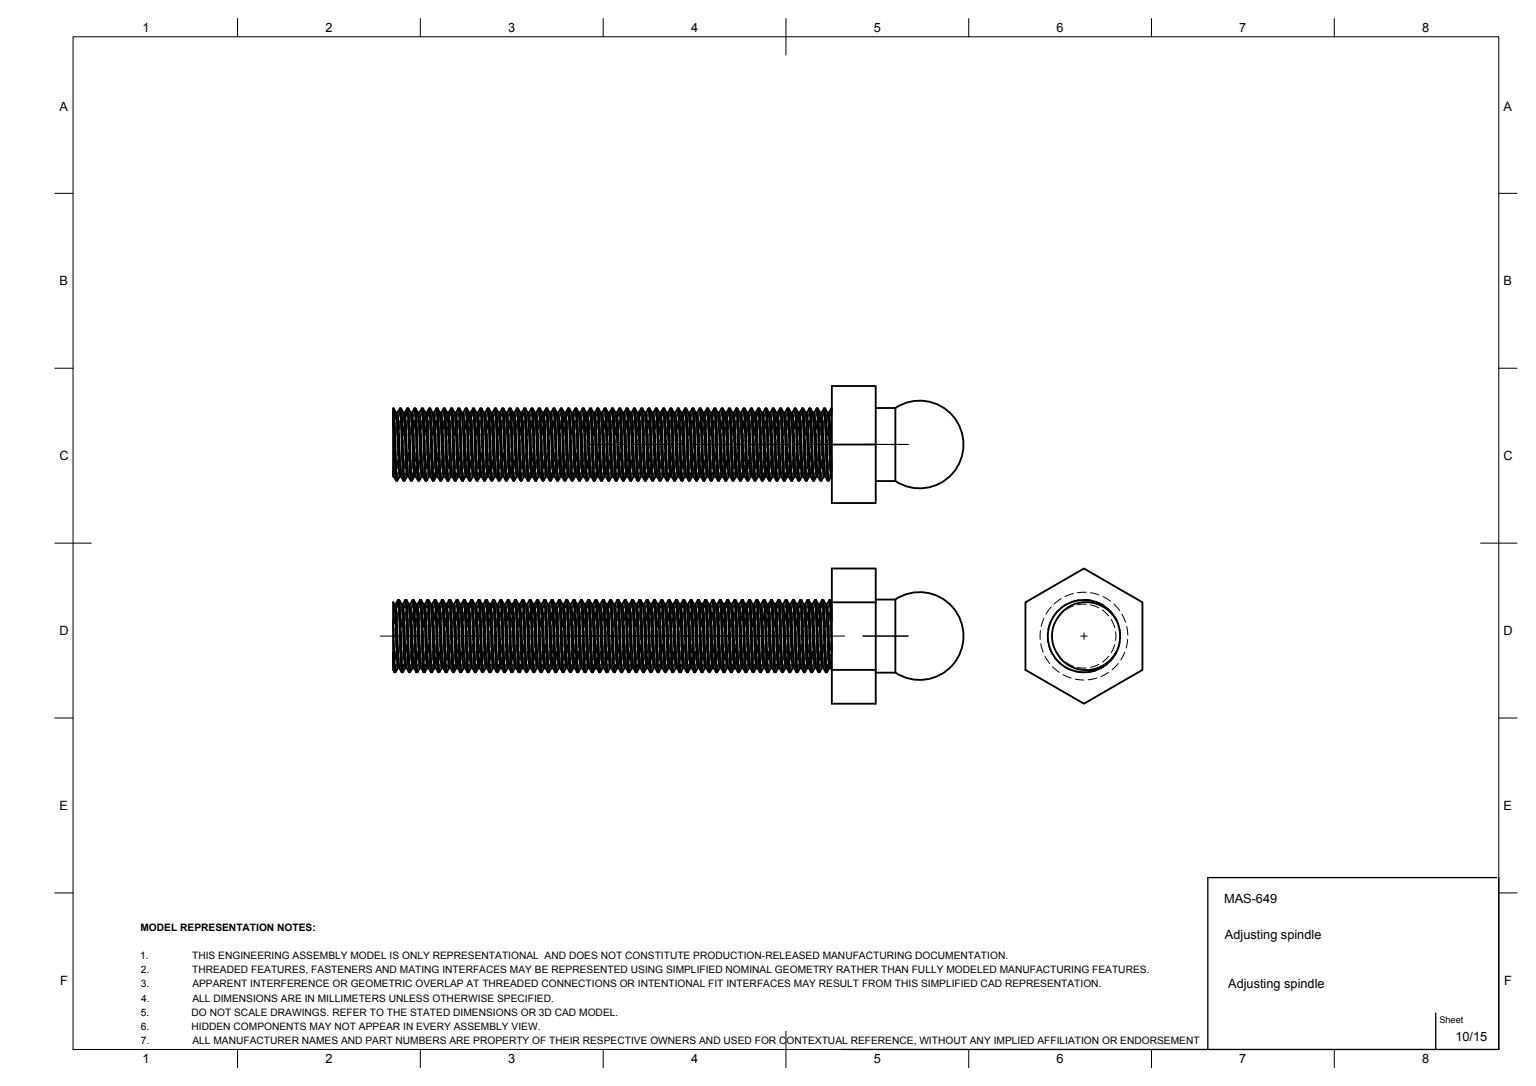
ISO-10303-21;
HEADER;
/* Generated by software containing ST-Developer
 * from STEP Tools, Inc. (www.steptools.com) 
 */

FILE_DESCRIPTION(
/* description */ ('Independent equipment support assembly with bolted 600 x 500 mm welde
d perimeter frame, four adjustable legs and swivel feet. Nominal overa
ll height 518 mm. No load rating assigned.'),
/* implementation_level */ '2;1');

FILE_NAME(
/* name */ 'Adjusting spindle.step',
/* time_stamp */ '2026-11-07T17:30:39-08:00',
/* author */ (''),
/* organization */ (''),
/* preprocessor_version */ 'ST-DEVELOPER v20.2',
/* originating_system */ 'Autodesk Translation Framework v15.17.0.0',
/* authorisation */ '');

FILE_SCHEMA (('AUTOMOTIVE_DESIGN { 1 0 10303 214 3 1 1 }'));
ENDSEC;

DATA;
#10=MECHANICAL_DESIGN_GEOMETRIC_PRESENTATION_REPRESENTATION('',(#2219),#63755);
#13=SPHERICAL_SURFACE('',#15392,6.);
#279=B_SPLINE_SURFACE_WITH_KNOTS('',3,3,((#55973,#55974,#55975,#55976,#55977,
#55978,#55979,#55980,#55981,#55982,#55983,#55984,#55985,#55986,#55987,#55988,
#55989,#55990,#55991,#55992,#55993,#55994,#55995,#55996,#55997,#55998,#55999,
#56000,#56001,#56002,#56003,#56004,#56005,#56006,#56007,#56008,#56009,#56010,
#56011,#56012,#56013,#56014,#56015,#56016,#56017,#56018,#56019,#56020,#56021,
#56022,#56023,#56024,#56025,#56026,#56027,#56028,#56029,#56030,#56031,#56032,
#56033,#56034,#56035,#56036,#56037,#56038,#56039,#56040,#56041,#56042,#56043,
#56044,#56045,#56046,#56047,#56048,#56049,#56050,#56051,#56052,#56053,#56054,
#56055,#56056,#56057,#56058,#56059,#56060,#56061,#56062,#56063,#56064,#56065,
#56066,#56067,#56068,#56069,#56070,#56071,#56072,#56073,#56074,#56075,#56076,
#56077,#56078,#56079,#56080,#56081,#56082,#56083,#56084,#56085,#56086,#56087,
#56088,#56089,#56090,#56091,#56092,#56093,#56094,#56095,#56096,#56097,#56098,
#56099,#56100,#56101,#56102,#56103,#56104,#56105,#56106,#56107,#56108,#56109,
#56110,#56111,#56112,#56113,#56114,#56115,#56116,#56117,#56118,#56119,#56120,
#56121,#56122,#56123,#56124,#56125,#56126,#56127,#56128,#56129,#56130,#56131,
#56132,#56133,#56134,#56135,#56136,#56137,#56138,#56139,#56140,#56141,#56142,
#56143,#56144,#56145,#56146,#56147,#56148,#56149,#56150,#56151,#56152,#56153,
#56154,#56155,#56156,#56157,#56158,#56159,#56160,#56161,#56162,#56163,#56164,
#56165,#56166,#56167,#56168,#56169,#56170,#56171,#56172,#56173,#56174,#56175,
#56176,#56177,#56178,#56179,#56180,#56181,#56182,#56183,#56184,#56185,#56186,
#56187,#56188,#56189,#56190,#56191,#56192,#56193,#56194,#56195,#56196,#56197,
#56198,#56199,#56200,#56201,#56202,#56203,#56204,#56205,#56206,#56207,#56208,
#56209,#56210,#56211,#56212,#56213,#56214,#56215,#56216,#56217,#56218,#56219,
#56220,#56221,#56222,#56223,#56224,#56225,#56226,#56227,#56228,#56229,#56230,
#56231,#56232,#56233,#56234,#56235,#56236,#56237,#56238,#56239,#56240,#56241,
#56242,#56243,#56244,#56245,#56246,#56247,#56248,#56249,#56250,#56251,#56252,
#56253,#56254,#56255,#56256,#56257,#56258,#56259,#56260,#56261,#56262,#56263,
#56264,#56265,#56266,#56267,#56268,#56269,#56270,#56271,#56272,#56273,#56274,
#56275,#56276,#56277,#56278,#56279,#56280,#56281,#56282,#56283,#56284,#56285,
#56286,#56287,#56288,#56289,#56290,#56291,#56292,#56293,#56294,#56295,#56296,
#56297,#56298,#56299,#56300,#56301,#56302,#56303,#56304,#56305,#56306,#56307,
#56308,#56309,#56310,#56311,#56312,#56313,#56314,#56315,#56316,#56317,#56318,
#56319,#56320,#56321,#56322,#56323,#56324,#56325,#56326,#56327,#56328,#56329,
#56330,#56331,#56332,#56333,#56334,#56335,#56336,#56337,#56338,#56339,#56340,
#56341,#56342,#56343,#56344,#56345,#56346,#56347,#56348,#56349,#56350,#56351,
#56352,#56353,#56354,#56355,#56356,#56357),(#56358,#56359,#56360,#56361,
#56362,#56363,#56364,#56365,#56366,#56367,#56368,#56369,#56370,#56371,#56372,
#56373,#56374,#56375,#56376,#56377,#56378,#56379,#56380,#56381,#56382,#56383,
#56384,#56385,#56386,#56387,#56388,#56389,#56390,#56391,#56392,#56393,#56394,
#56395,#56396,#56397,#56398,#56399,#56400,#56401,#56402,#56403,#56404,#56405,
#56406,#56407,#56408,#56409,#56410,#56411,#56412,#56413,#56414,#56415,#56416,
#56417,#56418,#56419,#56420,#56421,#56422,#56423,#56424,#56425,#56426,#56427,
#56428,#56429,#56430,#56431,#56432,#56433,#56434,#56435,#56436,#56437,#56438,
#56439,#56440,#56441,#56442,#56443,#56444,#56445,#56446,#56447,#56448,#56449,
#56450,#56451,#56452,#56453,#56454,#56455,#56456,#56457,#56458,#56459,#56460,
#56461,#56462,#56463,#56464,#56465,#56466,#56467,#56468,#56469,#56470,#56471,
#56472,#56473,#56474,#56475,#56476,#56477,#56478,#56479,#56480,#56481,#56482,
#56483,#56484,#56485,#56486,#56487,#56488,#56489,#56490,#56491,#56492,#56493,
#56494,#56495,#56496,#56497,#56498,#56499,#56500,#56501,#56502,#56503,#56504,
#56505,#56506,#56507,#56508,#56509,#56510,#56511,#56512,#56513,#56514,#56515,
#56516,#56517,#56518,#56519,#56520,#56521,#56522,#56523,#56524,#56525,#56526,
#56527,#56528,#56529,#56530,#56531,#56532,#56533,#56534,#56535,#56536,#56537,
#56538,#56539,#56540,#56541,#56542,#56543,#56544,#56545,#56546,#56547,#56548,
#56549,#56550,#56551,#56552,#56553,#56554,#56555,#56556,#56557,#56558,#56559,
#56560,#56561,#56562,#56563,#56564,#56565,#56566,#56567,#56568,#56569,#56570,
#56571,#56572,#56573,#56574,#56575,#56576,#56577,#56578,#56579,#56580,#56581,
#56582,#56583,#56584,#56585,#56586,#56587,#56588,#56589,#56590,#56591,#56592,
#56593,#56594,#56595,#56596,#56597,#56598,#56599,#56600,#56601,#56602,#56603,
#56604,#56605,#56606,#56607,#56608,#56609,#56610,#56611,#56612,#56613,#56614,
#56615,#56616,#56617,#56618,#56619,#56620,#56621,#56622,#56623,#56624,#56625,
#56626,#56627,#56628,#56629,#56630,#56631,#56632,#56633,#56634,#56635,#56636,
#56637,#56638,#56639,#56640,#56641,#56642,#56643,#56644,#56645,#56646,#56647,
#56648,#56649,#56650,#56651,#56652,#56653,#56654,#56655,#56656,#56657,#56658,
#56659,#56660,#56661,#56662,#56663,#56664,#56665,#56666,#56667,#56668,#56669,
#56670,#56671,#56672,#56673,#56674,#56675,#56676,#56677,#56678,#56679,#56680,
#56681,#56682,#56683,#56684,#56685,#56686,#56687,#56688,#56689,#56690,#56691,
#56692,#56693,#56694,#56695,#56696,#56697,#56698,#56699,#56700,#56701,#56702,
#56703,#56704,#56705,#56706,#56707,#56708,#56709,#56710,#56711,#56712,#56713,
#56714,#56715,#56716,#56717,#56718,#56719,#56720,#56721,#56722,#56723,#56724,
#56725,#56726,#56727,#56728,#56729,#56730,#56731,#56732,#56733,#56734,#56735,
#56736,#56737,#56738,#56739,#56740,#56741,#56742),(#56743,#56744,#56745,
#56746,#56747,#56748,#56749,#56750,#56751,#56752,#56753,#56754,#56755,#56756,
#56757,#56758,#56759,#56760,#56761,#56762,#56763,#56764,#56765,#56766,#56767,
#56768,#56769,#56770,#56771,#56772,#56773,#56774,#56775,#56776,#56777,#56778,
#56779,#56780,#56781,#56782,#56783,#56784,#56785,#56786,#56787,#56788,#56789,
#56790,#56791,#56792,#56793,#56794,#56795,#56796,#56797,#56798,#56799,#56800,
#56801,#56802,#56803,#56804,#56805,#56806,#56807,#56808,#56809,#56810,#56811,
#56812,#56813,#56814,#56815,#56816,#56817,#56818,#56819,#56820,#56821,#56822,
#56823,#56824,#56825,#56826,#56827,#56828,#56829,#56830,#56831,#56832,#56833,
#56834,#56835,#56836,#56837,#56838,#56839,#56840,#56841,#56842,#56843,#56844,
#56845,#56846,#56847,#56848,#56849,#56850,#56851,#56852,#56853,#56854,#56855,
#56856,#56857,#56858,#56859,#56860,#56861,#56862,#56863,#56864,#56865,#56866,
#56867,#56868,#56869,#56870,#56871,#56872,#56873,#56874,#56875,#56876,#56877,
#56878,#56879,#56880,#56881,#56882,#56883,#56884,#56885,#56886,#56887,#56888,
#56889,#56890,#56891,#56892,#56893,#56894,#56895,#56896,#56897,#56898,#56899,
#56900,#56901,#56902,#56903,#56904,#56905,#56906,#56907,#56908,#56909,#56910,
#56911,#56912,#56913,#56914,#56915,#56916,#56917,#56918,#56919,#56920,#56921,
#56922,#56923,#56924,#56925,#56926,#56927,#56928,#56929,#56930,#56931,#56932,
#56933,#56934,#56935,#56936,#56937,#56938,#56939,#56940,#56941,#56942,#56943,
#56944,#56945,#56946,#56947,#56948,#56949,#56950,#56951,#56952,#56953,#56954,
#56955,#56956,#56957,#56958,#56959,#56960,#56961,#56962,#56963,#56964,#56965,
#56966,#56967,#56968,#56969,#56970,#56971,#56972,#56973,#56974,#56975,#56976,
#56977,#56978,#56979,#56980,#56981,#56982,#56983,#56984,#56985,#56986,#56987,
#56988,#56989,#56990,#56991,#56992,#56993,#56994,#56995,#56996,#56997,#56998,
#56999,#57000,#57001,#57002,#57003,#57004,#57005,#57006,#57007,#57008,#57009,
#57010,#57011,#57012,#57013,#57014,#57015,#57016,#57017,#57018,#57019,#57020,
#57021,#57022,#57023,#57024,#57025,#57026,#57027,#57028,#57029,#57030,#57031,
#57032,#57033,#57034,#57035,#57036,#57037,#57038,#57039,#57040,#57041,#57042,
#57043,#57044,#57045,#57046,#57047,#57048,#57049,#57050,#57051,#57052,#57053,
#57054,#57055,#57056,#57057,#57058,#57059,#57060,#57061,#57062,#57063,#57064,
#57065,#57066,#57067,#57068,#57069,#57070,#57071,#57072,#57073,#57074,#57075,
#57076,#57077,#57078,#57079,#57080,#57081,#57082,#57083,#57084,#57085,#57086,
#57087,#57088,#57089,#57090,#57091,#57092,#57093,#57094,#57095,#57096,#57097,
#57098,#57099,#57100,#57101,#57102,#57103,#57104,#57105,#57106,#57107,#57108,
#57109,#57110,#57111,#57112,#57113,#57114,#57115,#57116,#57117,#57118,#57119,
#57120,#57121,#57122,#57123,#57124,#57125,#57126,#57127),(#57128,#57129,
#57130,#57131,#57132,#57133,#57134,#57135,#57136,#57137,#57138,#57139,#57140,
#57141,#57142,#57143,#57144,#57145,#57146,#57147,#57148,#57149,#57150,#57151,
#57152,#57153,#57154,#57155,#57156,#57157,#57158,#57159,#57160,#57161,#57162,
#57163,#57164,#57165,#57166,#57167,#57168,#57169,#57170,#57171,#57172,#57173,
#57174,#57175,#57176,#57177,#57178,#57179,#57180,#57181,#57182,#57183,#57184,
#57185,#57186,#57187,#57188,#57189,#57190,#57191,#57192,#57193,#57194,#57195,
#57196,#57197,#57198,#57199,#57200,#57201,#57202,#57203,#57204,#57205,#57206,
#57207,#57208,#57209,#57210,#57211,#57212,#57213,#57214,#57215,#57216,#57217,
#57218,#57219,#57220,#57221,#57222,#57223,#57224,#57225,#57226,#57227,#57228,
#57229,#57230,#57231,#57232,#57233,#57234,#57235,#57236,#57237,#57238,#57239,
#57240,#57241,#57242,#57243,#57244,#57245,#57246,#57247,#57248,#57249,#57250,
#57251,#57252,#57253,#57254,#57255,#57256,#57257,#57258,#57259,#57260,#57261,
#57262,#57263,#57264,#57265,#57266,#57267,#57268,#57269,#57270,#57271,#57272,
#57273,#57274,#57275,#57276,#57277,#57278,#57279,#57280,#57281,#57282,#57283,
#57284,#57285,#57286,#57287,#57288,#57289,#57290,#57291,#57292,#57293,#57294,
#57295,#57296,#57297,#57298,#57299,#57300,#57301,#57302,#57303,#57304,#57305,
#57306,#57307,#57308,#57309,#57310,#57311,#57312,#57313,#57314,#57315,#57316,
#57317,#57318,#57319,#57320,#57321,#57322,#57323,#57324,#57325,#57326,#57327,
#57328,#57329,#57330,#57331,#57332,#57333,#57334,#57335,#57336,#57337,#57338,
#57339,#57340,#57341,#57342,#57343,#57344,#57345,#57346,#57347,#57348,#57349,
#57350,#57351,#57352,#57353,#57354,#57355,#57356,#57357,#57358,#57359,#57360,
#57361,#57362,#57363,#57364,#57365,#57366,#57367,#57368,#57369,#57370,#57371,
#57372,#57373,#57374,#57375,#57376,#57377,#57378,#57379,#57380,#57381,#57382,
#57383,#57384,#57385,#57386,#57387,#57388,#57389,#57390,#57391,#57392,#57393,
#57394,#57395,#57396,#57397,#57398,#57399,#57400,#57401,#57402,#57403,#57404,
#57405,#57406,#57407,#57408,#57409,#57410,#57411,#57412,#57413,#57414,#57415,
#57416,#57417,#57418,#57419,#57420,#57421,#57422,#57423,#57424,#57425,#57426,
#57427,#57428,#57429,#57430,#57431,#57432,#57433,#57434,#57435,#57436,#57437,
#57438,#57439,#57440,#57441,#57442,#57443,#57444,#57445,#57446,#57447,#57448,
#57449,#57450,#57451,#57452,#57453,#57454,#57455,#57456,#57457,#57458,#57459,
#57460,#57461,#57462,#57463,#57464,#57465,#57466,#57467,#57468,#57469,#57470,
#57471,#57472,#57473,#57474,#57475,#57476,#57477,#57478,#57479,#57480,#57481,
#57482,#57483,#57484,#57485,#57486,#57487,#57488,#57489,#57490,#57491,#57492,
#57493,#57494,#57495,#57496,#57497,#57498,#57499,#57500,#57501,#57502,#57503,
#57504,#57505,#57506,#57507,#57508,#57509,#57510,#57511,#57512)),
 .UNSPECIFIED.,.F.,.F.,.F.,(4,4),(4,1,1,1,1,1,1,1,1,1,1,1,1,1,1,1,1,1,1,
1,1,1,1,1,1,1,1,1,1,1,1,1,1,1,1,1,1,1,1,1,1,1,1,1,1,1,1,1,1,1,1,1,1,1,1,
1,1,1,1,1,1,1,1,1,1,1,1,1,1,1,1,1,1,1,1,1,1,1,1,1,1,1,1,1,1,1,1,1,1,1,1,
1,1,1,1,1,1,1,1,1,1,1,1,1,1,1,1,1,1,1,1,1,1,1,1,1,1,1,1,1,1,1,1,1,1,1,1,
1,1,1,1,1,1,1,1,1,1,1,1,1,1,1,1,1,1,1,1,1,1,1,1,1,1,1,1,1,1,1,1,1,1,1,1,
1,1,1,1,1,1,1,1,1,1,1,1,1,1,1,1,1,1,1,1,1,1,1,1,1,1,1,1,1,1,1,1,1,1,1,1,
1,1,1,1,1,1,1,1,1,1,1,1,1,1,1,1,1,1,1,1,1,1,1,1,1,1,1,1,1,1,1,1,1,1,1,1,
1,1,1,1,1,1,1,1,1,1,1,1,1,1,1,1,1,1,1,1,1,1,1,1,1,1,1,1,1,1,1,1,1,1,1,1,
1,1,1,1,1,1,1,1,1,1,1,1,1,1,1,1,1,1,1,1,1,1,1,1,1,1,1,1,1,1,1,1,1,1,1,1,
1,1,1,1,1,1,1,1,1,1,1,1,1,1,1,1,1,1,1,1,1,1,1,1,1,1,1,1,1,1,1,1,1,1,1,1,
1,1,1,1,1,1,1,1,1,1,1,1,1,1,1,1,1,1,1,1,1,1,1,1,1,1,1,1,1,1,1,1,1,1,1,1,
1,1,1,4),(0.,0.0658179306876174),(8.30838445208392,8.80714609643392,9.30590774078392,
10.3034310294839,11.3009543181839,12.2984776068839,13.2960008955839,14.2935241842839,
15.291047472984,16.288570761684,17.286094050384,18.283617339084,19.281140627784,
20.278663916484,21.276187205184,22.273710493884,23.271233782584,24.268757071284,
25.266280359984,26.263803648684,27.261326937384,28.258850226084,29.256373514784,
30.253896803484,31.251420092184,32.2489433808841,33.2464666695841,34.2439899582841,
35.2415132469841,36.2390365356841,37.2365598243841,38.2340831130841,39.2316064017841,
40.2291296904841,41.2266529791841,42.2241762678841,43.2216995565841,44.2192228452841,
45.2167461339841,46.2142694226841,47.2117927113841,48.2093160000841,49.2068392887841,
50.2043625774841,51.2018858661842,52.1994091548842,53.1969324435842,54.1944557322842,
55.1919790209842,56.1895023096842,57.1870255983842,58.1845488870842,59.1820721757842,
60.1795954644842,61.1771187531842,62.1746420418842,63.1721653305842,64.1696886192842,
65.1672119079842,66.1647351966842,67.1622584853842,68.1597817740843,69.1573050627842,
70.1548283514843,71.1523516401843,72.1498749288843,73.1473982175843,74.1449215062843,
75.1424447949843,76.1399680836843,77.1374913723843,78.1350146610843,79.1325379497843,
80.1300612384843,81.1275845271843,82.1251078158843,83.1226311045843,84.1201543932843,
85.1176776819843,86.1152009706843,87.1127242593844,88.1102475480844,89.1077708367844,
90.1052941254844,91.1028174141844,92.1003407028844,93.0978639915844,94.0953872802844,
95.0929105689844,96.0904338576844,97.0879571463844,98.0854804350844,99.0830037237844,
100.080527012484,101.078050301184,102.075573589884,103.073096878584,104.070620167284,
105.068143455984,106.065666744684,107.063190033384,108.060713322084,109.058236610784,
110.055759899484,111.053283188184,112.050806476884,113.048329765584,114.045853054284,
115.043376342985,116.040899631685,117.038422920385,118.035946209085,119.033469497785,
120.030992786485,121.028516075185,122.026039363885,123.023562652585,124.021085941285,
125.018609229985,126.016132518685,127.013655807385,128.011179096085,129.008702384785,
130.006225673485,131.003748962185,132.001272250885,132.998795539585,133.996318828285,
134.993842116985,135.991365405685,136.988888694385,137.986411983085,138.983935271785,
139.981458560485,140.978981849185,141.976505137885,142.974028426585,143.971551715285,
144.969075003985,145.966598292685,146.964121581385,147.961644870085,148.959168158785,
149.956691447485,150.954214736185,151.951738024885,152.949261313585,153.946784602285,
154.944307890985,155.941831179685,156.939354468385,157.936877757085,158.934401045785,
159.931924334485,160.929447623185,161.926970911885,162.924494200585,163.922017489285,
164.919540777985,165.917064066685,166.914587355385,167.912110644085,168.909633932785,
169.907157221485,170.904680510185,171.902203798885,172.899727087585,173.897250376285,
174.894773664985,175.892296953685,176.889820242385,177.887343531085,178.884866819785,
179.882390108485,180.879913397185,181.877436685885,182.874959974585,183.872483263285,
184.870006551985,185.867529840685,186.865053129385,187.862576418085,188.860099706785,
189.857622995485,190.855146284185,191.852669572885,192.850192861585,193.847716150285,
194.845239438985,195.842762727685,196.840286016385,197.837809305085,198.835332593785,
199.832855882485,200.830379171185,201.827902459885,202.825425748585,203.822949037285,
204.820472325985,205.817995614685,206.815518903385,207.813042192085,208.810565480785,
209.808088769485,210.805612058185,211.803135346885,212.800658635585,213.798181924285,
214.795705212985,215.793228501685,216.790751790385,217.788275079085,218.785798367785,
219.783321656485,220.780844945185,221.778368233885,222.775891522585,223.773414811285,
224.770938099985,225.768461388685,226.765984677385,227.763507966085,228.761031254785,
229.758554543485,230.756077832185,231.753601120885,232.751124409585,233.748647698285,
234.746170986985,235.743694275685,236.741217564385,237.738740853085,238.736264141785,
239.733787430485,240.731310719185,241.728834007885,242.726357296585,243.723880585285,
244.721403873985,245.718927162685,246.716450451385,247.713973740085,248.711497028785,
249.709020317485,250.706543606185,251.704066894885,252.701590183585,253.699113472285,
254.696636760985,255.694160049685,256.691683338385,257.689206627085,258.686729915785,
259.684253204485,260.681776493185,261.679299781885,262.676823070585,263.674346359285,
264.671869647985,265.669392936685,266.666916225385,267.664439514085,268.661962802785,
269.659486091485,270.657009380185,271.654532668885,272.652055957585,273.649579246285,
274.647102534985,275.644625823685,276.642149112385,277.639672401085,278.637195689785,
279.634718978485,280.632242267185,281.629765555885,282.627288844585,283.624812133285,
284.622335421985,285.619858710685,286.617381999385,287.614905288085,288.612428576785,
289.609951865485,290.607475154186,291.604998442886,292.602521731586,293.600045020286,
294.597568308986,295.595091597686,296.592614886386,297.590138175086,298.587661463786,
299.585184752486,300.582708041186,301.580231329886,302.577754618586,303.575277907286,
304.572801195986,305.570324484686,306.567847773386,307.565371062086,308.562894350786,
309.560417639486,310.557940928186,311.555464216886,312.552987505586,313.550510794286,
314.548034082986,315.545557371686,316.543080660386,317.540603949086,318.538127237786,
319.535650526486,320.533173815186,321.530697103886,322.528220392586,323.525743681286,
324.523266969986,325.520790258686,326.518313547386,327.515836836086,328.513360124786,
329.510883413486,330.508406702186,331.505929990886,332.503453279586,333.500976568286,
334.498499856986,335.496023145686,336.493546434386,337.491069723086,338.488593011786,
339.486116300486,340.483639589186,341.481162877886,342.478686166586,343.476209455286,
344.473732743986,345.471256032686,346.468779321386,347.466302610086,348.463825898786,
349.461349187486,350.458872476186,351.456395764886,352.453919053586,353.451442342286,
354.448965630986,355.446488919686,356.444012208386,357.441535497086,358.439058785786,
359.436582074486,360.434105363186,361.431628651886,362.429151940586,363.426675229286,
364.424198517986,365.421721806686,366.419245095386,367.416768384086,368.414291672786,
369.411814961486,370.409338250186,371.406861538886,372.404384827586,373.401908116286,
374.399431404986,375.396954693686,376.394477982386,377.392001271086,378.389524559786,
379.387047848486,380.384571137186,381.382094425886,382.379617714586,383.377141003286,
384.374664291986,385.372187580686,386.369710869386,386.868472513736,387.367234158086),
 .UNSPECIFIED.);
#280=B_SPLINE_SURFACE_WITH_KNOTS('',3,3,((#57770,#57771,#57772,#57773,#57774,
#57775,#57776,#57777,#57778,#57779,#57780,#57781,#57782,#57783,#57784,#57785,
#57786,#57787,#57788,#57789,#57790,#57791,#57792,#57793,#57794,#57795,#57796,
#57797,#57798,#57799,#57800,#57801,#57802,#57803,#57804,#57805,#57806,#57807,
#57808,#57809,#57810,#57811,#57812,#57813,#57814,#57815,#57816,#57817,#57818,
#57819,#57820,#57821,#57822,#57823,#57824,#57825,#57826,#57827,#57828,#57829,
#57830,#57831,#57832,#57833,#57834,#57835,#57836,#57837,#57838,#57839,#57840,
#57841,#57842,#57843,#57844,#57845,#57846,#57847,#57848,#57849,#57850,#57851,
#57852,#57853,#57854,#57855,#57856,#57857,#57858,#57859,#57860,#57861,#57862,
#57863,#57864,#57865,#57866,#57867,#57868,#57869,#57870,#57871,#57872,#57873,
#57874,#57875,#57876,#57877,#57878,#57879,#57880,#57881,#57882,#57883,#57884,
#57885,#57886,#57887,#57888,#57889,#57890,#57891,#57892,#57893,#57894,#57895,
#57896,#57897,#57898,#57899,#57900,#57901,#57902,#57903,#57904,#57905,#57906,
#57907,#57908,#57909,#57910,#57911,#57912,#57913,#57914,#57915,#57916,#57917,
#57918,#57919,#57920,#57921,#57922,#57923,#57924,#57925,#57926,#57927,#57928,
#57929,#57930,#57931,#57932,#57933,#57934,#57935,#57936,#57937,#57938,#57939,
#57940,#57941,#57942,#57943,#57944,#57945,#57946,#57947,#57948,#57949,#57950,
#57951,#57952,#57953,#57954,#57955,#57956,#57957,#57958,#57959,#57960,#57961,
#57962,#57963,#57964,#57965,#57966,#57967,#57968,#57969,#57970,#57971,#57972,
#57973,#57974,#57975,#57976,#57977,#57978,#57979,#57980,#57981,#57982,#57983,
#57984,#57985,#57986,#57987,#57988,#57989,#57990,#57991,#57992,#57993,#57994,
#57995,#57996,#57997,#57998,#57999,#58000,#58001,#58002,#58003,#58004,#58005,
#58006,#58007,#58008,#58009,#58010,#58011,#58012,#58013,#58014,#58015,#58016,
#58017,#58018,#58019,#58020,#58021,#58022,#58023,#58024,#58025,#58026,#58027,
#58028,#58029,#58030,#58031,#58032,#58033,#58034,#58035,#58036,#58037,#58038,
#58039,#58040,#58041,#58042,#58043,#58044,#58045,#58046,#58047,#58048,#58049,
#58050,#58051,#58052,#58053,#58054,#58055,#58056,#58057,#58058,#58059,#58060,
#58061,#58062,#58063,#58064,#58065,#58066,#58067,#58068,#58069,#58070,#58071,
#58072,#58073,#58074,#58075,#58076,#58077,#58078,#58079,#58080,#58081,#58082,
#58083,#58084,#58085,#58086,#58087,#58088,#58089,#58090,#58091,#58092,#58093,
#58094,#58095,#58096,#58097,#58098,#58099,#58100,#58101,#58102,#58103,#58104,
#58105,#58106,#58107,#58108,#58109,#58110,#58111,#58112,#58113,#58114,#58115,
#58116,#58117,#58118,#58119,#58120,#58121,#58122,#58123,#58124,#58125,#58126,
#58127,#58128,#58129,#58130,#58131,#58132,#58133,#58134,#58135,#58136,#58137,
#58138,#58139,#58140,#58141,#58142,#58143,#58144,#58145,#58146,#58147,#58148,
#58149,#58150,#58151,#58152,#58153,#58154),(#58155,#58156,#58157,#58158,
#58159,#58160,#58161,#58162,#58163,#58164,#58165,#58166,#58167,#58168,#58169,
#58170,#58171,#58172,#58173,#58174,#58175,#58176,#58177,#58178,#58179,#58180,
#58181,#58182,#58183,#58184,#58185,#58186,#58187,#58188,#58189,#58190,#58191,
#58192,#58193,#58194,#58195,#58196,#58197,#58198,#58199,#58200,#58201,#58202,
#58203,#58204,#58205,#58206,#58207,#58208,#58209,#58210,#58211,#58212,#58213,
#58214,#58215,#58216,#58217,#58218,#58219,#58220,#58221,#58222,#58223,#58224,
#58225,#58226,#58227,#58228,#58229,#58230,#58231,#58232,#58233,#58234,#58235,
#58236,#58237,#58238,#58239,#58240,#58241,#58242,#58243,#58244,#58245,#58246,
#58247,#58248,#58249,#58250,#58251,#58252,#58253,#58254,#58255,#58256,#58257,
#58258,#58259,#58260,#58261,#58262,#58263,#58264,#58265,#58266,#58267,#58268,
#58269,#58270,#58271,#58272,#58273,#58274,#58275,#58276,#58277,#58278,#58279,
#58280,#58281,#58282,#58283,#58284,#58285,#58286,#58287,#58288,#58289,#58290,
#58291,#58292,#58293,#58294,#58295,#58296,#58297,#58298,#58299,#58300,#58301,
#58302,#58303,#58304,#58305,#58306,#58307,#58308,#58309,#58310,#58311,#58312,
#58313,#58314,#58315,#58316,#58317,#58318,#58319,#58320,#58321,#58322,#58323,
#58324,#58325,#58326,#58327,#58328,#58329,#58330,#58331,#58332,#58333,#58334,
#58335,#58336,#58337,#58338,#58339,#58340,#58341,#58342,#58343,#58344,#58345,
#58346,#58347,#58348,#58349,#58350,#58351,#58352,#58353,#58354,#58355,#58356,
#58357,#58358,#58359,#58360,#58361,#58362,#58363,#58364,#58365,#58366,#58367,
#58368,#58369,#58370,#58371,#58372,#58373,#58374,#58375,#58376,#58377,#58378,
#58379,#58380,#58381,#58382,#58383,#58384,#58385,#58386,#58387,#58388,#58389,
#58390,#58391,#58392,#58393,#58394,#58395,#58396,#58397,#58398,#58399,#58400,
#58401,#58402,#58403,#58404,#58405,#58406,#58407,#58408,#58409,#58410,#58411,
#58412,#58413,#58414,#58415,#58416,#58417,#58418,#58419,#58420,#58421,#58422,
#58423,#58424,#58425,#58426,#58427,#58428,#58429,#58430,#58431,#58432,#58433,
#58434,#58435,#58436,#58437,#58438,#58439,#58440,#58441,#58442,#58443,#58444,
#58445,#58446,#58447,#58448,#58449,#58450,#58451,#58452,#58453,#58454,#58455,
#58456,#58457,#58458,#58459,#58460,#58461,#58462,#58463,#58464,#58465,#58466,
#58467,#58468,#58469,#58470,#58471,#58472,#58473,#58474,#58475,#58476,#58477,
#58478,#58479,#58480,#58481,#58482,#58483,#58484,#58485,#58486,#58487,#58488,
#58489,#58490,#58491,#58492,#58493,#58494,#58495,#58496,#58497,#58498,#58499,
#58500,#58501,#58502,#58503,#58504,#58505,#58506,#58507,#58508,#58509,#58510,
#58511,#58512,#58513,#58514,#58515,#58516,#58517,#58518,#58519,#58520,#58521,
#58522,#58523,#58524,#58525,#58526,#58527,#58528,#58529,#58530,#58531,#58532,
#58533,#58534,#58535,#58536,#58537,#58538,#58539),(#58540,#58541,#58542,
#58543,#58544,#58545,#58546,#58547,#58548,#58549,#58550,#58551,#58552,#58553,
#58554,#58555,#58556,#58557,#58558,#58559,#58560,#58561,#58562,#58563,#58564,
#58565,#58566,#58567,#58568,#58569,#58570,#58571,#58572,#58573,#58574,#58575,
#58576,#58577,#58578,#58579,#58580,#58581,#58582,#58583,#58584,#58585,#58586,
#58587,#58588,#58589,#58590,#58591,#58592,#58593,#58594,#58595,#58596,#58597,
#58598,#58599,#58600,#58601,#58602,#58603,#58604,#58605,#58606,#58607,#58608,
#58609,#58610,#58611,#58612,#58613,#58614,#58615,#58616,#58617,#58618,#58619,
#58620,#58621,#58622,#58623,#58624,#58625,#58626,#58627,#58628,#58629,#58630,
#58631,#58632,#58633,#58634,#58635,#58636,#58637,#58638,#58639,#58640,#58641,
#58642,#58643,#58644,#58645,#58646,#58647,#58648,#58649,#58650,#58651,#58652,
#58653,#58654,#58655,#58656,#58657,#58658,#58659,#58660,#58661,#58662,#58663,
#58664,#58665,#58666,#58667,#58668,#58669,#58670,#58671,#58672,#58673,#58674,
#58675,#58676,#58677,#58678,#58679,#58680,#58681,#58682,#58683,#58684,#58685,
#58686,#58687,#58688,#58689,#58690,#58691,#58692,#58693,#58694,#58695,#58696,
#58697,#58698,#58699,#58700,#58701,#58702,#58703,#58704,#58705,#58706,#58707,
#58708,#58709,#58710,#58711,#58712,#58713,#58714,#58715,#58716,#58717,#58718,
#58719,#58720,#58721,#58722,#58723,#58724,#58725,#58726,#58727,#58728,#58729,
#58730,#58731,#58732,#58733,#58734,#58735,#58736,#58737,#58738,#58739,#58740,
#58741,#58742,#58743,#58744,#58745,#58746,#58747,#58748,#58749,#58750,#58751,
#58752,#58753,#58754,#58755,#58756,#58757,#58758,#58759,#58760,#58761,#58762,
#58763,#58764,#58765,#58766,#58767,#58768,#58769,#58770,#58771,#58772,#58773,
#58774,#58775,#58776,#58777,#58778,#58779,#58780,#58781,#58782,#58783,#58784,
#58785,#58786,#58787,#58788,#58789,#58790,#58791,#58792,#58793,#58794,#58795,
#58796,#58797,#58798,#58799,#58800,#58801,#58802,#58803,#58804,#58805,#58806,
#58807,#58808,#58809,#58810,#58811,#58812,#58813,#58814,#58815,#58816,#58817,
#58818,#58819,#58820,#58821,#58822,#58823,#58824,#58825,#58826,#58827,#58828,
#58829,#58830,#58831,#58832,#58833,#58834,#58835,#58836,#58837,#58838,#58839,
#58840,#58841,#58842,#58843,#58844,#58845,#58846,#58847,#58848,#58849,#58850,
#58851,#58852,#58853,#58854,#58855,#58856,#58857,#58858,#58859,#58860,#58861,
#58862,#58863,#58864,#58865,#58866,#58867,#58868,#58869,#58870,#58871,#58872,
#58873,#58874,#58875,#58876,#58877,#58878,#58879,#58880,#58881,#58882,#58883,
#58884,#58885,#58886,#58887,#58888,#58889,#58890,#58891,#58892,#58893,#58894,
#58895,#58896,#58897,#58898,#58899,#58900,#58901,#58902,#58903,#58904,#58905,
#58906,#58907,#58908,#58909,#58910,#58911,#58912,#58913,#58914,#58915,#58916,
#58917,#58918,#58919,#58920,#58921,#58922,#58923,#58924),(#58925,#58926,
#58927,#58928,#58929,#58930,#58931,#58932,#58933,#58934,#58935,#58936,#58937,
#58938,#58939,#58940,#58941,#58942,#58943,#58944,#58945,#58946,#58947,#58948,
#58949,#58950,#58951,#58952,#58953,#58954,#58955,#58956,#58957,#58958,#58959,
#58960,#58961,#58962,#58963,#58964,#58965,#58966,#58967,#58968,#58969,#58970,
#58971,#58972,#58973,#58974,#58975,#58976,#58977,#58978,#58979,#58980,#58981,
#58982,#58983,#58984,#58985,#58986,#58987,#58988,#58989,#58990,#58991,#58992,
#58993,#58994,#58995,#58996,#58997,#58998,#58999,#59000,#59001,#59002,#59003,
#59004,#59005,#59006,#59007,#59008,#59009,#59010,#59011,#59012,#59013,#59014,
#59015,#59016,#59017,#59018,#59019,#59020,#59021,#59022,#59023,#59024,#59025,
#59026,#59027,#59028,#59029,#59030,#59031,#59032,#59033,#59034,#59035,#59036,
#59037,#59038,#59039,#59040,#59041,#59042,#59043,#59044,#59045,#59046,#59047,
#59048,#59049,#59050,#59051,#59052,#59053,#59054,#59055,#59056,#59057,#59058,
#59059,#59060,#59061,#59062,#59063,#59064,#59065,#59066,#59067,#59068,#59069,
#59070,#59071,#59072,#59073,#59074,#59075,#59076,#59077,#59078,#59079,#59080,
#59081,#59082,#59083,#59084,#59085,#59086,#59087,#59088,#59089,#59090,#59091,
#59092,#59093,#59094,#59095,#59096,#59097,#59098,#59099,#59100,#59101,#59102,
#59103,#59104,#59105,#59106,#59107,#59108,#59109,#59110,#59111,#59112,#59113,
#59114,#59115,#59116,#59117,#59118,#59119,#59120,#59121,#59122,#59123,#59124,
#59125,#59126,#59127,#59128,#59129,#59130,#59131,#59132,#59133,#59134,#59135,
#59136,#59137,#59138,#59139,#59140,#59141,#59142,#59143,#59144,#59145,#59146,
#59147,#59148,#59149,#59150,#59151,#59152,#59153,#59154,#59155,#59156,#59157,
#59158,#59159,#59160,#59161,#59162,#59163,#59164,#59165,#59166,#59167,#59168,
#59169,#59170,#59171,#59172,#59173,#59174,#59175,#59176,#59177,#59178,#59179,
#59180,#59181,#59182,#59183,#59184,#59185,#59186,#59187,#59188,#59189,#59190,
#59191,#59192,#59193,#59194,#59195,#59196,#59197,#59198,#59199,#59200,#59201,
#59202,#59203,#59204,#59205,#59206,#59207,#59208,#59209,#59210,#59211,#59212,
#59213,#59214,#59215,#59216,#59217,#59218,#59219,#59220,#59221,#59222,#59223,
#59224,#59225,#59226,#59227,#59228,#59229,#59230,#59231,#59232,#59233,#59234,
#59235,#59236,#59237,#59238,#59239,#59240,#59241,#59242,#59243,#59244,#59245,
#59246,#59247,#59248,#59249,#59250,#59251,#59252,#59253,#59254,#59255,#59256,
#59257,#59258,#59259,#59260,#59261,#59262,#59263,#59264,#59265,#59266,#59267,
#59268,#59269,#59270,#59271,#59272,#59273,#59274,#59275,#59276,#59277,#59278,
#59279,#59280,#59281,#59282,#59283,#59284,#59285,#59286,#59287,#59288,#59289,
#59290,#59291,#59292,#59293,#59294,#59295,#59296,#59297,#59298,#59299,#59300,
#59301,#59302,#59303,#59304,#59305,#59306,#59307,#59308,#59309)),
 .UNSPECIFIED.,.F.,.F.,.F.,(4,4),(4,1,1,1,1,1,1,1,1,1,1,1,1,1,1,1,1,1,1,
1,1,1,1,1,1,1,1,1,1,1,1,1,1,1,1,1,1,1,1,1,1,1,1,1,1,1,1,1,1,1,1,1,1,1,1,
1,1,1,1,1,1,1,1,1,1,1,1,1,1,1,1,1,1,1,1,1,1,1,1,1,1,1,1,1,1,1,1,1,1,1,1,
1,1,1,1,1,1,1,1,1,1,1,1,1,1,1,1,1,1,1,1,1,1,1,1,1,1,1,1,1,1,1,1,1,1,1,1,
1,1,1,1,1,1,1,1,1,1,1,1,1,1,1,1,1,1,1,1,1,1,1,1,1,1,1,1,1,1,1,1,1,1,1,1,
1,1,1,1,1,1,1,1,1,1,1,1,1,1,1,1,1,1,1,1,1,1,1,1,1,1,1,1,1,1,1,1,1,1,1,1,
1,1,1,1,1,1,1,1,1,1,1,1,1,1,1,1,1,1,1,1,1,1,1,1,1,1,1,1,1,1,1,1,1,1,1,1,
1,1,1,1,1,1,1,1,1,1,1,1,1,1,1,1,1,1,1,1,1,1,1,1,1,1,1,1,1,1,1,1,1,1,1,1,
1,1,1,1,1,1,1,1,1,1,1,1,1,1,1,1,1,1,1,1,1,1,1,1,1,1,1,1,1,1,1,1,1,1,1,1,
1,1,1,1,1,1,1,1,1,1,1,1,1,1,1,1,1,1,1,1,1,1,1,1,1,1,1,1,1,1,1,1,1,1,1,1,
1,1,1,1,1,1,1,1,1,1,1,1,1,1,1,1,1,1,1,1,1,1,1,1,1,1,1,1,1,1,1,1,1,1,1,1,
1,1,1,4),(0.,0.0658179306876174),(11.6150328478191,12.1137944921691,12.6125561365191,
13.6100794252191,14.6076027139191,15.6051260026191,16.6026492913191,17.6001725800191,
18.5976958687191,19.5952191574192,20.5927424461192,21.5902657348192,22.5877890235192,
23.5853123122192,24.5828356009192,25.5803588896192,26.5778821783192,27.5754054670192,
28.5729287557192,29.5704520444192,30.5679753331192,31.5654986218192,32.5630219105192,
33.5605451992192,34.5580684879192,35.5555917766192,36.5531150653192,37.5506383540192,
38.5481616427193,39.5456849314193,40.5432082201193,41.5407315088193,42.5382547975193,
43.5357780862193,44.5333013749193,45.5308246636193,46.5283479523193,47.5258712410193,
48.5233945297193,49.5209178184193,50.5184411071193,51.5159643958193,52.5134876845193,
53.5110109732193,54.5085342619193,55.5060575506193,56.5035808393194,57.5011041280194,
58.4986274167194,59.4961507054194,60.4936739941194,61.4911972828194,62.4887205715194,
63.4862438602194,64.4837671489194,65.4812904376194,66.4788137263194,67.4763370150194,
68.4738603037194,69.4713835924194,70.4689068811194,71.4664301698194,72.4639534585194,
73.4614767472195,74.4590000359194,75.4565233246195,76.4540466133195,77.4515699020195,
78.4490931907195,79.4466164794195,80.4441397681195,81.4416630568195,82.4391863455195,
83.4367096342195,84.4342329229195,85.4317562116195,86.4292795003195,87.4268027890195,
88.4243260777195,89.4218493664195,90.4193726551195,91.4168959438195,92.4144192325195,
93.4119425212196,94.4094658099196,95.4069890986196,96.4045123873196,97.4020356760196,
98.3995589647196,99.3970822534196,100.39460554212,101.39212883082,102.38965211952,
103.38717540822,104.38469869692,105.38222198562,106.37974527432,107.37726856302,
108.37479185172,109.37231514042,110.36983842912,111.36736171782,112.36488500652,
113.36240829522,114.35993158392,115.35745487262,116.35497816132,117.35250145002,
118.35002473872,119.34754802742,120.34507131612,121.34259460482,122.34011789352,
123.33764118222,124.33516447092,125.33268775962,126.33021104832,127.32773433702,
128.32525762572,129.32278091442,130.32030420312,131.31782749182,132.31535078052,
133.31287406922,134.31039735792,135.30792064662,136.30544393532,137.30296722402,
138.30049051272,139.29801380142,140.29553709012,141.29306037882,142.29058366752,
143.28810695622,144.28563024492,145.28315353362,146.28067682232,147.27820011102,
148.27572339972,149.27324668842,150.27076997712,151.26829326582,152.26581655452,
153.26333984322,154.26086313192,155.25838642062,156.25590970932,157.25343299802,
158.25095628672,159.24847957542,160.24600286412,161.24352615282,162.24104944152,
163.23857273022,164.23609601892,165.23361930762,166.23114259632,167.22866588502,
168.22618917372,169.22371246242,170.22123575112,171.21875903982,172.21628232852,
173.21380561722,174.21132890592,175.20885219462,176.20637548332,177.20389877202,
178.20142206072,179.19894534942,180.19646863812,181.19399192682,182.19151521552,
183.18903850422,184.18656179292,185.18408508162,186.18160837032,187.17913165902,
188.17665494772,189.17417823642,190.17170152512,191.16922481382,192.16674810252,
193.16427139122,194.16179467992,195.15931796862,196.15684125732,197.15436454602,
198.15188783472,199.14941112342,200.14693441212,201.14445770082,202.14198098952,
203.13950427822,204.13702756692,205.13455085562,206.13207414432,207.12959743302,
208.12712072172,209.12464401042,210.12216729912,211.11969058782,212.11721387652,
213.11473716522,214.11226045392,215.10978374262,216.10730703132,217.10483032002,
218.10235360872,219.09987689742,220.09740018612,221.09492347482,222.09244676352,
223.08997005222,224.08749334092,225.08501662962,226.08253991832,227.08006320702,
228.07758649572,229.07510978442,230.07263307312,231.07015636182,232.06767965052,
233.06520293922,234.06272622792,235.06024951662,236.05777280532,237.05529609402,
238.05281938272,239.05034267142,240.04786596012,241.04538924882,242.04291253752,
243.04043582622,244.03795911492,245.03548240362,246.03300569232,247.03052898102,
248.02805226972,249.02557555842,250.02309884712,251.02062213582,252.01814542452,
253.01566871322,254.01319200192,255.01071529062,256.00823857932,257.00576186802,
258.00328515672,259.00080844542,259.99833173412,260.99585502282,261.99337831152,
262.99090160022,263.98842488892,264.98594817762,265.983471466321,266.980994755021,
267.97851804372,268.97604133242,269.973564621121,270.971087909821,271.968611198521,
272.966134487221,273.963657775921,274.961181064621,275.958704353321,276.956227642021,
277.953750930721,278.951274219421,279.948797508121,280.946320796821,281.943844085521,
282.941367374221,283.938890662921,284.936413951621,285.933937240321,286.931460529021,
287.928983817721,288.926507106421,289.924030395121,290.921553683821,291.919076972521,
292.916600261221,293.914123549921,294.911646838621,295.909170127321,296.906693416021,
297.904216704721,298.901739993421,299.899263282121,300.896786570821,301.894309859521,
302.891833148221,303.889356436921,304.886879725621,305.884403014321,306.881926303021,
307.879449591721,308.876972880421,309.874496169121,310.872019457821,311.869542746521,
312.867066035221,313.864589323921,314.862112612621,315.859635901321,316.857159190021,
317.854682478721,318.852205767421,319.849729056121,320.847252344821,321.844775633521,
322.842298922221,323.839822210921,324.837345499621,325.834868788321,326.832392077021,
327.829915365721,328.827438654421,329.824961943121,330.822485231821,331.820008520521,
332.817531809221,333.815055097921,334.812578386621,335.810101675321,336.807624964021,
337.805148252721,338.802671541421,339.800194830121,340.797718118821,341.795241407521,
342.792764696221,343.790287984921,344.787811273621,345.785334562321,346.782857851021,
347.780381139721,348.777904428421,349.775427717121,350.772951005821,351.770474294521,
352.767997583221,353.765520871921,354.763044160621,355.760567449321,356.758090738021,
357.755614026721,358.753137315421,359.750660604121,360.748183892821,361.745707181521,
362.743230470221,363.740753758921,364.738277047621,365.735800336321,366.733323625021,
367.730846913721,368.728370202421,369.725893491121,370.723416779821,371.720940068521,
372.718463357221,373.715986645921,374.713509934621,375.711033223321,376.708556512021,
377.706079800721,378.703603089421,379.701126378121,380.698649666821,381.696172955521,
382.693696244221,383.691219532921,384.688742821621,385.686266110321,386.683789399021,
387.681312687721,388.678835976421,389.676359265121,390.175120909471,390.673882553821),
 .UNSPECIFIED.);
#461=CIRCLE('',#15255,4.942);
#462=CIRCLE('',#15316,4.372);
#463=CIRCLE('',#15377,4.372);
#464=CIRCLE('',#15379,4.942);
#465=CIRCLE('',#15382,5.);
#466=CIRCLE('',#15390,5.);
#467=CIRCLE('',#15393,6.);
#1233=B_SPLINE_CURVE_WITH_KNOTS('',3,(#51551,#51552,#51553,#51554,#51555,
#51556,#51557,#51558,#51559,#51560),.UNSPECIFIED.,.F.,.F.,(4,3,3,4),(-4.09293042013064,
-3.99009315480002,-2.99256986610002,-2.06773127522702),.UNSPECIFIED.);
#1234=B_SPLINE_CURVE_WITH_KNOTS('',3,(#51563,#51564,#51565,#51566,#51567,
#51568,#51569,#51570,#51571,#51572),.UNSPECIFIED.,.F.,.F.,(4,3,3,4),(0.,
0.49876164434999,0.997523288699981,1.11639350868703),.UNSPECIFIED.);
#1235=B_SPLINE_CURVE_WITH_KNOTS('',3,(#51577,#51578,#51579,#51580,#51581,
#51582,#51583,#51584,#51585,#51586,#51587,#51588,#51589,#51590,#51591,#51592,
#51593,#51594,#51595,#51596,#51597,#51598),.UNSPECIFIED.,.F.,.F.,(4,3,3,
3,3,3,3,4),(-10.3761157273102,-9.97523288700005,-8.97770959830005,-7.98018630960004,
-6.98266302090004,-5.98513973220003,-4.98761644350003,-4.09293042013064),
 .UNSPECIFIED.);
#1236=B_SPLINE_CURVE_WITH_KNOTS('',3,(#51599,#51600,#51601,#51602,#51603,
#51604,#51605,#51606,#51607,#51608,#51609,#51610,#51611,#51612,#51613,#51614,
#51615,#51616,#51617,#51618,#51619,#51620),.UNSPECIFIED.,.F.,.F.,(4,3,3,
3,3,3,3,4),(1.11639350868703,1.99504657739999,2.9925698661,3.9900931548,
4.98761644350001,5.98513973220002,6.98266302090003,7.39957881586659),
 .UNSPECIFIED.);
#1237=B_SPLINE_CURVE_WITH_KNOTS('',3,(#51625,#51626,#51627,#51628,#51629,
#51630,#51631,#51632,#51633,#51634,#51635,#51636,#51637,#51638,#51639,#51640,
#51641,#51642,#51643,#51644,#51645,#51646),.UNSPECIFIED.,.F.,.F.,(4,3,3,
3,3,3,3,4),(-16.6593010344898,-15.9603726192001,-14.9628493305001,-13.9653260418001,
-12.9678027531001,-11.9702794644001,-10.9727561757001,-10.3761157273102),
 .UNSPECIFIED.);
#1238=B_SPLINE_CURVE_WITH_KNOTS('',3,(#51647,#51648,#51649,#51650,#51651,
#51652,#51653,#51654,#51655,#51656,#51657,#51658,#51659,#51660,#51661,#51662,
#51663,#51664,#51665,#51666,#51667,#51668),.UNSPECIFIED.,.F.,.F.,(4,3,3,
3,3,3,3,4),(7.39957881586659,7.98018630960004,8.97770959830006,9.97523288700007,
10.9727561757001,11.9702794644001,12.9678027531001,13.6827641230462),
 .UNSPECIFIED.);
#1239=B_SPLINE_CURVE_WITH_KNOTS('',3,(#51673,#51674,#51675,#51676,#51677,
#51678,#51679,#51680,#51681,#51682,#51683,#51684,#51685,#51686,#51687,#51688,
#51689,#51690,#51691,#51692,#51693,#51694),.UNSPECIFIED.,.F.,.F.,(4,3,3,
3,3,3,3,4),(-22.9424863416694,-21.9455123514001,-20.9479890627001,-19.9504657740001,
-18.9529424853001,-17.9554191966001,-16.9578959079001,-16.6593010344898),
 .UNSPECIFIED.);
#1240=B_SPLINE_CURVE_WITH_KNOTS('',3,(#51695,#51696,#51697,#51698,#51699,
#51700,#51701,#51702,#51703,#51704,#51705,#51706,#51707,#51708,#51709,#51710,
#51711,#51712,#51713,#51714,#51715,#51716,#51717,#51718,#51719),
 .UNSPECIFIED.,.F.,.F.,(4,3,3,3,3,3,3,3,4),(13.6827641230462,13.9653260418001,
14.9628493305001,15.9603726192001,16.9578959079001,17.9554191966001,18.9529424853001,
19.9504657740001,19.9659494302258),.UNSPECIFIED.);
#1241=B_SPLINE_CURVE_WITH_KNOTS('',3,(#51724,#51725,#51726,#51727,#51728,
#51729,#51730,#51731,#51732,#51733,#51734,#51735,#51736,#51737,#51738,#51739,
#51740,#51741,#51742,#51743,#51744,#51745),.UNSPECIFIED.,.F.,.F.,(4,3,3,
3,3,3,3,4),(-29.225671648849,-28.9281753723002,-27.9306520836002,-26.9331287949001,
-25.9356055062001,-24.9380822175001,-23.9405589288001,-22.9424863416694),
 .UNSPECIFIED.);
#1242=B_SPLINE_CURVE_WITH_KNOTS('',3,(#51746,#51747,#51748,#51749,#51750,
#51751,#51752,#51753,#51754,#51755,#51756,#51757,#51758,#51759,#51760,#51761,
#51762,#51763,#51764,#51765,#51766,#51767),.UNSPECIFIED.,.F.,.F.,(4,3,3,
3,3,3,3,4),(19.9659494302258,20.9479890627001,21.9455123514001,22.9430356401001,
23.9405589288002,24.9380822175002,25.9356055062002,26.2491347374054),
 .UNSPECIFIED.);
#1243=B_SPLINE_CURVE_WITH_KNOTS('',3,(#51772,#51773,#51774,#51775,#51776,
#51777,#51778,#51779,#51780,#51781,#51782,#51783,#51784,#51785,#51786,#51787,
#51788,#51789,#51790,#51791,#51792,#51793),.UNSPECIFIED.,.F.,.F.,(4,3,3,
3,3,3,3,4),(-35.5088569560286,-34.9133151045002,-33.9157918158002,-32.9182685271002,
-31.9207452384002,-30.9232219497002,-29.9256986610002,-29.225671648849),
 .UNSPECIFIED.);
#1244=B_SPLINE_CURVE_WITH_KNOTS('',3,(#51794,#51795,#51796,#51797,#51798,
#51799,#51800,#51801,#51802,#51803,#51804,#51805,#51806,#51807,#51808,#51809,
#51810,#51811,#51812,#51813,#51814,#51815),.UNSPECIFIED.,.F.,.F.,(4,3,3,
3,3,3,3,4),(26.2491347374054,26.9331287949002,27.9306520836002,28.9281753723002,
29.9256986610002,30.9232219497002,31.9207452384002,32.532320044585),
 .UNSPECIFIED.);
#1245=B_SPLINE_CURVE_WITH_KNOTS('',3,(#51820,#51821,#51822,#51823,#51824,
#51825,#51826,#51827,#51828,#51829,#51830,#51831,#51832,#51833,#51834,#51835,
#51836,#51837,#51838,#51839,#51840,#51841),.UNSPECIFIED.,.F.,.F.,(4,3,3,
3,3,3,3,4),(-41.7920422632082,-40.8984548367002,-39.9009315480002,-38.9034082593002,
-37.9058849706002,-36.9083616819002,-35.9108383932002,-35.5088569560286),
 .UNSPECIFIED.);
#1246=B_SPLINE_CURVE_WITH_KNOTS('',3,(#51842,#51843,#51844,#51845,#51846,
#51847,#51848,#51849,#51850,#51851,#51852,#51853,#51854,#51855,#51856,#51857,
#51858,#51859,#51860,#51861,#51862,#51863),.UNSPECIFIED.,.F.,.F.,(4,3,3,
3,3,3,3,4),(32.532320044585,32.9182685271002,33.9157918158002,34.9133151045002,
35.9108383932002,36.9083616819002,37.9058849706002,38.8155053517645),
 .UNSPECIFIED.);
#1247=B_SPLINE_CURVE_WITH_KNOTS('',3,(#51868,#51869,#51870,#51871,#51872,
#51873,#51874,#51875,#51876,#51877,#51878,#51879,#51880,#51881,#51882,#51883,
#51884,#51885,#51886,#51887,#51888,#51889,#51890,#51891,#51892),
 .UNSPECIFIED.,.F.,.F.,(4,3,3,3,3,3,3,3,4),(-48.0752275703878,-47.8811178576003,
-46.8835945689003,-45.8860712802002,-44.8885479915002,-43.8910247028002,
-42.8935014141002,-41.8959781254002,-41.7920422632082),.UNSPECIFIED.);
#1248=B_SPLINE_CURVE_WITH_KNOTS('',3,(#51893,#51894,#51895,#51896,#51897,
#51898,#51899,#51900,#51901,#51902,#51903,#51904,#51905,#51906,#51907,#51908,
#51909,#51910,#51911,#51912,#51913,#51914,#51915,#51916,#51917),
 .UNSPECIFIED.,.F.,.F.,(4,3,3,3,3,3,3,3,4),(38.8155053517645,38.9034082593002,
39.9009315480002,40.8984548367002,41.8959781254002,42.8935014141002,43.8910247028003,
44.8885479915003,45.0986906589441),.UNSPECIFIED.);
#1249=B_SPLINE_CURVE_WITH_KNOTS('',3,(#51922,#51923,#51924,#51925,#51926,
#51927,#51928,#51929,#51930,#51931,#51932,#51933,#51934,#51935,#51936,#51937,
#51938,#51939,#51940,#51941,#51942,#51943),.UNSPECIFIED.,.F.,.F.,(4,3,3,
3,3,3,3,4),(-54.3584128775673,-53.8662575898003,-52.8687343011003,-51.8712110124003,
-50.8736877237003,-49.8761644350003,-48.8786411463003,-48.0752275703878),
 .UNSPECIFIED.);
#1250=B_SPLINE_CURVE_WITH_KNOTS('',3,(#51944,#51945,#51946,#51947,#51948,
#51949,#51950,#51951,#51952,#51953,#51954,#51955,#51956,#51957,#51958,#51959,
#51960,#51961,#51962,#51963,#51964,#51965),.UNSPECIFIED.,.F.,.F.,(4,3,3,
3,3,3,3,4),(45.0986906589441,45.8860712802003,46.8835945689003,47.8811178576003,
48.8786411463002,49.8761644350002,50.8736877237002,51.3818759661237),
 .UNSPECIFIED.);
#1251=B_SPLINE_CURVE_WITH_KNOTS('',3,(#51970,#51971,#51972,#51973,#51974,
#51975,#51976,#51977,#51978,#51979,#51980,#51981,#51982,#51983,#51984,#51985,
#51986,#51987,#51988,#51989,#51990,#51991),.UNSPECIFIED.,.F.,.F.,(4,3,3,
3,3,3,3,4),(-60.6415981847469,-59.8513973220003,-58.8538740333003,-57.8563507446003,
-56.8588274559003,-55.8613041672003,-54.8637808785003,-54.3584128775673),
 .UNSPECIFIED.);
#1252=B_SPLINE_CURVE_WITH_KNOTS('',3,(#51992,#51993,#51994,#51995,#51996,
#51997,#51998,#51999,#52000,#52001,#52002,#52003,#52004,#52005,#52006,#52007,
#52008,#52009,#52010,#52011,#52012,#52013),.UNSPECIFIED.,.F.,.F.,(4,3,3,
3,3,3,3,4),(51.3818759661237,51.8712110124002,52.8687343011003,53.8662575898003,
54.8637808785003,55.8613041672003,56.8588274559003,57.6650612733033),
 .UNSPECIFIED.);
#1253=B_SPLINE_CURVE_WITH_KNOTS('',3,(#52018,#52019,#52020,#52021,#52022,
#52023,#52024,#52025,#52026,#52027,#52028,#52029,#52030,#52031,#52032,#52033,
#52034,#52035,#52036,#52037,#52038,#52039,#52040,#52041,#52042),
 .UNSPECIFIED.,.F.,.F.,(4,3,3,3,3,3,3,3,4),(-66.9247834919265,-66.8340603429004,
-65.8365370542004,-64.8390137655004,-63.8414904768003,-62.8439671881003,
-61.8464438994003,-60.8489206107003,-60.6415981847469),.UNSPECIFIED.);
#1254=B_SPLINE_CURVE_WITH_KNOTS('',3,(#52043,#52044,#52045,#52046,#52047,
#52048,#52049,#52050,#52051,#52052,#52053,#52054,#52055,#52056,#52057,#52058,
#52059,#52060,#52061,#52062,#52063,#52064,#52065,#52066,#52067),
 .UNSPECIFIED.,.F.,.F.,(4,3,3,3,3,3,3,3,4),(57.6650612733033,57.8563507446003,
58.8538740333003,59.8513973220003,60.8489206107003,61.8464438994003,62.8439671881003,
63.8414904768003,63.9482465804829),.UNSPECIFIED.);
#1255=B_SPLINE_CURVE_WITH_KNOTS('',3,(#52072,#52073,#52074,#52075,#52076,
#52077,#52078,#52079,#52080,#52081,#52082,#52083,#52084,#52085,#52086,#52087,
#52088,#52089,#52090,#52091,#52092,#52093),.UNSPECIFIED.,.F.,.F.,(4,3,3,
3,3,3,3,4),(-73.2079687991061,-72.8192000751004,-71.8216767864004,-70.8241534977004,
-69.8266302090004,-68.8291069203004,-67.8315836316004,-66.9247834919265),
 .UNSPECIFIED.);
#1256=B_SPLINE_CURVE_WITH_KNOTS('',3,(#52094,#52095,#52096,#52097,#52098,
#52099,#52100,#52101,#52102,#52103,#52104,#52105,#52106,#52107,#52108,#52109,
#52110,#52111,#52112,#52113,#52114,#52115),.UNSPECIFIED.,.F.,.F.,(4,3,3,
3,3,3,3,4),(63.9482465804829,64.8390137655003,65.8365370542003,66.8340603429004,
67.8315836316004,68.8291069203004,69.8266302090004,70.2314318876625),
 .UNSPECIFIED.);
#1257=B_SPLINE_CURVE_WITH_KNOTS('',3,(#52120,#52121,#52122,#52123,#52124,
#52125,#52126,#52127,#52128,#52129,#52130,#52131,#52132,#52133,#52134,#52135,
#52136,#52137,#52138,#52139,#52140,#52141),.UNSPECIFIED.,.F.,.F.,(4,3,3,
3,3,3,3,4),(-79.4911541062857,-78.8043398073004,-77.8068165186004,-76.8092932299004,
-75.8117699412004,-74.8142466525004,-73.8167233638004,-73.2079687991061),
 .UNSPECIFIED.);
#1258=B_SPLINE_CURVE_WITH_KNOTS('',3,(#52142,#52143,#52144,#52145,#52146,
#52147,#52148,#52149,#52150,#52151,#52152,#52153,#52154,#52155,#52156,#52157,
#52158,#52159,#52160,#52161,#52162,#52163),.UNSPECIFIED.,.F.,.F.,(4,3,3,
3,3,3,3,4),(70.2314318876625,70.8241534977004,71.8216767864004,72.8192000751004,
73.8167233638004,74.8142466525004,75.8117699412004,76.5146171948421),
 .UNSPECIFIED.);
#1259=B_SPLINE_CURVE_WITH_KNOTS('',3,(#52168,#52169,#52170,#52171,#52172,
#52173,#52174,#52175,#52176,#52177,#52178,#52179,#52180,#52181,#52182,#52183,
#52184,#52185,#52186,#52187,#52188,#52189),.UNSPECIFIED.,.F.,.F.,(4,3,3,
3,3,3,3,4),(-85.7743394134653,-84.7894795395005,-83.7919562508005,-82.7944329621005,
-81.7969096734005,-80.7993863847005,-79.8018630960004,-79.4911541062857),
 .UNSPECIFIED.);
#1260=B_SPLINE_CURVE_WITH_KNOTS('',3,(#52190,#52191,#52192,#52193,#52194,
#52195,#52196,#52197,#52198,#52199,#52200,#52201,#52202,#52203,#52204,#52205,
#52206,#52207,#52208,#52209,#52210,#52211,#52212,#52213,#52214),
 .UNSPECIFIED.,.F.,.F.,(4,3,3,3,3,3,3,3,4),(76.5146171948421,76.8092932299004,
77.8068165186004,78.8043398073004,79.8018630960004,80.7993863847004,81.7969096734004,
82.7944329621005,82.7978025020217),.UNSPECIFIED.);
#1261=B_SPLINE_CURVE_WITH_KNOTS('',3,(#52219,#52220,#52221,#52222,#52223,
#52224,#52225,#52226,#52227,#52228,#52229,#52230,#52231,#52232,#52233,#52234,
#52235,#52236,#52237,#52238,#52239,#52240,#52241,#52242,#52243),
 .UNSPECIFIED.,.F.,.F.,(4,3,3,3,3,3,3,3,4),(-92.0575247206449,-91.7721425604005,
-90.7746192717005,-89.7770959830005,-88.7795726943005,-87.7820494056005,
-86.7845261169005,-85.7870028282005,-85.7743394134653),.UNSPECIFIED.);
#1262=B_SPLINE_CURVE_WITH_KNOTS('',3,(#52244,#52245,#52246,#52247,#52248,
#52249,#52250,#52251,#52252,#52253,#52254,#52255,#52256,#52257,#52258,#52259,
#52260,#52261,#52262,#52263,#52264,#52265),.UNSPECIFIED.,.F.,.F.,(4,3,3,
3,3,3,3,4),(82.7978025020217,83.7919562508005,84.7894795395004,85.7870028282005,
86.7845261169005,87.7820494056005,88.7795726943005,89.0809878092013),
 .UNSPECIFIED.);
#1263=B_SPLINE_CURVE_WITH_KNOTS('',3,(#52270,#52271,#52272,#52273,#52274,
#52275,#52276,#52277,#52278,#52279,#52280,#52281,#52282,#52283,#52284,#52285,
#52286,#52287,#52288,#52289,#52290,#52291),.UNSPECIFIED.,.F.,.F.,(4,3,3,
3,3,3,3,4),(-98.3407100278245,-97.7572822926005,-96.7597590039005,-95.7622357152005,
-94.7647124265005,-93.7671891378005,-92.7696658491005,-92.0575247206449),
 .UNSPECIFIED.);
#1264=B_SPLINE_CURVE_WITH_KNOTS('',3,(#52292,#52293,#52294,#52295,#52296,
#52297,#52298,#52299,#52300,#52301,#52302,#52303,#52304,#52305,#52306,#52307,
#52308,#52309,#52310,#52311,#52312,#52313),.UNSPECIFIED.,.F.,.F.,(4,3,3,
3,3,3,3,4),(89.0809878092013,89.7770959830005,90.7746192717005,91.7721425604005,
92.7696658491005,93.7671891378005,94.7647124265005,95.3641731163809),
 .UNSPECIFIED.);
#1265=B_SPLINE_CURVE_WITH_KNOTS('',3,(#52318,#52319,#52320,#52321,#52322,
#52323,#52324,#52325,#52326,#52327,#52328,#52329,#52330,#52331,#52332,#52333,
#52334,#52335,#52336,#52337,#52338,#52339),.UNSPECIFIED.,.F.,.F.,(4,3,3,
3,3,3,3,4),(-104.623895335004,-103.742422024801,-102.744898736101,-101.747375447401,
-100.749852158701,-99.7523288700005,-98.7548055813005,-98.3407100278245),
 .UNSPECIFIED.);
#1266=B_SPLINE_CURVE_WITH_KNOTS('',3,(#52340,#52341,#52342,#52343,#52344,
#52345,#52346,#52347,#52348,#52349,#52350,#52351,#52352,#52353,#52354,#52355,
#52356,#52357,#52358,#52359,#52360,#52361),.UNSPECIFIED.,.F.,.F.,(4,3,3,
3,3,3,3,4),(95.3641731163809,95.7622357152005,96.7597590039006,97.7572822926005,
98.7548055813005,99.7523288700006,100.749852158701,101.647358423561),
 .UNSPECIFIED.);
#1267=B_SPLINE_CURVE_WITH_KNOTS('',3,(#52366,#52367,#52368,#52369,#52370,
#52371,#52372,#52373,#52374,#52375,#52376,#52377,#52378,#52379,#52380,#52381,
#52382,#52383,#52384,#52385,#52386,#52387,#52388,#52389,#52390),
 .UNSPECIFIED.,.F.,.F.,(4,3,3,3,3,3,3,3,4),(-110.907080642184,-110.725085045701,
-109.727561757001,-108.730038468301,-107.732515179601,-106.734991890901,
-105.737468602201,-104.739945313501,-104.623895335004),.UNSPECIFIED.);
#1268=B_SPLINE_CURVE_WITH_KNOTS('',3,(#52391,#52392,#52393,#52394,#52395,
#52396,#52397,#52398,#52399,#52400,#52401,#52402,#52403,#52404,#52405,#52406,
#52407,#52408,#52409,#52410,#52411,#52412,#52413,#52414,#52415),
 .UNSPECIFIED.,.F.,.F.,(4,3,3,3,3,3,3,3,4),(101.647358423561,101.747375447401,
102.744898736101,103.742422024801,104.739945313501,105.737468602201,106.734991890901,
107.732515179601,107.93054373074),.UNSPECIFIED.);
#1269=B_SPLINE_CURVE_WITH_KNOTS('',3,(#52420,#52421,#52422,#52423,#52424,
#52425,#52426,#52427,#52428,#52429,#52430,#52431,#52432,#52433,#52434,#52435,
#52436,#52437,#52438,#52439,#52440,#52441),.UNSPECIFIED.,.F.,.F.,(4,3,3,
3,3,3,3,4),(-117.190265949363,-116.710224777901,-115.712701489201,-114.715178200501,
-113.717654911801,-112.720131623101,-111.722608334401,-110.907080642184),
 .UNSPECIFIED.);
#1270=B_SPLINE_CURVE_WITH_KNOTS('',3,(#52442,#52443,#52444,#52445,#52446,
#52447,#52448,#52449,#52450,#52451,#52452,#52453,#52454,#52455,#52456,#52457,
#52458,#52459,#52460,#52461,#52462,#52463),.UNSPECIFIED.,.F.,.F.,(4,3,3,
3,3,3,3,4),(107.93054373074,108.730038468301,109.727561757001,110.725085045701,
111.722608334401,112.720131623101,113.717654911801,114.21372903792),
 .UNSPECIFIED.);
#1271=B_SPLINE_CURVE_WITH_KNOTS('',3,(#52468,#52469,#52470,#52471,#52472,
#52473,#52474,#52475,#52476,#52477,#52478,#52479,#52480,#52481,#52482,#52483,
#52484,#52485,#52486,#52487,#52488,#52489),.UNSPECIFIED.,.F.,.F.,(4,3,3,
3,3,3,3,4),(-123.473451256543,-122.695364510101,-121.697841221401,-120.700317932701,
-119.702794644001,-118.705271355301,-117.707748066601,-117.190265949363),
 .UNSPECIFIED.);
#1272=B_SPLINE_CURVE_WITH_KNOTS('',3,(#52490,#52491,#52492,#52493,#52494,
#52495,#52496,#52497,#52498,#52499,#52500,#52501,#52502,#52503,#52504,#52505,
#52506,#52507,#52508,#52509,#52510,#52511),.UNSPECIFIED.,.F.,.F.,(4,3,3,
3,3,3,3,4),(114.21372903792,114.715178200501,115.712701489201,116.710224777901,
117.707748066601,118.705271355301,119.702794644001,120.496914345099),
 .UNSPECIFIED.);
#1273=B_SPLINE_CURVE_WITH_KNOTS('',3,(#52516,#52517,#52518,#52519,#52520,
#52521,#52522,#52523,#52524,#52525,#52526,#52527,#52528,#52529,#52530,#52531,
#52532,#52533,#52534,#52535,#52536,#52537,#52538,#52539,#52540),
 .UNSPECIFIED.,.F.,.F.,(4,3,3,3,3,3,3,3,4),(-129.756636563722,-129.678027531001,
-128.680504242301,-127.682980953601,-126.685457664901,-125.687934376201,
-124.690411087501,-123.692887798801,-123.473451256543),.UNSPECIFIED.);
#1274=B_SPLINE_CURVE_WITH_KNOTS('',3,(#52541,#52542,#52543,#52544,#52545,
#52546,#52547,#52548,#52549,#52550,#52551,#52552,#52553,#52554,#52555,#52556,
#52557,#52558,#52559,#52560,#52561,#52562,#52563,#52564,#52565),
 .UNSPECIFIED.,.F.,.F.,(4,3,3,3,3,3,3,3,4),(120.496914345099,120.700317932701,
121.697841221401,122.695364510101,123.692887798801,124.690411087501,125.687934376201,
126.685457664901,126.780099652279),.UNSPECIFIED.);
#1275=B_SPLINE_CURVE_WITH_KNOTS('',3,(#52570,#52571,#52572,#52573,#52574,
#52575,#52576,#52577,#52578,#52579,#52580,#52581,#52582,#52583,#52584,#52585,
#52586,#52587,#52588,#52589,#52590,#52591),.UNSPECIFIED.,.F.,.F.,(4,3,3,
3,3,3,3,4),(-136.039821870902,-135.663167263201,-134.665643974501,-133.668120685801,
-132.670597397101,-131.673074108401,-130.675550819701,-129.756636563722),
 .UNSPECIFIED.);
#1276=B_SPLINE_CURVE_WITH_KNOTS('',3,(#52592,#52593,#52594,#52595,#52596,
#52597,#52598,#52599,#52600,#52601,#52602,#52603,#52604,#52605,#52606,#52607,
#52608,#52609,#52610,#52611,#52612,#52613),.UNSPECIFIED.,.F.,.F.,(4,3,3,
3,3,3,3,4),(126.780099652279,127.682980953601,128.680504242301,129.678027531001,
130.675550819701,131.673074108401,132.670597397101,133.063284959458),
 .UNSPECIFIED.);
#1277=B_SPLINE_CURVE_WITH_KNOTS('',3,(#52618,#52619,#52620,#52621,#52622,
#52623,#52624,#52625,#52626,#52627,#52628,#52629,#52630,#52631,#52632,#52633,
#52634,#52635,#52636,#52637,#52638,#52639),.UNSPECIFIED.,.F.,.F.,(4,3,3,
3,3,3,3,4),(-142.323007178082,-141.648306995401,-140.650783706701,-139.653260418001,
-138.655737129301,-137.658213840601,-136.660690551901,-136.039821870902),
 .UNSPECIFIED.);
#1278=B_SPLINE_CURVE_WITH_KNOTS('',3,(#52640,#52641,#52642,#52643,#52644,
#52645,#52646,#52647,#52648,#52649,#52650,#52651,#52652,#52653,#52654,#52655,
#52656,#52657,#52658,#52659,#52660,#52661),.UNSPECIFIED.,.F.,.F.,(4,3,3,
3,3,3,3,4),(133.063284959458,133.668120685801,134.665643974501,135.663167263201,
136.660690551901,137.658213840601,138.655737129301,139.346470266638),
 .UNSPECIFIED.);
#1279=B_SPLINE_CURVE_WITH_KNOTS('',3,(#52666,#52667,#52668,#52669,#52670,
#52671,#52672,#52673,#52674,#52675,#52676,#52677,#52678,#52679,#52680,#52681,
#52682,#52683,#52684,#52685,#52686,#52687),.UNSPECIFIED.,.F.,.F.,(4,3,3,
3,3,3,3,4),(-148.606192485261,-147.633446727601,-146.635923438901,-145.638400150201,
-144.640876861501,-143.643353572801,-142.645830284101,-142.323007178082),
 .UNSPECIFIED.);
#1280=B_SPLINE_CURVE_WITH_KNOTS('',3,(#52688,#52689,#52690,#52691,#52692,
#52693,#52694,#52695,#52696,#52697,#52698,#52699,#52700,#52701,#52702,#52703,
#52704,#52705,#52706,#52707,#52708,#52709),.UNSPECIFIED.,.F.,.F.,(4,3,3,
3,3,3,3,4),(139.346470266638,139.653260418001,140.650783706701,141.648306995401,
142.645830284101,143.643353572801,144.640876861501,145.629655573818),
 .UNSPECIFIED.);
#1281=B_SPLINE_CURVE_WITH_KNOTS('',3,(#52714,#52715,#52716,#52717,#52718,
#52719,#52720,#52721,#52722,#52723,#52724,#52725,#52726,#52727,#52728,#52729,
#52730,#52731,#52732,#52733,#52734,#52735,#52736,#52737,#52738),
 .UNSPECIFIED.,.F.,.F.,(4,3,3,3,3,3,3,3,4),(-154.889377792441,-154.616109748501,
-153.618586459801,-152.621063171101,-151.623539882401,-150.626016593701,
-149.628493305001,-148.630970016301,-148.606192485261),.UNSPECIFIED.);
#1282=B_SPLINE_CURVE_WITH_KNOTS('',3,(#52739,#52740,#52741,#52742,#52743,
#52744,#52745,#52746,#52747,#52748,#52749,#52750,#52751,#52752,#52753,#52754,
#52755,#52756,#52757,#52758,#52759,#52760,#52761,#52762,#52763),
 .UNSPECIFIED.,.F.,.F.,(4,3,3,3,3,3,3,3,4),(145.629655573818,145.638400150201,
146.635923438901,147.633446727601,148.630970016301,149.628493305001,150.626016593701,
151.623539882401,151.912840880997),.UNSPECIFIED.);
#1283=B_SPLINE_CURVE_WITH_KNOTS('',3,(#52768,#52769,#52770,#52771,#52772,
#52773,#52774,#52775,#52776,#52777,#52778,#52779,#52780,#52781,#52782,#52783,
#52784,#52785,#52786,#52787,#52788,#52789),.UNSPECIFIED.,.F.,.F.,(4,3,3,
3,3,3,3,4),(-161.17256309962,-160.601249480701,-159.603726192001,-158.606202903301,
-157.608679614601,-156.611156325901,-155.613633037201,-154.889377792441),
 .UNSPECIFIED.);
#1284=B_SPLINE_CURVE_WITH_KNOTS('',3,(#52790,#52791,#52792,#52793,#52794,
#52795,#52796,#52797,#52798,#52799,#52800,#52801,#52802,#52803,#52804,#52805,
#52806,#52807,#52808,#52809,#52810,#52811),.UNSPECIFIED.,.F.,.F.,(4,3,3,
3,3,3,3,4),(151.912840880997,152.621063171101,153.618586459801,154.616109748501,
155.613633037201,156.611156325901,157.608679614601,158.196026188177),
 .UNSPECIFIED.);
#1285=B_SPLINE_CURVE_WITH_KNOTS('',3,(#52816,#52817,#52818,#52819,#52820,
#52821,#52822,#52823,#52824,#52825,#52826,#52827,#52828,#52829,#52830,#52831,
#52832,#52833,#52834,#52835,#52836,#52837),.UNSPECIFIED.,.F.,.F.,(4,3,3,
3,3,3,3,4),(-167.4557484068,-166.586389212901,-165.588865924201,-164.591342635501,
-163.593819346801,-162.596296058101,-161.598772769401,-161.17256309962),
 .UNSPECIFIED.);
#1286=B_SPLINE_CURVE_WITH_KNOTS('',3,(#52838,#52839,#52840,#52841,#52842,
#52843,#52844,#52845,#52846,#52847,#52848,#52849,#52850,#52851,#52852,#52853,
#52854,#52855,#52856,#52857,#52858,#52859),.UNSPECIFIED.,.F.,.F.,(4,3,3,
3,3,3,3,4),(158.196026188177,158.606202903301,159.603726192001,160.601249480701,
161.598772769401,162.596296058101,163.593819346801,164.479211495356),
 .UNSPECIFIED.);
#1287=B_SPLINE_CURVE_WITH_KNOTS('',3,(#52864,#52865,#52866,#52867,#52868,
#52869,#52870,#52871,#52872,#52873,#52874,#52875,#52876,#52877,#52878,#52879,
#52880,#52881,#52882,#52883,#52884,#52885,#52886,#52887,#52888),
 .UNSPECIFIED.,.F.,.F.,(4,3,3,3,3,3,3,3,4),(-173.738933713979,-173.569052233801,
-172.571528945101,-171.574005656401,-170.576482367701,-169.578959079001,
-168.581435790301,-167.583912501601,-167.4557484068),.UNSPECIFIED.);
#1288=B_SPLINE_CURVE_WITH_KNOTS('',3,(#52889,#52890,#52891,#52892,#52893,
#52894,#52895,#52896,#52897,#52898,#52899,#52900,#52901,#52902,#52903,#52904,
#52905,#52906,#52907,#52908,#52909,#52910,#52911,#52912,#52913),
 .UNSPECIFIED.,.F.,.F.,(4,3,3,3,3,3,3,3,4),(164.479211495356,164.591342635501,
165.588865924201,166.586389212901,167.583912501601,168.581435790301,169.578959079001,
170.576482367701,170.762396802536),.UNSPECIFIED.);
#1289=B_SPLINE_CURVE_WITH_KNOTS('',3,(#52918,#52919,#52920,#52921,#52922,
#52923,#52924,#52925,#52926,#52927,#52928,#52929,#52930,#52931,#52932,#52933,
#52934,#52935,#52936,#52937,#52938,#52939),.UNSPECIFIED.,.F.,.F.,(4,3,3,
3,3,3,3,4),(-180.022119021159,-179.554191966001,-178.556668677301,-177.559145388601,
-176.561622099901,-175.564098811201,-174.566575522501,-173.738933713979),
 .UNSPECIFIED.);
#1290=B_SPLINE_CURVE_WITH_KNOTS('',3,(#52940,#52941,#52942,#52943,#52944,
#52945,#52946,#52947,#52948,#52949,#52950,#52951,#52952,#52953,#52954,#52955,
#52956,#52957,#52958,#52959,#52960,#52961),.UNSPECIFIED.,.F.,.F.,(4,3,3,
3,3,3,3,4),(170.762396802536,171.574005656401,172.571528945101,173.569052233801,
174.566575522501,175.564098811201,176.561622099901,177.045582109715),
 .UNSPECIFIED.);
#1291=B_SPLINE_CURVE_WITH_KNOTS('',3,(#52966,#52967,#52968,#52969,#52970,
#52971,#52972,#52973,#52974,#52975,#52976,#52977,#52978,#52979,#52980,#52981,
#52982,#52983,#52984,#52985,#52986,#52987),.UNSPECIFIED.,.F.,.F.,(4,3,3,
3,3,3,3,4),(-186.305304328338,-185.539331698201,-184.541808409501,-183.544285120801,
-182.546761832101,-181.549238543401,-180.551715254701,-180.022119021159),
 .UNSPECIFIED.);
#1292=B_SPLINE_CURVE_WITH_KNOTS('',3,(#52988,#52989,#52990,#52991,#52992,
#52993,#52994,#52995,#52996,#52997,#52998,#52999,#53000,#53001,#53002,#53003,
#53004,#53005,#53006,#53007,#53008,#53009),.UNSPECIFIED.,.F.,.F.,(4,3,3,
3,3,3,3,4),(177.045582109715,177.559145388601,178.556668677301,179.554191966001,
180.551715254701,181.549238543401,182.546761832101,183.328767416895),
 .UNSPECIFIED.);
#1293=B_SPLINE_CURVE_WITH_KNOTS('',3,(#53014,#53015,#53016,#53017,#53018,
#53019,#53020,#53021,#53022,#53023,#53024,#53025,#53026,#53027,#53028,#53029,
#53030,#53031,#53032,#53033,#53034,#53035,#53036,#53037,#53038),
 .UNSPECIFIED.,.F.,.F.,(4,3,3,3,3,3,3,3,4),(-192.588489635518,-192.521994719101,
-191.524471430401,-190.526948141701,-189.529424853001,-188.531901564301,
-187.534378275601,-186.536854986901,-186.305304328338),.UNSPECIFIED.);
#1294=B_SPLINE_CURVE_WITH_KNOTS('',3,(#53039,#53040,#53041,#53042,#53043,
#53044,#53045,#53046,#53047,#53048,#53049,#53050,#53051,#53052,#53053,#53054,
#53055,#53056,#53057,#53058,#53059,#53060,#53061,#53062,#53063),
 .UNSPECIFIED.,.F.,.F.,(4,3,3,3,3,3,3,3,4),(183.328767416895,183.544285120801,
184.541808409501,185.539331698201,186.536854986901,187.534378275601,188.531901564301,
189.529424853001,189.611952724075),.UNSPECIFIED.);
#1295=B_SPLINE_CURVE_WITH_KNOTS('',3,(#53068,#53069,#53070,#53071,#53072,
#53073,#53074,#53075,#53076,#53077,#53078,#53079,#53080,#53081,#53082,#53083,
#53084,#53085,#53086,#53087,#53088,#53089),.UNSPECIFIED.,.F.,.F.,(4,3,3,
3,3,3,3,4),(-198.871674942698,-198.507134451301,-197.509611162601,-196.512087873901,
-195.514564585201,-194.517041296501,-193.519518007801,-192.588489635518),
 .UNSPECIFIED.);
#1296=B_SPLINE_CURVE_WITH_KNOTS('',3,(#53090,#53091,#53092,#53093,#53094,
#53095,#53096,#53097,#53098,#53099,#53100,#53101,#53102,#53103,#53104,#53105,
#53106,#53107,#53108,#53109,#53110,#53111),.UNSPECIFIED.,.F.,.F.,(4,3,3,
3,3,3,3,4),(189.611952724075,190.526948141701,191.524471430401,192.521994719101,
193.519518007801,194.517041296501,195.514564585201,195.895138031254),
 .UNSPECIFIED.);
#1297=B_SPLINE_CURVE_WITH_KNOTS('',3,(#53116,#53117,#53118,#53119,#53120,
#53121,#53122,#53123,#53124,#53125,#53126,#53127,#53128,#53129,#53130,#53131,
#53132,#53133,#53134,#53135,#53136,#53137),.UNSPECIFIED.,.F.,.F.,(4,3,3,
3,3,3,3,4),(-205.154860249877,-204.492274183501,-203.494750894801,-202.497227606101,
-201.499704317401,-200.502181028701,-199.504657740001,-198.871674942698),
 .UNSPECIFIED.);
#1298=B_SPLINE_CURVE_WITH_KNOTS('',3,(#53138,#53139,#53140,#53141,#53142,
#53143,#53144,#53145,#53146,#53147,#53148,#53149,#53150,#53151,#53152,#53153,
#53154,#53155,#53156,#53157,#53158,#53159),.UNSPECIFIED.,.F.,.F.,(4,3,3,
3,3,3,3,4),(195.895138031254,196.512087873901,197.509611162601,198.507134451301,
199.504657740001,200.502181028701,201.499704317401,202.178323338434),
 .UNSPECIFIED.);
#1299=B_SPLINE_CURVE_WITH_KNOTS('',3,(#53164,#53165,#53166,#53167,#53168,
#53169,#53170,#53171,#53172,#53173,#53174,#53175,#53176,#53177,#53178,#53179,
#53180,#53181,#53182,#53183,#53184,#53185),.UNSPECIFIED.,.F.,.F.,(4,3,3,
3,3,3,3,4),(-211.438045557057,-210.477413915701,-209.479890627001,-208.482367338301,
-207.484844049601,-206.487320760901,-205.489797472201,-205.154860249877),
 .UNSPECIFIED.);
#1300=B_SPLINE_CURVE_WITH_KNOTS('',3,(#53186,#53187,#53188,#53189,#53190,
#53191,#53192,#53193,#53194,#53195,#53196,#53197,#53198,#53199,#53200,#53201,
#53202,#53203,#53204,#53205,#53206,#53207),.UNSPECIFIED.,.F.,.F.,(4,3,3,
3,3,3,3,4),(202.178323338434,202.497227606101,203.494750894801,204.492274183501,
205.489797472201,206.487320760901,207.484844049601,208.461508645613),
 .UNSPECIFIED.);
#1301=B_SPLINE_CURVE_WITH_KNOTS('',3,(#53212,#53213,#53214,#53215,#53216,
#53217,#53218,#53219,#53220,#53221,#53222,#53223,#53224,#53225,#53226,#53227,
#53228,#53229,#53230,#53231,#53232,#53233,#53234,#53235,#53236),
 .UNSPECIFIED.,.F.,.F.,(4,3,3,3,3,3,3,3,4),(-217.721230864236,-217.460076936601,
-216.462553647901,-215.465030359201,-214.467507070501,-213.469983781801,
-212.472460493101,-211.474937204401,-211.438045557057),.UNSPECIFIED.);
#1302=B_SPLINE_CURVE_WITH_KNOTS('',3,(#53237,#53238,#53239,#53240,#53241,
#53242,#53243,#53244,#53245,#53246,#53247,#53248,#53249,#53250,#53251,#53252,
#53253,#53254,#53255,#53256,#53257,#53258,#53259,#53260,#53261),
 .UNSPECIFIED.,.F.,.F.,(4,3,3,3,3,3,3,3,4),(208.461508645613,208.482367338301,
209.479890627001,210.477413915701,211.474937204401,212.472460493101,213.469983781801,
214.467507070501,214.744693952793),.UNSPECIFIED.);
#1303=B_SPLINE_CURVE_WITH_KNOTS('',3,(#53266,#53267,#53268,#53269,#53270,
#53271,#53272,#53273,#53274,#53275,#53276,#53277,#53278,#53279,#53280,#53281,
#53282,#53283,#53284,#53285,#53286,#53287),.UNSPECIFIED.,.F.,.F.,(4,3,3,
3,3,3,3,4),(-224.004416171416,-223.445216668801,-222.447693380101,-221.450170091401,
-220.452646802701,-219.455123514001,-218.457600225301,-217.721230864236),
 .UNSPECIFIED.);
#1304=B_SPLINE_CURVE_WITH_KNOTS('',3,(#53288,#53289,#53290,#53291,#53292,
#53293,#53294,#53295,#53296,#53297,#53298,#53299,#53300,#53301,#53302,#53303,
#53304,#53305,#53306,#53307,#53308,#53309),.UNSPECIFIED.,.F.,.F.,(4,3,3,
3,3,3,3,4),(214.744693952793,215.465030359201,216.462553647901,217.460076936601,
218.457600225301,219.455123514001,220.452646802701,221.027879259972),
 .UNSPECIFIED.);
#1305=B_SPLINE_CURVE_WITH_KNOTS('',3,(#53314,#53315,#53316,#53317,#53318,
#53319,#53320,#53321,#53322,#53323,#53324,#53325,#53326,#53327,#53328,#53329,
#53330,#53331,#53332,#53333,#53334,#53335),.UNSPECIFIED.,.F.,.F.,(4,3,3,
3,3,3,3,4),(-230.287601478595,-229.430356401001,-228.432833112301,-227.435309823601,
-226.437786534901,-225.440263246201,-224.442739957501,-224.004416171416),
 .UNSPECIFIED.);
#1306=B_SPLINE_CURVE_WITH_KNOTS('',3,(#53336,#53337,#53338,#53339,#53340,
#53341,#53342,#53343,#53344,#53345,#53346,#53347,#53348,#53349,#53350,#53351,
#53352,#53353,#53354,#53355,#53356,#53357),.UNSPECIFIED.,.F.,.F.,(4,3,3,
3,3,3,3,4),(221.027879259972,221.450170091401,222.447693380101,223.445216668801,
224.442739957501,225.440263246201,226.437786534901,227.311064567152),
 .UNSPECIFIED.);
#1307=B_SPLINE_CURVE_WITH_KNOTS('',3,(#53362,#53363,#53364,#53365,#53366,
#53367,#53368,#53369,#53370,#53371,#53372,#53373,#53374,#53375,#53376,#53377,
#53378,#53379,#53380,#53381,#53382,#53383,#53384,#53385,#53386),
 .UNSPECIFIED.,.F.,.F.,(4,3,3,3,3,3,3,3,4),(-236.570786785775,-236.413019421901,
-235.415496133201,-234.417972844501,-233.420449555801,-232.422926267101,
-231.425402978401,-230.427879689701,-230.287601478595),.UNSPECIFIED.);
#1308=B_SPLINE_CURVE_WITH_KNOTS('',3,(#53387,#53388,#53389,#53390,#53391,
#53392,#53393,#53394,#53395,#53396,#53397,#53398,#53399,#53400,#53401,#53402,
#53403,#53404,#53405,#53406,#53407,#53408,#53409,#53410,#53411),
 .UNSPECIFIED.,.F.,.F.,(4,3,3,3,3,3,3,3,4),(227.311064567152,227.435309823601,
228.432833112301,229.430356401001,230.427879689701,231.425402978401,232.422926267101,
233.420449555801,233.594249874331),.UNSPECIFIED.);
#1309=B_SPLINE_CURVE_WITH_KNOTS('',3,(#53416,#53417,#53418,#53419,#53420,
#53421,#53422,#53423,#53424,#53425,#53426,#53427,#53428,#53429,#53430,#53431,
#53432,#53433,#53434,#53435,#53436,#53437),.UNSPECIFIED.,.F.,.F.,(4,3,3,
3,3,3,3,4),(-242.853972092955,-242.398159154101,-241.400635865401,-240.403112576701,
-239.405589288001,-238.408065999301,-237.410542710601,-236.570786785775),
 .UNSPECIFIED.);
#1310=B_SPLINE_CURVE_WITH_KNOTS('',3,(#53438,#53439,#53440,#53441,#53442,
#53443,#53444,#53445,#53446,#53447,#53448,#53449,#53450,#53451,#53452,#53453,
#53454,#53455,#53456,#53457,#53458,#53459),.UNSPECIFIED.,.F.,.F.,(4,3,3,
3,3,3,3,4),(233.594249874331,234.417972844501,235.415496133201,236.413019421901,
237.410542710601,238.408065999301,239.405589288001,239.877435181511),
 .UNSPECIFIED.);
#1311=B_SPLINE_CURVE_WITH_KNOTS('',3,(#53464,#53465,#53466,#53467,#53468,
#53469,#53470,#53471,#53472,#53473,#53474,#53475,#53476,#53477,#53478,#53479,
#53480,#53481,#53482,#53483,#53484,#53485),.UNSPECIFIED.,.F.,.F.,(4,3,3,
3,3,3,3,4),(-249.137157400134,-248.383298886301,-247.385775597601,-246.388252308901,
-245.390729020201,-244.393205731501,-243.395682442801,-242.853972092955),
 .UNSPECIFIED.);
#1312=B_SPLINE_CURVE_WITH_KNOTS('',3,(#53486,#53487,#53488,#53489,#53490,
#53491,#53492,#53493,#53494,#53495,#53496,#53497,#53498,#53499,#53500,#53501,
#53502,#53503,#53504,#53505,#53506,#53507),.UNSPECIFIED.,.F.,.F.,(4,3,3,
3,3,3,3,4),(239.877435181511,240.403112576701,241.400635865401,242.398159154101,
243.395682442801,244.393205731501,245.390729020201,246.160620488691),
 .UNSPECIFIED.);
#1313=B_SPLINE_CURVE_WITH_KNOTS('',3,(#53512,#53513,#53514,#53515,#53516,
#53517,#53518,#53519,#53520,#53521,#53522,#53523,#53524,#53525,#53526,#53527,
#53528,#53529,#53530,#53531,#53532,#53533,#53534,#53535,#53536),
 .UNSPECIFIED.,.F.,.F.,(4,3,3,3,3,3,3,3,4),(-255.420342707314,-255.365961907201,
-254.368438618501,-253.370915329801,-252.373392041101,-251.375868752401,
-250.378345463701,-249.380822175001,-249.137157400134),.UNSPECIFIED.);
#1314=B_SPLINE_CURVE_WITH_KNOTS('',3,(#53537,#53538,#53539,#53540,#53541,
#53542,#53543,#53544,#53545,#53546,#53547,#53548,#53549,#53550,#53551,#53552,
#53553,#53554,#53555,#53556,#53557,#53558,#53559,#53560,#53561),
 .UNSPECIFIED.,.F.,.F.,(4,3,3,3,3,3,3,3,4),(246.160620488691,246.388252308901,
247.385775597601,248.383298886301,249.380822175001,250.378345463701,251.375868752401,
252.373392041101,252.44380579587),.UNSPECIFIED.);
#1315=B_SPLINE_CURVE_WITH_KNOTS('',3,(#53566,#53567,#53568,#53569,#53570,
#53571,#53572,#53573,#53574,#53575,#53576,#53577,#53578,#53579,#53580,#53581,
#53582,#53583,#53584,#53585,#53586,#53587),.UNSPECIFIED.,.F.,.F.,(4,3,3,
3,3,3,3,4),(-261.703528014493,-261.351101639401,-260.353578350701,-259.356055062001,
-258.358531773301,-257.361008484601,-256.363485195901,-255.420342707314),
 .UNSPECIFIED.);
#1316=B_SPLINE_CURVE_WITH_KNOTS('',3,(#53588,#53589,#53590,#53591,#53592,
#53593,#53594,#53595,#53596,#53597,#53598,#53599,#53600,#53601,#53602,#53603,
#53604,#53605,#53606,#53607,#53608,#53609),.UNSPECIFIED.,.F.,.F.,(4,3,3,
3,3,3,3,4),(252.44380579587,253.370915329801,254.368438618501,255.365961907201,
256.363485195901,257.361008484601,258.358531773301,258.72699110305),
 .UNSPECIFIED.);
#1317=B_SPLINE_CURVE_WITH_KNOTS('',3,(#53614,#53615,#53616,#53617,#53618,
#53619,#53620,#53621,#53622,#53623,#53624,#53625,#53626,#53627,#53628,#53629,
#53630,#53631,#53632,#53633,#53634,#53635),.UNSPECIFIED.,.F.,.F.,(4,3,3,
3,3,3,3,4),(-267.986713321673,-267.336241371601,-266.338718082901,-265.341194794201,
-264.343671505501,-263.346148216802,-262.348624928101,-261.703528014493),
 .UNSPECIFIED.);
#1318=B_SPLINE_CURVE_WITH_KNOTS('',3,(#53636,#53637,#53638,#53639,#53640,
#53641,#53642,#53643,#53644,#53645,#53646,#53647,#53648,#53649,#53650,#53651,
#53652,#53653,#53654,#53655,#53656,#53657),.UNSPECIFIED.,.F.,.F.,(4,3,3,
3,3,3,3,4),(258.72699110305,259.356055062001,260.353578350701,261.351101639402,
262.348624928102,263.346148216802,264.343671505502,265.010176410229),
 .UNSPECIFIED.);
#1319=B_SPLINE_CURVE_WITH_KNOTS('',3,(#53662,#53663,#53664,#53665,#53666,
#53667,#53668,#53669,#53670,#53671,#53672,#53673,#53674,#53675,#53676,#53677,
#53678,#53679,#53680,#53681,#53682,#53683),.UNSPECIFIED.,.F.,.F.,(4,3,3,
3,3,3,3,4),(-274.269898628852,-273.321381103802,-272.323857815102,-271.326334526402,
-270.328811237701,-269.331287949001,-268.333764660301,-267.986713321673),
 .UNSPECIFIED.);
#1320=B_SPLINE_CURVE_WITH_KNOTS('',3,(#53684,#53685,#53686,#53687,#53688,
#53689,#53690,#53691,#53692,#53693,#53694,#53695,#53696,#53697,#53698,#53699,
#53700,#53701,#53702,#53703,#53704,#53705),.UNSPECIFIED.,.F.,.F.,(4,3,3,
3,3,3,3,4),(265.010176410229,265.341194794201,266.338718082902,267.336241371602,
268.333764660302,269.331287949002,270.328811237702,271.293361717409),
 .UNSPECIFIED.);
#1321=B_SPLINE_CURVE_WITH_KNOTS('',3,(#53710,#53711,#53712,#53713,#53714,
#53715,#53716,#53717,#53718,#53719,#53720,#53721,#53722,#53723,#53724,#53725,
#53726,#53727,#53728,#53729,#53730,#53731,#53732,#53733,#53734),
 .UNSPECIFIED.,.F.,.F.,(4,3,3,3,3,3,3,3,4),(-280.553083936032,-280.304044124702,
-279.306520836001,-278.308997547301,-277.311474258601,-276.313950969901,
-275.316427681202,-274.318904392502,-274.269898628852),.UNSPECIFIED.);
#1322=B_SPLINE_CURVE_WITH_KNOTS('',3,(#53735,#53736,#53737,#53738,#53739,
#53740,#53741,#53742,#53743,#53744,#53745,#53746,#53747,#53748,#53749,#53750,
#53751,#53752,#53753,#53754,#53755,#53756,#53757,#53758,#53759),
 .UNSPECIFIED.,.F.,.F.,(4,3,3,3,3,3,3,3,4),(271.293361717409,271.326334526402,
272.323857815102,273.321381103802,274.318904392502,275.316427681202,276.313950969902,
277.311474258602,277.576547024588),.UNSPECIFIED.);
#1323=B_SPLINE_CURVE_WITH_KNOTS('',3,(#53764,#53765,#53766,#53767,#53768,
#53769,#53770,#53771,#53772,#53773,#53774,#53775,#53776,#53777,#53778,#53779,
#53780,#53781,#53782,#53783,#53784,#53785),.UNSPECIFIED.,.F.,.F.,(4,3,3,
3,3,3,3,4),(-286.836269243212,-286.289183856902,-285.291660568202,-284.294137279502,
-283.296613990802,-282.299090702102,-281.301567413402,-280.553083936032),
 .UNSPECIFIED.);
#1324=B_SPLINE_CURVE_WITH_KNOTS('',3,(#53786,#53787,#53788,#53789,#53790,
#53791,#53792,#53793,#53794,#53795,#53796,#53797,#53798,#53799,#53800,#53801,
#53802,#53803,#53804,#53805,#53806,#53807),.UNSPECIFIED.,.F.,.F.,(4,3,3,
3,3,3,3,4),(277.576547024588,278.308997547302,279.306520836002,280.304044124702,
281.301567413402,282.299090702102,283.296613990802,283.859732331768),
 .UNSPECIFIED.);
#1325=B_SPLINE_CURVE_WITH_KNOTS('',3,(#53812,#53813,#53814,#53815,#53816,
#53817,#53818,#53819,#53820,#53821,#53822,#53823,#53824,#53825,#53826,#53827,
#53828,#53829,#53830,#53831,#53832,#53833),.UNSPECIFIED.,.F.,.F.,(4,3,3,
3,3,3,3,4),(-293.119454550391,-292.274323589102,-291.276800300402,-290.279277011702,
-289.281753723002,-288.284230434302,-287.286707145602,-286.836269243212),
 .UNSPECIFIED.);
#1326=B_SPLINE_CURVE_WITH_KNOTS('',3,(#53834,#53835,#53836,#53837,#53838,
#53839,#53840,#53841,#53842,#53843,#53844,#53845,#53846,#53847,#53848,#53849,
#53850,#53851,#53852,#53853,#53854,#53855),.UNSPECIFIED.,.F.,.F.,(4,3,3,
3,3,3,3,4),(283.859732331768,284.294137279502,285.291660568202,286.289183856902,
287.286707145602,288.284230434302,289.281753723002,290.142917638947),
 .UNSPECIFIED.);
#1327=B_SPLINE_CURVE_WITH_KNOTS('',3,(#53860,#53861,#53862,#53863,#53864,
#53865,#53866,#53867,#53868,#53869,#53870,#53871,#53872,#53873,#53874,#53875,
#53876,#53877,#53878,#53879,#53880,#53881,#53882,#53883,#53884),
 .UNSPECIFIED.,.F.,.F.,(4,3,3,3,3,3,3,3,4),(-299.402639857571,-299.256986610002,
-298.259463321302,-297.261940032602,-296.264416743902,-295.266893455202,
-294.269370166502,-293.271846877802,-293.119454550391),.UNSPECIFIED.);
#1328=B_SPLINE_CURVE_WITH_KNOTS('',3,(#53885,#53886,#53887,#53888,#53889,
#53890,#53891,#53892,#53893,#53894,#53895,#53896,#53897,#53898,#53899,#53900,
#53901,#53902,#53903,#53904,#53905,#53906,#53907,#53908,#53909),
 .UNSPECIFIED.,.F.,.F.,(4,3,3,3,3,3,3,3,4),(290.142917638947,290.279277011702,
291.276800300402,292.274323589102,293.271846877802,294.269370166502,295.266893455202,
296.264416743902,296.426102946127),.UNSPECIFIED.);
#1329=B_SPLINE_CURVE_WITH_KNOTS('',3,(#53914,#53915,#53916,#53917,#53918,
#53919,#53920,#53921,#53922,#53923,#53924,#53925,#53926,#53927,#53928,#53929,
#53930,#53931,#53932,#53933,#53934,#53935),.UNSPECIFIED.,.F.,.F.,(4,3,3,
3,3,3,3,4),(-305.68582516475,-305.242126342202,-304.244603053502,-303.247079764802,
-302.249556476102,-301.252033187402,-300.254509898702,-299.402639857571),
 .UNSPECIFIED.);
#1330=B_SPLINE_CURVE_WITH_KNOTS('',3,(#53936,#53937,#53938,#53939,#53940,
#53941,#53942,#53943,#53944,#53945,#53946,#53947,#53948,#53949,#53950,#53951,
#53952,#53953,#53954,#53955,#53956,#53957),.UNSPECIFIED.,.F.,.F.,(4,3,3,
3,3,3,3,4),(296.426102946127,297.261940032602,298.259463321302,299.256986610002,
300.254509898702,301.252033187402,302.249556476102,302.709288253307),
 .UNSPECIFIED.);
#1331=B_SPLINE_CURVE_WITH_KNOTS('',3,(#53962,#53963,#53964,#53965,#53966,
#53967,#53968,#53969,#53970,#53971,#53972,#53973,#53974,#53975,#53976,#53977,
#53978,#53979,#53980,#53981,#53982,#53983),.UNSPECIFIED.,.F.,.F.,(4,3,3,
3,3,3,3,4),(-311.96901047193,-311.227266074402,-310.229742785702,-309.232219497002,
-308.234696208302,-307.237172919602,-306.239649630902,-305.68582516475),
 .UNSPECIFIED.);
#1332=B_SPLINE_CURVE_WITH_KNOTS('',3,(#53984,#53985,#53986,#53987,#53988,
#53989,#53990,#53991,#53992,#53993,#53994,#53995,#53996,#53997,#53998,#53999,
#54000,#54001,#54002,#54003,#54004,#54005),.UNSPECIFIED.,.F.,.F.,(4,3,3,
3,3,3,3,4),(302.709288253307,303.247079764802,304.244603053502,305.242126342202,
306.239649630902,307.237172919602,308.234696208302,308.992473560486),
 .UNSPECIFIED.);
#1333=B_SPLINE_CURVE_WITH_KNOTS('',3,(#54010,#54011,#54012,#54013,#54014,
#54015,#54016,#54017,#54018,#54019,#54020,#54021,#54022,#54023,#54024,#54025,
#54026,#54027,#54028,#54029,#54030,#54031,#54032,#54033,#54034),
 .UNSPECIFIED.,.F.,.F.,(4,3,3,3,3,3,3,3,4),(-318.252195779109,-318.209929095302,
-317.212405806602,-316.214882517902,-315.217359229202,-314.219835940502,
-313.222312651802,-312.224789363102,-311.96901047193),.UNSPECIFIED.);
#1334=B_SPLINE_CURVE_WITH_KNOTS('',3,(#54035,#54036,#54037,#54038,#54039,
#54040,#54041,#54042,#54043,#54044,#54045,#54046,#54047,#54048,#54049,#54050,
#54051,#54052,#54053,#54054,#54055,#54056,#54057,#54058,#54059),
 .UNSPECIFIED.,.F.,.F.,(4,3,3,3,3,3,3,3,4),(308.992473560486,309.232219497002,
310.229742785702,311.227266074402,312.224789363102,313.222312651802,314.219835940502,
315.217359229202,315.275658867666),.UNSPECIFIED.);
#1335=B_SPLINE_CURVE_WITH_KNOTS('',3,(#54064,#54065,#54066,#54067,#54068,
#54069,#54070,#54071,#54072,#54073,#54074,#54075,#54076,#54077,#54078,#54079,
#54080,#54081,#54082,#54083,#54084,#54085),.UNSPECIFIED.,.F.,.F.,(4,3,3,
3,3,3,3,4),(-324.535381086289,-324.195068827502,-323.197545538802,-322.200022250102,
-321.202498961402,-320.204975672702,-319.207452384002,-318.252195779109),
 .UNSPECIFIED.);
#1336=B_SPLINE_CURVE_WITH_KNOTS('',3,(#54086,#54087,#54088,#54089,#54090,
#54091,#54092,#54093,#54094,#54095,#54096,#54097,#54098,#54099,#54100,#54101,
#54102,#54103,#54104,#54105,#54106,#54107),.UNSPECIFIED.,.F.,.F.,(4,3,3,
3,3,3,3,4),(315.275658867666,316.214882517902,317.212405806602,318.209929095302,
319.207452384002,320.204975672702,321.202498961402,321.558844174845),
 .UNSPECIFIED.);
#1337=B_SPLINE_CURVE_WITH_KNOTS('',3,(#54112,#54113,#54114,#54115,#54116,
#54117,#54118,#54119,#54120,#54121,#54122,#54123,#54124,#54125,#54126,#54127,
#54128,#54129,#54130,#54131,#54132,#54133),.UNSPECIFIED.,.F.,.F.,(4,3,3,
3,3,3,3,4),(-330.818566393468,-330.180208559702,-329.182685271002,-328.185161982302,
-327.187638693602,-326.190115404902,-325.192592116202,-324.535381086289),
 .UNSPECIFIED.);
#1338=B_SPLINE_CURVE_WITH_KNOTS('',3,(#54134,#54135,#54136,#54137,#54138,
#54139,#54140,#54141,#54142,#54143,#54144,#54145,#54146,#54147,#54148,#54149,
#54150,#54151,#54152,#54153,#54154,#54155),.UNSPECIFIED.,.F.,.F.,(4,3,3,
3,3,3,3,4),(321.558844174845,322.200022250102,323.197545538802,324.195068827502,
325.192592116202,326.190115404902,327.187638693602,327.842029482025),
 .UNSPECIFIED.);
#1339=B_SPLINE_CURVE_WITH_KNOTS('',3,(#54160,#54161,#54162,#54163,#54164,
#54165,#54166,#54167,#54168,#54169,#54170,#54171,#54172,#54173,#54174,#54175,
#54176,#54177,#54178,#54179,#54180,#54181),.UNSPECIFIED.,.F.,.F.,(4,3,3,
3,3,3,3,4),(-337.101751700648,-336.165348291902,-335.167825003202,-334.170301714502,
-333.172778425802,-332.175255137102,-331.177731848402,-330.818566393468),
 .UNSPECIFIED.);
#1340=B_SPLINE_CURVE_WITH_KNOTS('',3,(#54182,#54183,#54184,#54185,#54186,
#54187,#54188,#54189,#54190,#54191,#54192,#54193,#54194,#54195,#54196,#54197,
#54198,#54199,#54200,#54201,#54202,#54203),.UNSPECIFIED.,.F.,.F.,(4,3,3,
3,3,3,3,4),(327.842029482025,328.185161982302,329.182685271002,330.180208559702,
331.177731848402,332.175255137102,333.172778425802,334.125214789205),
 .UNSPECIFIED.);
#1341=B_SPLINE_CURVE_WITH_KNOTS('',3,(#54208,#54209,#54210,#54211,#54212,
#54213,#54214,#54215,#54216,#54217,#54218,#54219,#54220,#54221,#54222,#54223,
#54224,#54225,#54226,#54227,#54228,#54229,#54230,#54231,#54232),
 .UNSPECIFIED.,.F.,.F.,(4,3,3,3,3,3,3,3,4),(-343.384937007828,-343.148011312802,
-342.150488024102,-341.152964735402,-340.155441446702,-339.157918158002,
-338.160394869302,-337.162871580602,-337.101751700648),.UNSPECIFIED.);
#1342=B_SPLINE_CURVE_WITH_KNOTS('',3,(#54233,#54234,#54235,#54236,#54237,
#54238,#54239,#54240,#54241,#54242,#54243,#54244,#54245,#54246,#54247,#54248,
#54249,#54250,#54251,#54252,#54253,#54254,#54255,#54256,#54257),
 .UNSPECIFIED.,.F.,.F.,(4,3,3,3,3,3,3,3,4),(334.125214789205,334.170301714502,
335.167825003202,336.165348291902,337.162871580602,338.160394869302,339.157918158002,
340.155441446702,340.408400096384),.UNSPECIFIED.);
#1343=B_SPLINE_CURVE_WITH_KNOTS('',3,(#54262,#54263,#54264,#54265,#54266,
#54267,#54268,#54269,#54270,#54271,#54272,#54273,#54274,#54275,#54276,#54277,
#54278,#54279,#54280,#54281,#54282,#54283),.UNSPECIFIED.,.F.,.F.,(4,3,3,
3,3,3,3,4),(-349.668122315007,-349.133151045002,-348.135627756302,-347.138104467602,
-346.140581178902,-345.143057890202,-344.145534601502,-343.384937007828),
 .UNSPECIFIED.);
#1344=B_SPLINE_CURVE_WITH_KNOTS('',3,(#54284,#54285,#54286,#54287,#54288,
#54289,#54290,#54291,#54292,#54293,#54294,#54295,#54296,#54297,#54298,#54299,
#54300,#54301,#54302,#54303,#54304,#54305),.UNSPECIFIED.,.F.,.F.,(4,3,3,
3,3,3,3,4),(340.408400096384,341.152964735402,342.150488024102,343.148011312802,
344.145534601502,345.143057890202,346.140581178902,346.691585403564),
 .UNSPECIFIED.);
#1345=B_SPLINE_CURVE_WITH_KNOTS('',3,(#54310,#54311,#54312,#54313,#54314,
#54315,#54316,#54317,#54318,#54319,#54320,#54321,#54322,#54323,#54324,#54325,
#54326,#54327,#54328,#54329,#54330,#54331),.UNSPECIFIED.,.F.,.F.,(4,3,3,
3,3,3,3,4),(-355.951307622187,-355.118290777202,-354.120767488502,-353.123244199802,
-352.125720911102,-351.128197622402,-350.130674333702,-349.668122315007),
 .UNSPECIFIED.);
#1346=B_SPLINE_CURVE_WITH_KNOTS('',3,(#54332,#54333,#54334,#54335,#54336,
#54337,#54338,#54339,#54340,#54341,#54342,#54343,#54344,#54345,#54346,#54347,
#54348,#54349,#54350,#54351,#54352,#54353),.UNSPECIFIED.,.F.,.F.,(4,3,3,
3,3,3,3,4),(346.691585403564,347.138104467602,348.135627756302,349.133151045002,
350.130674333702,351.128197622402,352.125720911102,352.974770710743),
 .UNSPECIFIED.);
#1347=B_SPLINE_CURVE_WITH_KNOTS('',3,(#54358,#54359,#54360,#54361,#54362,
#54363,#54364,#54365,#54366,#54367,#54368,#54369,#54370,#54371,#54372,#54373,
#54374,#54375,#54376,#54377,#54378,#54379,#54380,#54381,#54382),
 .UNSPECIFIED.,.F.,.F.,(4,3,3,3,3,3,3,3,4),(-362.234492929366,-362.100953798102,
-361.103430509402,-360.105907220702,-359.108383932002,-358.110860643302,
-357.113337354602,-356.115814065902,-355.951307622187),.UNSPECIFIED.);
#1348=B_SPLINE_CURVE_WITH_KNOTS('',3,(#54383,#54384,#54385,#54386,#54387,
#54388,#54389,#54390,#54391,#54392,#54393,#54394,#54395,#54396,#54397,#54398,
#54399,#54400,#54401,#54402,#54403,#54404,#54405,#54406,#54407),
 .UNSPECIFIED.,.F.,.F.,(4,3,3,3,3,3,3,3,4),(352.974770710743,353.123244199802,
354.120767488502,355.118290777202,356.115814065902,357.113337354602,358.110860643302,
359.108383932002,359.257956017923),.UNSPECIFIED.);
#1349=B_SPLINE_CURVE_WITH_KNOTS('',3,(#54412,#54413,#54414,#54415,#54416,
#54417,#54418,#54419,#54420,#54421,#54422,#54423,#54424,#54425,#54426,#54427,
#54428,#54429,#54430,#54431,#54432,#54433),.UNSPECIFIED.,.F.,.F.,(4,3,3,
3,3,3,3,4),(-368.517678236546,-368.086093530302,-367.088570241602,-366.091046952902,
-365.093523664202,-364.096000375502,-363.098477086802,-362.234492929366),
 .UNSPECIFIED.);
#1350=B_SPLINE_CURVE_WITH_KNOTS('',3,(#54434,#54435,#54436,#54437,#54438,
#54439,#54440,#54441,#54442,#54443,#54444,#54445,#54446,#54447,#54448,#54449,
#54450,#54451,#54452,#54453,#54454,#54455),.UNSPECIFIED.,.F.,.F.,(4,3,3,
3,3,3,3,4),(359.257956017923,360.105907220702,361.103430509402,362.100953798102,
363.098477086802,364.096000375502,365.093523664202,365.541141325102),
 .UNSPECIFIED.);
#1351=B_SPLINE_CURVE_WITH_KNOTS('',3,(#54460,#54461,#54462,#54463,#54464,
#54465,#54466,#54467,#54468,#54469,#54470,#54471,#54472,#54473,#54474,#54475,
#54476,#54477,#54478,#54479,#54480,#54481),.UNSPECIFIED.,.F.,.F.,(4,3,3,
3,3,3,3,4),(-374.800863543725,-374.071233262502,-373.073709973802,-372.076186685102,
-371.078663396402,-370.081140107702,-369.083616819002,-368.517678236546),
 .UNSPECIFIED.);
#1352=B_SPLINE_CURVE_WITH_KNOTS('',3,(#54482,#54483,#54484,#54485,#54486,
#54487,#54488,#54489,#54490,#54491,#54492,#54493,#54494,#54495,#54496,#54497,
#54498,#54499,#54500,#54501,#54502,#54503),.UNSPECIFIED.,.F.,.F.,(4,3,3,
3,3,3,3,4),(365.541141325102,366.091046952902,367.088570241602,368.086093530302,
369.083616819002,370.081140107702,371.078663396402,371.824326632282),
 .UNSPECIFIED.);
#1353=B_SPLINE_CURVE_WITH_KNOTS('',3,(#54509,#54510,#54511,#54512,#54513,
#54514),.UNSPECIFIED.,.F.,.F.,(4,1,1,4),(386.415896391544,386.683789399021,
387.681312687721,388.606151278594),.UNSPECIFIED.);
#1354=B_SPLINE_CURVE_WITH_KNOTS('',3,(#54517,#54518,#54519,#54520,#54521),
 .UNSPECIFIED.,.F.,.F.,(4,1,4),(386.415896391544,386.868472513736,387.367234158086),
 .UNSPECIFIED.);
#1355=B_SPLINE_CURVE_WITH_KNOTS('',3,(#54526,#54527,#54528,#54529,#54530,
#54531,#54532,#54533,#54534,#54535),.UNSPECIFIED.,.F.,.F.,(4,1,1,1,1,1,
1,4),(380.132711084365,380.698649666821,381.696172955521,382.693696244221,
383.691219532921,384.688742821621,385.686266110321,386.415896391544),
 .UNSPECIFIED.);
#1356=B_SPLINE_CURVE_WITH_KNOTS('',3,(#54536,#54537,#54538,#54539,#54540,
#54541,#54542,#54543,#54544,#54545,#54546),.UNSPECIFIED.,.F.,.F.,(4,1,1,
1,1,1,1,1,4),(380.132711084365,380.384571137186,381.382094425886,382.379617714586,
383.377141003286,384.374664291986,385.372187580686,386.369710869386,386.415896391544),
 .UNSPECIFIED.);
#1357=B_SPLINE_CURVE_WITH_KNOTS('',3,(#54551,#54552,#54553,#54554,#54555,
#54556,#54557,#54558,#54559,#54560),.UNSPECIFIED.,.F.,.F.,(4,1,1,1,1,1,
1,4),(373.849525777185,374.713509934621,375.711033223321,376.708556512021,
377.706079800721,378.703603089421,379.701126378121,380.132711084365),
 .UNSPECIFIED.);
#1358=B_SPLINE_CURVE_WITH_KNOTS('',3,(#54561,#54562,#54563,#54564,#54565,
#54566,#54567,#54568,#54569,#54570),.UNSPECIFIED.,.F.,.F.,(4,1,1,1,1,1,
1,4),(373.849525777185,374.399431404986,375.396954693686,376.394477982386,
377.392001271086,378.389524559786,379.387047848486,380.132711084365),
 .UNSPECIFIED.);
#1359=B_SPLINE_CURVE_WITH_KNOTS('',3,(#54575,#54576,#54577,#54578,#54579,
#54580,#54581,#54582,#54583,#54584,#54585),.UNSPECIFIED.,.F.,.F.,(4,1,1,
1,1,1,1,1,4),(367.566340470006,367.730846913721,368.728370202421,369.725893491121,
370.723416779821,371.720940068521,372.718463357221,373.715986645921,373.849525777185),
 .UNSPECIFIED.);
#1360=B_SPLINE_CURVE_WITH_KNOTS('',3,(#54586,#54587,#54588,#54589,#54590,
#54591,#54592,#54593,#54594,#54595),.UNSPECIFIED.,.F.,.F.,(4,1,1,1,1,1,
1,4),(367.566340470006,368.414291672786,369.411814961486,370.409338250186,
371.406861538886,372.404384827586,373.401908116286,373.849525777185),
 .UNSPECIFIED.);
#1361=B_SPLINE_CURVE_WITH_KNOTS('',3,(#54600,#54601,#54602,#54603,#54604,
#54605,#54606,#54607,#54608,#54609),.UNSPECIFIED.,.F.,.F.,(4,1,1,1,1,1,
1,4),(361.283155162826,361.745707181521,362.743230470221,363.740753758921,
364.738277047621,365.735800336321,366.733323625021,367.566340470006),
 .UNSPECIFIED.);
#1362=B_SPLINE_CURVE_WITH_KNOTS('',3,(#54610,#54611,#54612,#54613,#54614,
#54615,#54616,#54617,#54618,#54619,#54620),.UNSPECIFIED.,.F.,.F.,(4,1,1,
1,1,1,1,1,4),(361.283155162826,361.431628651886,362.429151940586,363.426675229286,
364.424198517986,365.421721806686,366.419245095386,367.416768384086,367.566340470006),
 .UNSPECIFIED.);
#1363=B_SPLINE_CURVE_WITH_KNOTS('',3,(#54625,#54626,#54627,#54628,#54629,
#54630,#54631,#54632,#54633,#54634),.UNSPECIFIED.,.F.,.F.,(4,1,1,1,1,1,
1,4),(354.999969855647,355.760567449321,356.758090738021,357.755614026721,
358.753137315421,359.750660604121,360.748183892821,361.283155162826),
 .UNSPECIFIED.);
#1364=B_SPLINE_CURVE_WITH_KNOTS('',3,(#54635,#54636,#54637,#54638,#54639,
#54640,#54641,#54642,#54643,#54644),.UNSPECIFIED.,.F.,.F.,(4,1,1,1,1,1,
1,4),(354.999969855647,355.446488919686,356.444012208386,357.441535497086,
358.439058785786,359.436582074486,360.434105363186,361.283155162826),
 .UNSPECIFIED.);
#1365=B_SPLINE_CURVE_WITH_KNOTS('',3,(#54649,#54650,#54651,#54652,#54653,
#54654,#54655,#54656,#54657,#54658,#54659),.UNSPECIFIED.,.F.,.F.,(4,1,1,
1,1,1,1,1,4),(348.716784548467,348.777904428421,349.775427717121,350.772951005821,
351.770474294521,352.767997583221,353.765520871921,354.763044160621,354.999969855647),
 .UNSPECIFIED.);
#1366=B_SPLINE_CURVE_WITH_KNOTS('',3,(#54660,#54661,#54662,#54663,#54664,
#54665,#54666,#54667,#54668,#54669),.UNSPECIFIED.,.F.,.F.,(4,1,1,1,1,1,
1,4),(348.716784548467,349.461349187486,350.458872476186,351.456395764886,
352.453919053586,353.451442342286,354.448965630986,354.999969855647),
 .UNSPECIFIED.);
#1367=B_SPLINE_CURVE_WITH_KNOTS('',3,(#54674,#54675,#54676,#54677,#54678,
#54679,#54680,#54681,#54682,#54683),.UNSPECIFIED.,.F.,.F.,(4,1,1,1,1,1,
1,4),(342.433599241287,342.792764696221,343.790287984921,344.787811273621,
345.785334562321,346.782857851021,347.780381139721,348.716784548467),
 .UNSPECIFIED.);
#1368=B_SPLINE_CURVE_WITH_KNOTS('',3,(#54684,#54685,#54686,#54687,#54688,
#54689,#54690,#54691,#54692,#54693,#54694),.UNSPECIFIED.,.F.,.F.,(4,1,1,
1,1,1,1,1,4),(342.433599241287,342.478686166586,343.476209455286,344.473732743986,
345.471256032686,346.468779321386,347.466302610086,348.463825898786,348.716784548467),
 .UNSPECIFIED.);
#1369=B_SPLINE_CURVE_WITH_KNOTS('',3,(#54699,#54700,#54701,#54702,#54703,
#54704,#54705,#54706,#54707,#54708),.UNSPECIFIED.,.F.,.F.,(4,1,1,1,1,1,
1,4),(336.150413934108,336.807624964021,337.805148252721,338.802671541421,
339.800194830121,340.797718118821,341.795241407521,342.433599241287),
 .UNSPECIFIED.);
#1370=B_SPLINE_CURVE_WITH_KNOTS('',3,(#54709,#54710,#54711,#54712,#54713,
#54714,#54715,#54716,#54717,#54718),.UNSPECIFIED.,.F.,.F.,(4,1,1,1,1,1,
1,4),(336.150413934108,336.493546434386,337.491069723086,338.488593011786,
339.486116300486,340.483639589186,341.481162877886,342.433599241287),
 .UNSPECIFIED.);
#1371=B_SPLINE_CURVE_WITH_KNOTS('',3,(#54723,#54724,#54725,#54726,#54727,
#54728,#54729,#54730,#54731,#54732),.UNSPECIFIED.,.F.,.F.,(4,1,1,1,1,1,
1,4),(329.867228626928,330.822485231821,331.820008520521,332.817531809221,
333.815055097921,334.812578386621,335.810101675321,336.150413934108),
 .UNSPECIFIED.);
#1372=B_SPLINE_CURVE_WITH_KNOTS('',3,(#54733,#54734,#54735,#54736,#54737,
#54738,#54739,#54740,#54741,#54742),.UNSPECIFIED.,.F.,.F.,(4,1,1,1,1,1,
1,4),(329.867228626928,330.508406702186,331.505929990886,332.503453279586,
333.500976568286,334.498499856986,335.496023145686,336.150413934108),
 .UNSPECIFIED.);
#1373=B_SPLINE_CURVE_WITH_KNOTS('',3,(#54747,#54748,#54749,#54750,#54751,
#54752,#54753,#54754,#54755,#54756,#54757),.UNSPECIFIED.,.F.,.F.,(4,1,1,
1,1,1,1,1,4),(323.584043319749,323.839822210921,324.837345499621,325.834868788321,
326.832392077021,327.829915365721,328.827438654421,329.824961943121,329.867228626928),
 .UNSPECIFIED.);
#1374=B_SPLINE_CURVE_WITH_KNOTS('',3,(#54758,#54759,#54760,#54761,#54762,
#54763,#54764,#54765,#54766,#54767),.UNSPECIFIED.,.F.,.F.,(4,1,1,1,1,1,
1,4),(323.584043319749,324.523266969986,325.520790258686,326.518313547386,
327.515836836086,328.513360124786,329.510883413486,329.867228626928),
 .UNSPECIFIED.);
#1375=B_SPLINE_CURVE_WITH_KNOTS('',3,(#54772,#54773,#54774,#54775,#54776,
#54777,#54778,#54779,#54780,#54781),.UNSPECIFIED.,.F.,.F.,(4,1,1,1,1,1,
1,4),(317.300858012569,317.854682478721,318.852205767421,319.849729056121,
320.847252344821,321.844775633521,322.842298922221,323.584043319749),
 .UNSPECIFIED.);
#1376=B_SPLINE_CURVE_WITH_KNOTS('',3,(#54782,#54783,#54784,#54785,#54786,
#54787,#54788,#54789,#54790,#54791,#54792),.UNSPECIFIED.,.F.,.F.,(4,1,1,
1,1,1,1,1,4),(317.300858012569,317.540603949086,318.538127237786,319.535650526486,
320.533173815186,321.530697103886,322.528220392586,323.525743681286,323.584043319749),
 .UNSPECIFIED.);
#1377=B_SPLINE_CURVE_WITH_KNOTS('',3,(#54797,#54798,#54799,#54800,#54801,
#54802,#54803,#54804,#54805,#54806),.UNSPECIFIED.,.F.,.F.,(4,1,1,1,1,1,
1,4),(311.01767270539,311.869542746521,312.867066035221,313.864589323921,
314.862112612621,315.859635901321,316.857159190021,317.300858012569),
 .UNSPECIFIED.);
#1378=B_SPLINE_CURVE_WITH_KNOTS('',3,(#54807,#54808,#54809,#54810,#54811,
#54812,#54813,#54814,#54815,#54816),.UNSPECIFIED.,.F.,.F.,(4,1,1,1,1,1,
1,4),(311.01767270539,311.555464216886,312.552987505586,313.550510794286,
314.548034082986,315.545557371686,316.543080660386,317.300858012569),
 .UNSPECIFIED.);
#1379=B_SPLINE_CURVE_WITH_KNOTS('',3,(#54821,#54822,#54823,#54824,#54825,
#54826,#54827,#54828,#54829,#54830,#54831),.UNSPECIFIED.,.F.,.F.,(4,1,1,
1,1,1,1,1,4),(304.73448739821,304.886879725621,305.884403014321,306.881926303021,
307.879449591721,308.876972880421,309.874496169121,310.872019457821,311.01767270539),
 .UNSPECIFIED.);
#1380=B_SPLINE_CURVE_WITH_KNOTS('',3,(#54832,#54833,#54834,#54835,#54836,
#54837,#54838,#54839,#54840,#54841),.UNSPECIFIED.,.F.,.F.,(4,1,1,1,1,1,
1,4),(304.73448739821,305.570324484686,306.567847773386,307.565371062086,
308.562894350786,309.560417639486,310.557940928186,311.01767270539),
 .UNSPECIFIED.);
#1381=B_SPLINE_CURVE_WITH_KNOTS('',3,(#54846,#54847,#54848,#54849,#54850,
#54851,#54852,#54853,#54854,#54855),.UNSPECIFIED.,.F.,.F.,(4,1,1,1,1,1,
1,4),(298.451302091031,298.901739993421,299.899263282121,300.896786570821,
301.894309859521,302.891833148221,303.889356436921,304.73448739821),
 .UNSPECIFIED.);
#1382=B_SPLINE_CURVE_WITH_KNOTS('',3,(#54856,#54857,#54858,#54859,#54860,
#54861,#54862,#54863,#54864,#54865,#54866),.UNSPECIFIED.,.F.,.F.,(4,1,1,
1,1,1,1,1,4),(298.451302091031,298.587661463786,299.585184752486,300.582708041186,
301.580231329886,302.577754618586,303.575277907286,304.572801195986,304.73448739821),
 .UNSPECIFIED.);
#1383=B_SPLINE_CURVE_WITH_KNOTS('',3,(#54871,#54872,#54873,#54874,#54875,
#54876,#54877,#54878,#54879,#54880),.UNSPECIFIED.,.F.,.F.,(4,1,1,1,1,1,
1,4),(292.168116783851,292.916600261221,293.914123549921,294.911646838621,
295.909170127321,296.906693416021,297.904216704721,298.451302091031),
 .UNSPECIFIED.);
#1384=B_SPLINE_CURVE_WITH_KNOTS('',3,(#54881,#54882,#54883,#54884,#54885,
#54886,#54887,#54888,#54889,#54890),.UNSPECIFIED.,.F.,.F.,(4,1,1,1,1,1,
1,4),(292.168116783851,292.602521731586,293.600045020286,294.597568308986,
295.595091597686,296.592614886386,297.590138175086,298.451302091031),
 .UNSPECIFIED.);
#1385=B_SPLINE_CURVE_WITH_KNOTS('',3,(#54895,#54896,#54897,#54898,#54899,
#54900,#54901,#54902,#54903,#54904,#54905),.UNSPECIFIED.,.F.,.F.,(4,1,1,
1,1,1,1,1,4),(285.884931476671,285.933937240321,286.931460529021,287.928983817721,
288.926507106421,289.924030395121,290.921553683821,291.919076972521,292.168116783851),
 .UNSPECIFIED.);
#1386=B_SPLINE_CURVE_WITH_KNOTS('',3,(#54906,#54907,#54908,#54909,#54910,
#54911,#54912,#54913,#54914,#54915),.UNSPECIFIED.,.F.,.F.,(4,1,1,1,1,1,
1,4),(285.884931476671,286.617381999385,287.614905288085,288.612428576785,
289.609951865485,290.607475154186,291.604998442886,292.168116783851),
 .UNSPECIFIED.);
#1387=B_SPLINE_CURVE_WITH_KNOTS('',3,(#54920,#54921,#54922,#54923,#54924,
#54925,#54926,#54927,#54928,#54929),.UNSPECIFIED.,.F.,.F.,(4,1,1,1,1,1,
1,4),(279.601746169492,279.948797508121,280.946320796821,281.943844085521,
282.941367374221,283.938890662921,284.936413951621,285.884931476671),
 .UNSPECIFIED.);
#1388=B_SPLINE_CURVE_WITH_KNOTS('',3,(#54930,#54931,#54932,#54933,#54934,
#54935,#54936,#54937,#54938,#54939,#54940),.UNSPECIFIED.,.F.,.F.,(4,1,1,
1,1,1,1,1,4),(279.601746169492,279.634718978485,280.632242267185,281.629765555885,
282.627288844585,283.624812133285,284.622335421985,285.619858710685,285.884931476671),
 .UNSPECIFIED.);
#1389=B_SPLINE_CURVE_WITH_KNOTS('',3,(#54945,#54946,#54947,#54948,#54949,
#54950,#54951,#54952,#54953,#54954),.UNSPECIFIED.,.F.,.F.,(4,1,1,1,1,1,
1,4),(273.318560862312,273.963657775921,274.961181064621,275.958704353321,
276.956227642021,277.953750930721,278.951274219421,279.601746169492),
 .UNSPECIFIED.);
#1390=B_SPLINE_CURVE_WITH_KNOTS('',3,(#54955,#54956,#54957,#54958,#54959,
#54960,#54961,#54962,#54963,#54964),.UNSPECIFIED.,.F.,.F.,(4,1,1,1,1,1,
1,4),(273.318560862312,273.649579246285,274.647102534985,275.644625823685,
276.642149112385,277.639672401085,278.637195689785,279.601746169492),
 .UNSPECIFIED.);
#1391=B_SPLINE_CURVE_WITH_KNOTS('',3,(#54969,#54970,#54971,#54972,#54973,
#54974,#54975,#54976,#54977,#54978),.UNSPECIFIED.,.F.,.F.,(4,1,1,1,1,1,
1,4),(267.035375555133,267.97851804372,268.97604133242,269.973564621121,
270.971087909821,271.968611198521,272.966134487221,273.318560862312),
 .UNSPECIFIED.);
#1392=B_SPLINE_CURVE_WITH_KNOTS('',3,(#54979,#54980,#54981,#54982,#54983,
#54984,#54985,#54986,#54987,#54988),.UNSPECIFIED.,.F.,.F.,(4,1,1,1,1,1,
1,4),(267.035375555133,267.664439514085,268.661962802785,269.659486091485,
270.657009380185,271.654532668885,272.652055957585,273.318560862312),
 .UNSPECIFIED.);
#1393=B_SPLINE_CURVE_WITH_KNOTS('',3,(#54993,#54994,#54995,#54996,#54997,
#54998,#54999,#55000,#55001,#55002,#55003),.UNSPECIFIED.,.F.,.F.,(4,1,1,
1,1,1,1,1,4),(260.752190247953,260.99585502282,261.99337831152,262.99090160022,
263.98842488892,264.98594817762,265.983471466321,266.980994755021,267.035375555133),
 .UNSPECIFIED.);
#1394=B_SPLINE_CURVE_WITH_KNOTS('',3,(#55004,#55005,#55006,#55007,#55008,
#55009,#55010,#55011,#55012,#55013),.UNSPECIFIED.,.F.,.F.,(4,1,1,1,1,1,
1,4),(260.752190247953,261.679299781885,262.676823070585,263.674346359285,
264.671869647985,265.669392936685,266.666916225385,267.035375555133),
 .UNSPECIFIED.);
#1395=B_SPLINE_CURVE_WITH_KNOTS('',3,(#55018,#55019,#55020,#55021,#55022,
#55023,#55024,#55025,#55026,#55027),.UNSPECIFIED.,.F.,.F.,(4,1,1,1,1,1,
1,4),(254.469004940774,255.01071529062,256.00823857932,257.00576186802,
258.00328515672,259.00080844542,259.99833173412,260.752190247953),
 .UNSPECIFIED.);
#1396=B_SPLINE_CURVE_WITH_KNOTS('',3,(#55028,#55029,#55030,#55031,#55032,
#55033,#55034,#55035,#55036,#55037,#55038),.UNSPECIFIED.,.F.,.F.,(4,1,1,
1,1,1,1,1,4),(254.469004940774,254.696636760985,255.694160049685,256.691683338385,
257.689206627085,258.686729915785,259.684253204485,260.681776493185,260.752190247953),
 .UNSPECIFIED.);
#1397=B_SPLINE_CURVE_WITH_KNOTS('',3,(#55043,#55044,#55045,#55046,#55047,
#55048,#55049,#55050,#55051,#55052),.UNSPECIFIED.,.F.,.F.,(4,1,1,1,1,1,
1,4),(248.185819633594,249.02557555842,250.02309884712,251.02062213582,
252.01814542452,253.01566871322,254.01319200192,254.469004940774),
 .UNSPECIFIED.);
#1398=B_SPLINE_CURVE_WITH_KNOTS('',3,(#55053,#55054,#55055,#55056,#55057,
#55058,#55059,#55060,#55061,#55062),.UNSPECIFIED.,.F.,.F.,(4,1,1,1,1,1,
1,4),(248.185819633594,248.711497028785,249.709020317485,250.706543606185,
251.704066894885,252.701590183585,253.699113472285,254.469004940774),
 .UNSPECIFIED.);
#1399=B_SPLINE_CURVE_WITH_KNOTS('',3,(#55067,#55068,#55069,#55070,#55071,
#55072,#55073,#55074,#55075,#55076,#55077),.UNSPECIFIED.,.F.,.F.,(4,1,1,
1,1,1,1,1,4),(241.902634326414,242.04291253752,243.04043582622,244.03795911492,
245.03548240362,246.03300569232,247.03052898102,248.02805226972,248.185819633594),
 .UNSPECIFIED.);
#1400=B_SPLINE_CURVE_WITH_KNOTS('',3,(#55078,#55079,#55080,#55081,#55082,
#55083,#55084,#55085,#55086,#55087),.UNSPECIFIED.,.F.,.F.,(4,1,1,1,1,1,
1,4),(241.902634326414,242.726357296585,243.723880585285,244.721403873985,
245.718927162685,246.716450451385,247.713973740085,248.185819633594),
 .UNSPECIFIED.);
#1401=B_SPLINE_CURVE_WITH_KNOTS('',3,(#55092,#55093,#55094,#55095,#55096,
#55097,#55098,#55099,#55100,#55101),.UNSPECIFIED.,.F.,.F.,(4,1,1,1,1,1,
1,4),(235.619449019235,236.05777280532,237.05529609402,238.05281938272,
239.05034267142,240.04786596012,241.04538924882,241.902634326414),
 .UNSPECIFIED.);
#1402=B_SPLINE_CURVE_WITH_KNOTS('',3,(#55102,#55103,#55104,#55105,#55106,
#55107,#55108,#55109,#55110,#55111,#55112),.UNSPECIFIED.,.F.,.F.,(4,1,1,
1,1,1,1,1,4),(235.619449019235,235.743694275685,236.741217564385,237.738740853085,
238.736264141785,239.733787430485,240.731310719185,241.728834007885,241.902634326414),
 .UNSPECIFIED.);
#1403=B_SPLINE_CURVE_WITH_KNOTS('',3,(#55117,#55118,#55119,#55120,#55121,
#55122,#55123,#55124,#55125,#55126),.UNSPECIFIED.,.F.,.F.,(4,1,1,1,1,1,
1,4),(229.336263712055,230.07263307312,231.07015636182,232.06767965052,
233.06520293922,234.06272622792,235.06024951662,235.619449019235),
 .UNSPECIFIED.);
#1404=B_SPLINE_CURVE_WITH_KNOTS('',3,(#55127,#55128,#55129,#55130,#55131,
#55132,#55133,#55134,#55135,#55136),.UNSPECIFIED.,.F.,.F.,(4,1,1,1,1,1,
1,4),(229.336263712055,229.758554543485,230.756077832185,231.753601120885,
232.751124409585,233.748647698285,234.746170986985,235.619449019235),
 .UNSPECIFIED.);
#1405=B_SPLINE_CURVE_WITH_KNOTS('',3,(#55141,#55142,#55143,#55144,#55145,
#55146,#55147,#55148,#55149,#55150,#55151),.UNSPECIFIED.,.F.,.F.,(4,1,1,
1,1,1,1,1,4),(223.053078404876,223.08997005222,224.08749334092,225.08501662962,
226.08253991832,227.08006320702,228.07758649572,229.07510978442,229.336263712055),
 .UNSPECIFIED.);
#1406=B_SPLINE_CURVE_WITH_KNOTS('',3,(#55152,#55153,#55154,#55155,#55156,
#55157,#55158,#55159,#55160,#55161),.UNSPECIFIED.,.F.,.F.,(4,1,1,1,1,1,
1,4),(223.053078404876,223.773414811285,224.770938099985,225.768461388685,
226.765984677385,227.763507966085,228.761031254785,229.336263712055),
 .UNSPECIFIED.);
#1407=B_SPLINE_CURVE_WITH_KNOTS('',3,(#55166,#55167,#55168,#55169,#55170,
#55171,#55172,#55173,#55174,#55175),.UNSPECIFIED.,.F.,.F.,(4,1,1,1,1,1,
1,4),(216.769893097696,217.10483032002,218.10235360872,219.09987689742,
220.09740018612,221.09492347482,222.09244676352,223.053078404876),
 .UNSPECIFIED.);
#1408=B_SPLINE_CURVE_WITH_KNOTS('',3,(#55176,#55177,#55178,#55179,#55180,
#55181,#55182,#55183,#55184,#55185,#55186),.UNSPECIFIED.,.F.,.F.,(4,1,1,
1,1,1,1,1,4),(216.769893097696,216.790751790385,217.788275079085,218.785798367785,
219.783321656485,220.780844945185,221.778368233885,222.775891522585,223.053078404876),
 .UNSPECIFIED.);
#1409=B_SPLINE_CURVE_WITH_KNOTS('',3,(#55191,#55192,#55193,#55194,#55195,
#55196,#55197,#55198,#55199,#55200),.UNSPECIFIED.,.F.,.F.,(4,1,1,1,1,1,
1,4),(210.486707790517,211.11969058782,212.11721387652,213.11473716522,
214.11226045392,215.10978374262,216.10730703132,216.769893097696),
 .UNSPECIFIED.);
#1410=B_SPLINE_CURVE_WITH_KNOTS('',3,(#55201,#55202,#55203,#55204,#55205,
#55206,#55207,#55208,#55209,#55210),.UNSPECIFIED.,.F.,.F.,(4,1,1,1,1,1,
1,4),(210.486707790517,210.805612058185,211.803135346885,212.800658635585,
213.798181924285,214.795705212985,215.793228501685,216.769893097696),
 .UNSPECIFIED.);
#1411=B_SPLINE_CURVE_WITH_KNOTS('',3,(#55215,#55216,#55217,#55218,#55219,
#55220,#55221,#55222,#55223,#55224),.UNSPECIFIED.,.F.,.F.,(4,1,1,1,1,1,
1,4),(204.203522483337,205.13455085562,206.13207414432,207.12959743302,
208.12712072172,209.12464401042,210.12216729912,210.486707790517),
 .UNSPECIFIED.);
#1412=B_SPLINE_CURVE_WITH_KNOTS('',3,(#55225,#55226,#55227,#55228,#55229,
#55230,#55231,#55232,#55233,#55234),.UNSPECIFIED.,.F.,.F.,(4,1,1,1,1,1,
1,4),(204.203522483337,204.820472325985,205.817995614685,206.815518903385,
207.813042192085,208.810565480785,209.808088769485,210.486707790517),
 .UNSPECIFIED.);
#1413=B_SPLINE_CURVE_WITH_KNOTS('',3,(#55239,#55240,#55241,#55242,#55243,
#55244,#55245,#55246,#55247,#55248,#55249),.UNSPECIFIED.,.F.,.F.,(4,1,1,
1,1,1,1,1,4),(197.920337176158,198.15188783472,199.14941112342,200.14693441212,
201.14445770082,202.14198098952,203.13950427822,204.13702756692,204.203522483337),
 .UNSPECIFIED.);
#1414=B_SPLINE_CURVE_WITH_KNOTS('',3,(#55250,#55251,#55252,#55253,#55254,
#55255,#55256,#55257,#55258,#55259),.UNSPECIFIED.,.F.,.F.,(4,1,1,1,1,1,
1,4),(197.920337176158,198.835332593785,199.832855882485,200.830379171185,
201.827902459885,202.825425748585,203.822949037285,204.203522483337),
 .UNSPECIFIED.);
#1415=B_SPLINE_CURVE_WITH_KNOTS('',3,(#55264,#55265,#55266,#55267,#55268,
#55269,#55270,#55271,#55272,#55273),.UNSPECIFIED.,.F.,.F.,(4,1,1,1,1,1,
1,4),(191.637151868978,192.16674810252,193.16427139122,194.16179467992,
195.15931796862,196.15684125732,197.15436454602,197.920337176158),
 .UNSPECIFIED.);
#1416=B_SPLINE_CURVE_WITH_KNOTS('',3,(#55274,#55275,#55276,#55277,#55278,
#55279,#55280,#55281,#55282,#55283,#55284),.UNSPECIFIED.,.F.,.F.,(4,1,1,
1,1,1,1,1,4),(191.637151868978,191.852669572885,192.850192861585,193.847716150285,
194.845239438985,195.842762727685,196.840286016385,197.837809305085,197.920337176158),
 .UNSPECIFIED.);
#1417=B_SPLINE_CURVE_WITH_KNOTS('',3,(#55289,#55290,#55291,#55292,#55293,
#55294,#55295,#55296,#55297,#55298),.UNSPECIFIED.,.F.,.F.,(4,1,1,1,1,1,
1,4),(185.353966561798,186.18160837032,187.17913165902,188.17665494772,
189.17417823642,190.17170152512,191.16922481382,191.637151868978),
 .UNSPECIFIED.);
#1418=B_SPLINE_CURVE_WITH_KNOTS('',3,(#55299,#55300,#55301,#55302,#55303,
#55304,#55305,#55306,#55307,#55308),.UNSPECIFIED.,.F.,.F.,(4,1,1,1,1,1,
1,4),(185.353966561798,185.867529840685,186.865053129385,187.862576418085,
188.860099706785,189.857622995485,190.855146284185,191.637151868978),
 .UNSPECIFIED.);
#1419=B_SPLINE_CURVE_WITH_KNOTS('',3,(#55313,#55314,#55315,#55316,#55317,
#55318,#55319,#55320,#55321,#55322,#55323),.UNSPECIFIED.,.F.,.F.,(4,1,1,
1,1,1,1,1,4),(179.070781254619,179.19894534942,180.19646863812,181.19399192682,
182.19151521552,183.18903850422,184.18656179292,185.18408508162,185.353966561798),
 .UNSPECIFIED.);
#1420=B_SPLINE_CURVE_WITH_KNOTS('',3,(#55324,#55325,#55326,#55327,#55328,
#55329,#55330,#55331,#55332,#55333),.UNSPECIFIED.,.F.,.F.,(4,1,1,1,1,1,
1,4),(179.070781254619,179.882390108485,180.879913397185,181.877436685885,
182.874959974585,183.872483263285,184.870006551985,185.353966561798),
 .UNSPECIFIED.);
#1421=B_SPLINE_CURVE_WITH_KNOTS('',3,(#55338,#55339,#55340,#55341,#55342,
#55343,#55344,#55345,#55346,#55347),.UNSPECIFIED.,.F.,.F.,(4,1,1,1,1,1,
1,4),(172.787595947439,173.21380561722,174.21132890592,175.20885219462,
176.20637548332,177.20389877202,178.20142206072,179.070781254619),
 .UNSPECIFIED.);
#1422=B_SPLINE_CURVE_WITH_KNOTS('',3,(#55348,#55349,#55350,#55351,#55352,
#55353,#55354,#55355,#55356,#55357,#55358),.UNSPECIFIED.,.F.,.F.,(4,1,1,
1,1,1,1,1,4),(172.787595947439,172.899727087585,173.897250376285,174.894773664985,
175.892296953685,176.889820242385,177.887343531085,178.884866819785,179.070781254619),
 .UNSPECIFIED.);
#1423=B_SPLINE_CURVE_WITH_KNOTS('',3,(#55363,#55364,#55365,#55366,#55367,
#55368,#55369,#55370,#55371,#55372),.UNSPECIFIED.,.F.,.F.,(4,1,1,1,1,1,
1,4),(166.50441064026,167.22866588502,168.22618917372,169.22371246242,170.22123575112,
171.21875903982,172.21628232852,172.787595947439),.UNSPECIFIED.);
#1424=B_SPLINE_CURVE_WITH_KNOTS('',3,(#55373,#55374,#55375,#55376,#55377,
#55378,#55379,#55380,#55381,#55382),.UNSPECIFIED.,.F.,.F.,(4,1,1,1,1,1,
1,4),(166.50441064026,166.914587355385,167.912110644085,168.909633932785,
169.907157221485,170.904680510185,171.902203798885,172.787595947439),
 .UNSPECIFIED.);
#1425=B_SPLINE_CURVE_WITH_KNOTS('',3,(#55387,#55388,#55389,#55390,#55391,
#55392,#55393,#55394,#55395,#55396,#55397),.UNSPECIFIED.,.F.,.F.,(4,1,1,
1,1,1,1,1,4),(160.22122533308,160.24600286412,161.24352615282,162.24104944152,
163.23857273022,164.23609601892,165.23361930762,166.23114259632,166.50441064026),
 .UNSPECIFIED.);
#1426=B_SPLINE_CURVE_WITH_KNOTS('',3,(#55398,#55399,#55400,#55401,#55402,
#55403,#55404,#55405,#55406,#55407),.UNSPECIFIED.,.F.,.F.,(4,1,1,1,1,1,
1,4),(160.22122533308,160.929447623185,161.926970911885,162.924494200585,
163.922017489285,164.919540777985,165.917064066685,166.50441064026),
 .UNSPECIFIED.);
#1427=B_SPLINE_CURVE_WITH_KNOTS('',3,(#55412,#55413,#55414,#55415,#55416,
#55417,#55418,#55419,#55420,#55421),.UNSPECIFIED.,.F.,.F.,(4,1,1,1,1,1,
1,4),(153.938040025901,154.26086313192,155.25838642062,156.25590970932,
157.25343299802,158.25095628672,159.24847957542,160.22122533308),
 .UNSPECIFIED.);
#1428=B_SPLINE_CURVE_WITH_KNOTS('',3,(#55422,#55423,#55424,#55425,#55426,
#55427,#55428,#55429,#55430,#55431,#55432),.UNSPECIFIED.,.F.,.F.,(4,1,1,
1,1,1,1,1,4),(153.938040025901,153.946784602285,154.944307890985,155.941831179685,
156.939354468385,157.936877757085,158.934401045785,159.931924334485,160.22122533308),
 .UNSPECIFIED.);
#1429=B_SPLINE_CURVE_WITH_KNOTS('',3,(#55437,#55438,#55439,#55440,#55441,
#55442,#55443,#55444,#55445,#55446),.UNSPECIFIED.,.F.,.F.,(4,1,1,1,1,1,
1,4),(147.654854718721,148.27572339972,149.27324668842,150.27076997712,
151.26829326582,152.26581655452,153.26333984322,153.938040025901),
 .UNSPECIFIED.);
#1430=B_SPLINE_CURVE_WITH_KNOTS('',3,(#55447,#55448,#55449,#55450,#55451,
#55452,#55453,#55454,#55455,#55456),.UNSPECIFIED.,.F.,.F.,(4,1,1,1,1,1,
1,4),(147.654854718721,147.961644870085,148.959168158785,149.956691447485,
150.954214736185,151.951738024885,152.949261313585,153.938040025901),
 .UNSPECIFIED.);
#1431=B_SPLINE_CURVE_WITH_KNOTS('',3,(#55461,#55462,#55463,#55464,#55465,
#55466,#55467,#55468,#55469,#55470),.UNSPECIFIED.,.F.,.F.,(4,1,1,1,1,1,
1,4),(141.371669411541,142.29058366752,143.28810695622,144.28563024492,
145.28315353362,146.28067682232,147.27820011102,147.654854718721),
 .UNSPECIFIED.);
#1432=B_SPLINE_CURVE_WITH_KNOTS('',3,(#55471,#55472,#55473,#55474,#55475,
#55476,#55477,#55478,#55479,#55480),.UNSPECIFIED.,.F.,.F.,(4,1,1,1,1,1,
1,4),(141.371669411541,141.976505137885,142.974028426585,143.971551715285,
144.969075003985,145.966598292685,146.964121581385,147.654854718721),
 .UNSPECIFIED.);
#1433=B_SPLINE_CURVE_WITH_KNOTS('',3,(#55485,#55486,#55487,#55488,#55489,
#55490,#55491,#55492,#55493,#55494,#55495),.UNSPECIFIED.,.F.,.F.,(4,1,1,
1,1,1,1,1,4),(135.088484104362,135.30792064662,136.30544393532,137.30296722402,
138.30049051272,139.29801380142,140.29553709012,141.29306037882,141.371669411541),
 .UNSPECIFIED.);
#1434=B_SPLINE_CURVE_WITH_KNOTS('',3,(#55496,#55497,#55498,#55499,#55500,
#55501,#55502,#55503,#55504,#55505),.UNSPECIFIED.,.F.,.F.,(4,1,1,1,1,1,
1,4),(135.088484104362,135.991365405685,136.988888694385,137.986411983085,
138.983935271785,139.981458560485,140.978981849185,141.371669411541),
 .UNSPECIFIED.);
#1435=B_SPLINE_CURVE_WITH_KNOTS('',3,(#55510,#55511,#55512,#55513,#55514,
#55515,#55516,#55517,#55518,#55519),.UNSPECIFIED.,.F.,.F.,(4,1,1,1,1,1,
1,4),(128.805298797182,129.32278091442,130.32030420312,131.31782749182,
132.31535078052,133.31287406922,134.31039735792,135.088484104362),
 .UNSPECIFIED.);
#1436=B_SPLINE_CURVE_WITH_KNOTS('',3,(#55520,#55521,#55522,#55523,#55524,
#55525,#55526,#55527,#55528,#55529,#55530),.UNSPECIFIED.,.F.,.F.,(4,1,1,
1,1,1,1,1,4),(128.805298797182,129.008702384785,130.006225673485,131.003748962185,
132.001272250885,132.998795539585,133.996318828285,134.993842116985,135.088484104362),
 .UNSPECIFIED.);
#1437=B_SPLINE_CURVE_WITH_KNOTS('',3,(#55535,#55536,#55537,#55538,#55539,
#55540,#55541,#55542,#55543,#55544),.UNSPECIFIED.,.F.,.F.,(4,1,1,1,1,1,
1,4),(122.522113490003,123.33764118222,124.33516447092,125.33268775962,
126.33021104832,127.32773433702,128.32525762572,128.805298797182),
 .UNSPECIFIED.);
#1438=B_SPLINE_CURVE_WITH_KNOTS('',3,(#55545,#55546,#55547,#55548,#55549,
#55550,#55551,#55552,#55553,#55554),.UNSPECIFIED.,.F.,.F.,(4,1,1,1,1,1,
1,4),(122.522113490003,123.023562652585,124.021085941285,125.018609229985,
126.016132518685,127.013655807385,128.011179096085,128.805298797182),
 .UNSPECIFIED.);
#1439=B_SPLINE_CURVE_WITH_KNOTS('',3,(#55559,#55560,#55561,#55562,#55563,
#55564,#55565,#55566,#55567,#55568,#55569),.UNSPECIFIED.,.F.,.F.,(4,1,1,
1,1,1,1,1,4),(116.238928182823,116.35497816132,117.35250145002,118.35002473872,
119.34754802742,120.34507131612,121.34259460482,122.34011789352,122.522113490003),
 .UNSPECIFIED.);
#1440=B_SPLINE_CURVE_WITH_KNOTS('',3,(#55570,#55571,#55572,#55573,#55574,
#55575,#55576,#55577,#55578,#55579),.UNSPECIFIED.,.F.,.F.,(4,1,1,1,1,1,
1,4),(116.238928182823,117.038422920385,118.035946209085,119.033469497785,
120.030992786485,121.028516075185,122.026039363885,122.522113490003),
 .UNSPECIFIED.);
#1441=B_SPLINE_CURVE_WITH_KNOTS('',3,(#55584,#55585,#55586,#55587,#55588,
#55589,#55590,#55591,#55592,#55593),.UNSPECIFIED.,.F.,.F.,(4,1,1,1,1,1,
1,4),(109.955742875644,110.36983842912,111.36736171782,112.36488500652,
113.36240829522,114.35993158392,115.35745487262,116.238928182823),
 .UNSPECIFIED.);
#1442=B_SPLINE_CURVE_WITH_KNOTS('',3,(#55594,#55595,#55596,#55597,#55598,
#55599,#55600,#55601,#55602,#55603,#55604),.UNSPECIFIED.,.F.,.F.,(4,1,1,
1,1,1,1,1,4),(109.955742875644,110.055759899484,111.053283188184,112.050806476884,
113.048329765584,114.045853054284,115.043376342985,116.040899631685,116.238928182823),
 .UNSPECIFIED.);
#1443=B_SPLINE_CURVE_WITH_KNOTS('',3,(#55609,#55610,#55611,#55612,#55613,
#55614,#55615,#55616,#55617,#55618),.UNSPECIFIED.,.F.,.F.,(4,1,1,1,1,1,
1,4),(103.672557568464,104.38469869692,105.38222198562,106.37974527432,
107.37726856302,108.37479185172,109.37231514042,109.955742875644),
 .UNSPECIFIED.);
#1444=B_SPLINE_CURVE_WITH_KNOTS('',3,(#55619,#55620,#55621,#55622,#55623,
#55624,#55625,#55626,#55627,#55628),.UNSPECIFIED.,.F.,.F.,(4,1,1,1,1,1,
1,4),(103.672557568464,104.070620167284,105.068143455984,106.065666744684,
107.063190033384,108.060713322084,109.058236610784,109.955742875644),
 .UNSPECIFIED.);
#1445=B_SPLINE_CURVE_WITH_KNOTS('',3,(#55633,#55634,#55635,#55636,#55637,
#55638,#55639,#55640,#55641,#55642,#55643),.UNSPECIFIED.,.F.,.F.,(4,1,1,
1,1,1,1,1,4),(97.3893722612843,97.4020356760196,98.3995589647196,99.3970822534196,
100.39460554212,101.39212883082,102.38965211952,103.38717540822,103.672557568464),
 .UNSPECIFIED.);
#1446=B_SPLINE_CURVE_WITH_KNOTS('',3,(#55644,#55645,#55646,#55647,#55648,
#55649,#55650,#55651,#55652,#55653),.UNSPECIFIED.,.F.,.F.,(4,1,1,1,1,1,
1,4),(97.3893722612844,98.0854804350844,99.0830037237844,100.080527012484,
101.078050301184,102.075573589884,103.073096878584,103.672557568464),
 .UNSPECIFIED.);
#1447=B_SPLINE_CURVE_WITH_KNOTS('',3,(#55658,#55659,#55660,#55661,#55662,
#55663,#55664,#55665,#55666,#55667),.UNSPECIFIED.,.F.,.F.,(4,1,1,1,1,1,
1,4),(91.1061869541047,91.4168959438195,92.4144192325195,93.4119425212196,
94.4094658099196,95.4069890986196,96.4045123873196,97.3893722612843),
 .UNSPECIFIED.);
#1448=B_SPLINE_CURVE_WITH_KNOTS('',3,(#55668,#55669,#55670,#55671,#55672,
#55673,#55674,#55675,#55676,#55677),.UNSPECIFIED.,.F.,.F.,(4,1,1,1,1,1,
1,4),(91.1061869541048,92.1003407028844,93.0978639915844,94.0953872802844,
95.0929105689844,96.0904338576844,97.0879571463844,97.3893722612844),
 .UNSPECIFIED.);
#1449=B_SPLINE_CURVE_WITH_KNOTS('',3,(#55682,#55683,#55684,#55685,#55686,
#55687,#55688,#55689,#55690,#55691),.UNSPECIFIED.,.F.,.F.,(4,1,1,1,1,1,
1,4),(84.8230016469251,85.4317562116195,86.4292795003195,87.4268027890195,
88.4243260777195,89.4218493664195,90.4193726551195,91.1061869541047),
 .UNSPECIFIED.);
#1450=B_SPLINE_CURVE_WITH_KNOTS('',3,(#55692,#55693,#55694,#55695,#55696,
#55697,#55698,#55699,#55700,#55701,#55702),.UNSPECIFIED.,.F.,.F.,(4,1,1,
1,1,1,1,1,4),(84.8230016469252,85.1176776819843,86.1152009706843,87.1127242593844,
88.1102475480844,89.1077708367844,90.1052941254844,91.1028174141844,91.1061869541048),
 .UNSPECIFIED.);
#1451=B_SPLINE_CURVE_WITH_KNOTS('',3,(#55707,#55708,#55709,#55710,#55711,
#55712,#55713,#55714,#55715,#55716),.UNSPECIFIED.,.F.,.F.,(4,1,1,1,1,1,
1,4),(78.5398163397455,79.4466164794195,80.4441397681195,81.4416630568195,
82.4391863455195,83.4367096342195,84.4342329229195,84.8230016469251),
 .UNSPECIFIED.);
#1452=B_SPLINE_CURVE_WITH_KNOTS('',3,(#55717,#55718,#55719,#55720,#55721,
#55722,#55723,#55724,#55725,#55726),.UNSPECIFIED.,.F.,.F.,(4,1,1,1,1,1,
1,4),(78.5398163397456,79.1325379497843,80.1300612384843,81.1275845271843,
82.1251078158843,83.1226311045843,84.1201543932843,84.8230016469252),
 .UNSPECIFIED.);
#1453=B_SPLINE_CURVE_WITH_KNOTS('',3,(#55731,#55732,#55733,#55734,#55735,
#55736,#55737,#55738,#55739,#55740,#55741),.UNSPECIFIED.,.F.,.F.,(4,1,1,
1,1,1,1,1,4),(72.2566310325659,72.4639534585194,73.4614767472195,74.4590000359194,
75.4565233246195,76.4540466133195,77.4515699020195,78.4490931907195,78.5398163397455),
 .UNSPECIFIED.);
#1454=B_SPLINE_CURVE_WITH_KNOTS('',3,(#55742,#55743,#55744,#55745,#55746,
#55747,#55748,#55749,#55750,#55751),.UNSPECIFIED.,.F.,.F.,(4,1,1,1,1,1,
1,4),(72.256631032566,73.1473982175843,74.1449215062843,75.1424447949843,
76.1399680836843,77.1374913723843,78.1350146610843,78.5398163397456),
 .UNSPECIFIED.);
#1455=B_SPLINE_CURVE_WITH_KNOTS('',3,(#55756,#55757,#55758,#55759,#55760,
#55761,#55762,#55763,#55764,#55765),.UNSPECIFIED.,.F.,.F.,(4,1,1,1,1,1,
1,4),(65.9734457253863,66.4788137263194,67.4763370150194,68.4738603037194,
69.4713835924194,70.4689068811194,71.4664301698194,72.2566310325659),
 .UNSPECIFIED.);
#1456=B_SPLINE_CURVE_WITH_KNOTS('',3,(#55766,#55767,#55768,#55769,#55770,
#55771,#55772,#55773,#55774,#55775,#55776),.UNSPECIFIED.,.F.,.F.,(4,1,1,
1,1,1,1,1,4),(65.9734457253864,66.1647351966842,67.1622584853842,68.1597817740843,
69.1573050627842,70.1548283514843,71.1523516401843,72.1498749288843,72.256631032566),
 .UNSPECIFIED.);
#1457=B_SPLINE_CURVE_WITH_KNOTS('',3,(#55781,#55782,#55783,#55784,#55785,
#55786,#55787,#55788,#55789,#55790),.UNSPECIFIED.,.F.,.F.,(4,1,1,1,1,1,
1,4),(59.6902604182067,60.4936739941194,61.4911972828194,62.4887205715194,
63.4862438602194,64.4837671489194,65.4812904376194,65.9734457253863),
 .UNSPECIFIED.);
#1458=B_SPLINE_CURVE_WITH_KNOTS('',3,(#55791,#55792,#55793,#55794,#55795,
#55796,#55797,#55798,#55799,#55800),.UNSPECIFIED.,.F.,.F.,(4,1,1,1,1,1,
1,4),(59.6902604182069,60.1795954644842,61.1771187531842,62.1746420418842,
63.1721653305842,64.1696886192842,65.1672119079842,65.9734457253864),
 .UNSPECIFIED.);
#1459=B_SPLINE_CURVE_WITH_KNOTS('',3,(#55805,#55806,#55807,#55808,#55809,
#55810,#55811,#55812,#55813,#55814,#55815),.UNSPECIFIED.,.F.,.F.,(4,1,1,
1,1,1,1,1,4),(53.4070751110272,53.5110109732193,54.5085342619193,55.5060575506193,
56.5035808393194,57.5011041280194,58.4986274167194,59.4961507054194,59.6902604182067),
 .UNSPECIFIED.);
#1460=B_SPLINE_CURVE_WITH_KNOTS('',3,(#55816,#55817,#55818,#55819,#55820,
#55821,#55822,#55823,#55824,#55825),.UNSPECIFIED.,.F.,.F.,(4,1,1,1,1,1,
1,4),(53.4070751110273,54.1944557322842,55.1919790209842,56.1895023096842,
57.1870255983842,58.1845488870842,59.1820721757842,59.6902604182069),
 .UNSPECIFIED.);
#1461=B_SPLINE_CURVE_WITH_KNOTS('',3,(#55830,#55831,#55832,#55833,#55834,
#55835,#55836,#55837,#55838,#55839),.UNSPECIFIED.,.F.,.F.,(4,1,1,1,1,1,
1,4),(47.1238898038476,47.5258712410193,48.5233945297193,49.5209178184193,
50.5184411071193,51.5159643958193,52.5134876845193,53.4070751110272),
 .UNSPECIFIED.);
#1462=B_SPLINE_CURVE_WITH_KNOTS('',3,(#55840,#55841,#55842,#55843,#55844,
#55845,#55846,#55847,#55848,#55849,#55850),.UNSPECIFIED.,.F.,.F.,(4,1,1,
1,1,1,1,1,4),(47.1238898038477,47.2117927113841,48.2093160000841,49.2068392887841,
50.2043625774841,51.2018858661842,52.1994091548842,53.1969324435842,53.4070751110273),
 .UNSPECIFIED.);
#1463=B_SPLINE_CURVE_WITH_KNOTS('',3,(#55855,#55856,#55857,#55858,#55859,
#55860,#55861,#55862,#55863,#55864),.UNSPECIFIED.,.F.,.F.,(4,1,1,1,1,1,
1,4),(40.840704496668,41.5407315088193,42.5382547975193,43.5357780862193,
44.5333013749193,45.5308246636193,46.5283479523193,47.1238898038476),
 .UNSPECIFIED.);
#1464=B_SPLINE_CURVE_WITH_KNOTS('',3,(#55865,#55866,#55867,#55868,#55869,
#55870,#55871,#55872,#55873,#55874),.UNSPECIFIED.,.F.,.F.,(4,1,1,1,1,1,
1,4),(40.8407044966681,41.2266529791841,42.2241762678841,43.2216995565841,
44.2192228452841,45.2167461339841,46.2142694226841,47.1238898038477),
 .UNSPECIFIED.);
#1465=B_SPLINE_CURVE_WITH_KNOTS('',3,(#55879,#55880,#55881,#55882,#55883,
#55884,#55885,#55886,#55887,#55888,#55889),.UNSPECIFIED.,.F.,.F.,(4,1,1,
1,1,1,1,1,4),(34.5575191894884,34.5580684879192,35.5555917766192,36.5531150653192,
37.5506383540192,38.5481616427193,39.5456849314193,40.5432082201193,40.840704496668),
 .UNSPECIFIED.);
#1466=B_SPLINE_CURVE_WITH_KNOTS('',3,(#55890,#55891,#55892,#55893,#55894,
#55895,#55896,#55897,#55898,#55899),.UNSPECIFIED.,.F.,.F.,(4,1,1,1,1,1,
1,4),(34.5575191894885,35.2415132469841,36.2390365356841,37.2365598243841,
38.2340831130841,39.2316064017841,40.2291296904841,40.8407044966681),
 .UNSPECIFIED.);
#1467=B_SPLINE_CURVE_WITH_KNOTS('',3,(#55904,#55905,#55906,#55907,#55908,
#55909,#55910,#55911,#55912,#55913),.UNSPECIFIED.,.F.,.F.,(4,1,1,1,1,1,
1,4),(28.2743338823088,28.5729287557192,29.5704520444192,30.5679753331192,
31.5654986218192,32.5630219105192,33.5605451992192,34.5575191894884),
 .UNSPECIFIED.);
#1468=B_SPLINE_CURVE_WITH_KNOTS('',3,(#55914,#55915,#55916,#55917,#55918,
#55919,#55920,#55921,#55922,#55923),.UNSPECIFIED.,.F.,.F.,(4,1,1,1,1,1,
1,4),(28.2743338823089,29.256373514784,30.253896803484,31.251420092184,
32.2489433808841,33.2464666695841,34.2439899582841,34.5575191894885),
 .UNSPECIFIED.);
#1469=B_SPLINE_CURVE_WITH_KNOTS('',3,(#55928,#55929,#55930,#55931,#55932,
#55933,#55934,#55935,#55936,#55937),.UNSPECIFIED.,.F.,.F.,(4,1,1,1,1,1,
1,4),(21.9911485751292,22.5877890235192,23.5853123122192,24.5828356009192,
25.5803588896192,26.5778821783192,27.5754054670192,28.2743338823088),
 .UNSPECIFIED.);
#1470=B_SPLINE_CURVE_WITH_KNOTS('',3,(#55938,#55939,#55940,#55941,#55942,
#55943,#55944,#55945,#55946,#55947,#55948),.UNSPECIFIED.,.F.,.F.,(4,1,1,
1,1,1,1,1,4),(21.9911485751293,22.273710493884,23.271233782584,24.268757071284,
25.266280359984,26.263803648684,27.261326937384,28.258850226084,28.2743338823089),
 .UNSPECIFIED.);
#1471=B_SPLINE_CURVE_WITH_KNOTS('',3,(#55953,#55954,#55955,#55956,#55957,
#55958,#55959,#55960,#55961,#55962),.UNSPECIFIED.,.F.,.F.,(4,1,1,1,1,1,
1,4),(15.7079632679496,16.6026492913191,17.6001725800191,18.5976958687191,
19.5952191574192,20.5927424461192,21.5902657348192,21.9911485751292),
 .UNSPECIFIED.);
#1472=B_SPLINE_CURVE_WITH_KNOTS('',3,(#55963,#55964,#55965,#55966,#55967,
#55968,#55969,#55970,#55971,#55972),.UNSPECIFIED.,.F.,.F.,(4,1,1,1,1,1,
1,4),(15.7079632679497,16.288570761684,17.286094050384,18.283617339084,
19.281140627784,20.278663916484,21.276187205184,21.9911485751293),
 .UNSPECIFIED.);
#1473=B_SPLINE_CURVE_WITH_KNOTS('',3,(#57514,#57515,#57516,#57517,#57518,
#57519,#57520,#57521,#57522,#57523,#57524,#57525,#57526,#57527,#57528,#57529,
#57530,#57531,#57532,#57533,#57534,#57535,#57536,#57537,#57538,#57539,#57540,
#57541,#57542,#57543,#57544,#57545,#57546,#57547,#57548,#57549,#57550,#57551,
#57552,#57553,#57554,#57555,#57556,#57557,#57558,#57559,#57560,#57561,#57562,
#57563,#57564,#57565,#57566,#57567,#57568,#57569,#57570,#57571,#57572,#57573,
#57574,#57575,#57576,#57577,#57578,#57579,#57580,#57581,#57582,#57583,#57584,
#57585,#57586,#57587,#57588,#57589,#57590,#57591,#57592,#57593,#57594,#57595,
#57596,#57597,#57598,#57599,#57600,#57601,#57602,#57603,#57604,#57605,#57606,
#57607,#57608,#57609,#57610,#57611,#57612,#57613,#57614,#57615,#57616,#57617,
#57618,#57619,#57620,#57621,#57622),.UNSPECIFIED.,.F.,.F.,(4,3,3,3,3,3,
3,3,3,3,3,3,3,3,3,3,3,3,3,3,3,3,3,3,3,3,3,3,3,3,3,3,3,3,3,3,4),(0.,0.0359628151845056,
0.0790640675124802,0.122944974172411,0.167078080679047,0.180430545026742,
0.19037773183983,0.196180338284082,0.239492682886256,0.282925566791464,
0.325969530232972,0.368238370501489,0.375078460706215,0.381042467863404,
0.42346125387141,0.465393907031249,0.506323913773678,0.51599109870151,0.544714566753401,
0.554178082246963,0.559723896450525,0.565364051500323,0.606359797650403,
0.648015429264718,0.689524423166306,0.717651633141474,0.732581126571207,
0.739096451862393,0.745778843116641,0.786822056096576,0.827804944486442,
0.845389038445888,0.853674880949773,0.860823772315063,0.901249933519242,
0.94103892518765,0.96847769616201),.UNSPECIFIED.);
#1474=B_SPLINE_CURVE_WITH_KNOTS('',3,(#57623,#57624,#57625,#57626,#57627,
#57628,#57629,#57630,#57631,#57632,#57633,#57634,#57635,#57636,#57637,#57638,
#57639,#57640,#57641),.UNSPECIFIED.,.F.,.F.,(4,3,3,3,3,3,4),(371.824326632282,
372.076186685102,373.073709973802,374.071233262502,375.068756551202,376.066279839902,
376.991118430775),.UNSPECIFIED.);
#1475=B_SPLINE_CURVE_WITH_KNOTS('',3,(#57643,#57644,#57645,#57646,#57647,
#57648,#57649,#57650,#57651,#57652,#57653,#57654,#57655,#57656,#57657,#57658,
#57659,#57660,#57661,#57662,#57663,#57664,#57665,#57666,#57667,#57668,#57669,
#57670,#57671,#57672,#57673,#57674,#57675,#57676,#57677,#57678,#57679,#57680,
#57681,#57682,#57683,#57684,#57685,#57686,#57687,#57688,#57689,#57690,#57691,
#57692,#57693,#57694,#57695,#57696,#57697,#57698,#57699,#57700,#57701,#57702,
#57703,#57704,#57705,#57706,#57707,#57708,#57709,#57710,#57711,#57712,#57713,
#57714,#57715,#57716,#57717,#57718,#57719,#57720,#57721,#57722,#57723,#57724,
#57725,#57726,#57727,#57728,#57729,#57730,#57731,#57732,#57733,#57734,#57735,
#57736,#57737,#57738,#57739,#57740,#57741,#57742,#57743,#57744,#57745,#57746,
#57747,#57748),.UNSPECIFIED.,.F.,.F.,(4,3,3,3,3,3,3,3,3,3,3,3,3,3,3,3,3,
3,3,3,3,3,3,3,3,3,3,3,3,3,3,3,3,3,3,4),(-0.968477696161913,-0.936462781732006,
-0.897034237282827,-0.871088158002514,-0.855755616551603,-0.849836345176422,
-0.809673382933614,-0.76870133116664,-0.750776058518589,-0.741856737530979,
-0.7341371378361,-0.692655598295136,-0.650704137993651,-0.608502345694694,
-0.576851001470477,-0.56347054188062,-0.556078670388381,-0.513475355214464,
-0.481896968797825,-0.440388916382611,-0.398291621794682,-0.386095361159993,
-0.379050278062876,-0.373539380612515,-0.331389873213074,-0.287819274607371,
-0.244248676001668,-0.213717591501459,-0.200360242032618,-0.19269654176718,
-0.1869673316623,-0.143586522253231,-0.0997397595963603,-0.0560111116848197,
-0.0129407155146067,0.),.UNSPECIFIED.);
#1476=B_SPLINE_CURVE_WITH_KNOTS('',3,(#57749,#57750,#57751,#57752,#57753,
#57754,#57755,#57756,#57757),.UNSPECIFIED.,.F.,.F.,(4,1,1,1,1,1,4),(10.3761157273111,
11.3009543181839,12.2984776068839,13.2960008955839,14.2935241842839,15.291047472984,
15.7079632679497),.UNSPECIFIED.);
#1477=B_SPLINE_CURVE_WITH_KNOTS('',3,(#57761,#57762,#57763,#57764,#57765,
#57766,#57767,#57768,#57769),.UNSPECIFIED.,.F.,.F.,(4,1,1,1,1,1,4),(11.6150328478191,
12.1137944921691,12.6125561365191,13.6100794252191,14.6076027139191,15.6051260026191,
15.7079632679496),.UNSPECIFIED.);
#1478=B_SPLINE_CURVE_WITH_KNOTS('',3,(#59311,#59312,#59313,#59314,#59315,
#59316,#59317,#59318,#59319,#59320,#59321,#59322,#59323,#59324,#59325,#59326,
#59327,#59328,#59329,#59330,#59331,#59332,#59333,#59334,#59335,#59336,#59337,
#59338,#59339,#59340,#59341,#59342,#59343,#59344,#59345,#59346,#59347,#59348,
#59349,#59350,#59351,#59352,#59353,#59354,#59355,#59356,#59357,#59358,#59359,
#59360,#59361,#59362,#59363,#59364,#59365,#59366,#59367,#59368,#59369,#59370,
#59371,#59372,#59373,#59374,#59375,#59376,#59377,#59378,#59379,#59380,#59381,
#59382,#59383,#59384,#59385,#59386,#59387,#59388,#59389,#59390,#59391,#59392,
#59393,#59394,#59395,#59396,#59397,#59398,#59399,#59400,#59401,#59402,#59403,
#59404,#59405,#59406,#59407,#59408,#59409,#59410,#59411,#59412,#59413,#59414,
#59415,#59416,#59417,#59418,#59419),.UNSPECIFIED.,.F.,.F.,(4,3,3,3,3,3,
3,3,3,3,3,3,3,3,3,3,3,3,3,3,3,3,3,3,3,3,3,3,3,3,3,3,3,3,3,3,4),(0.,0.0319610084124964,
0.0709970802367925,0.110918019903594,0.151489267836741,0.166268550959158,
0.172136820332691,0.17773227169752,0.218621519728627,0.260105203172031,
0.301749535598996,0.343042584632714,0.348577800050639,0.354310610465885,
0.396643769367683,0.438881645932778,0.480394489143215,0.485838103022159,
0.515447494563868,0.527322668925359,0.533096841618444,0.574119197999633,
0.616402831080215,0.659075854182062,0.69089454476895,0.706803890062393,
0.714443723340302,0.720575125052056,0.722713235355837,0.765747942600601,
0.80908641486819,0.828699390062085,0.838036583520388,0.844245630783005,
0.888067982944121,0.931632292905962,0.965990216419354),.UNSPECIFIED.);
#1479=B_SPLINE_CURVE_WITH_KNOTS('',3,(#59420,#59421,#59422,#59423,#59424,
#59425,#59426,#59427,#59428,#59429,#59430,#59431,#59432,#59433,#59434,#59435,
#59436,#59437,#59438,#59439,#59440,#59441,#59442,#59443,#59444,#59445,#59446,
#59447,#59448,#59449,#59450,#59451,#59452,#59453,#59454,#59455,#59456,#59457,
#59458,#59459,#59460,#59461,#59462,#59463,#59464,#59465,#59466,#59467,#59468,
#59469,#59470,#59471,#59472,#59473,#59474,#59475,#59476,#59477,#59478,#59479,
#59480,#59481,#59482,#59483,#59484,#59485,#59486,#59487,#59488,#59489,#59490,
#59491,#59492,#59493,#59494,#59495,#59496,#59497,#59498,#59499,#59500,#59501,
#59502,#59503,#59504,#59505,#59506,#59507,#59508,#59509,#59510,#59511,#59512,
#59513,#59514,#59515,#59516,#59517,#59518,#59519,#59520,#59521,#59522),
 .UNSPECIFIED.,.F.,.F.,(4,3,3,3,3,3,3,3,3,3,3,3,3,3,3,3,3,3,3,3,3,3,3,3,
3,3,3,3,3,3,3,3,3,3,4),(-0.965990216419533,-0.930132396483882,-0.886600314752691,
-0.859427241407658,-0.844575649172136,-0.83450269382505,-0.791217440053876,
-0.748794152701163,-0.730233964484351,-0.71490535117285,-0.708744621568391,
-0.665691199232105,-0.622727628938354,-0.580003507011809,-0.5479604155669,
-0.535021607402038,-0.529041072836267,-0.487381790675506,-0.451831141232172,
-0.409951411560376,-0.367982065107459,-0.353448430125576,-0.345247061313217,
-0.304116472475951,-0.262917042414806,-0.222498465588061,-0.194686157389553,
-0.181409937644946,-0.17316340151046,-0.167260443835079,-0.125445332876309,
-0.0850027204681986,-0.0449509623998064,-0.00571310113625183,0.),
 .UNSPECIFIED.);
#1480=B_SPLINE_CURVE_WITH_KNOTS('',3,(#59523,#59524,#59525,#59526,#59527,
#59528,#59529,#59530,#59531,#59532,#59533,#59534,#59535,#59536,#59537,#59538,
#59539,#59540,#59541),.UNSPECIFIED.,.F.,.F.,(4,3,3,3,3,3,4),(-379.058849706002,
-378.560088061652,-378.061326417302,-377.063803128602,-376.066279839902,
-375.068756551202,-374.800863543725),.UNSPECIFIED.);
#1998=CYLINDRICAL_SURFACE('',#15254,4.942);
#1999=CYLINDRICAL_SURFACE('',#15256,4.942);
#2000=CYLINDRICAL_SURFACE('',#15257,4.942);
#2001=CYLINDRICAL_SURFACE('',#15258,4.942);
#2002=CYLINDRICAL_SURFACE('',#15259,4.942);
#2003=CYLINDRICAL_SURFACE('',#15260,4.942);
#2004=CYLINDRICAL_SURFACE('',#15261,4.942);
#2005=CYLINDRICAL_SURFACE('',#15262,4.942);
#2006=CYLINDRICAL_SURFACE('',#15263,4.942);
#2007=CYLINDRICAL_SURFACE('',#15264,4.942);
#2008=CYLINDRICAL_SURFACE('',#15265,4.942);
#2009=CYLINDRICAL_SURFACE('',#15266,4.942);
#2010=CYLINDRICAL_SURFACE('',#15267,4.942);
#2011=CYLINDRICAL_SURFACE('',#15268,4.942);
#2012=CYLINDRICAL_SURFACE('',#15269,4.942);
#2013=CYLINDRICAL_SURFACE('',#15270,4.942);
#2014=CYLINDRICAL_SURFACE('',#15271,4.942);
#2015=CYLINDRICAL_SURFACE('',#15272,4.942);
#2016=CYLINDRICAL_SURFACE('',#15273,4.942);
#2017=CYLINDRICAL_SURFACE('',#15274,4.942);
#2018=CYLINDRICAL_SURFACE('',#15275,4.942);
#2019=CYLINDRICAL_SURFACE('',#15276,4.942);
#2020=CYLINDRICAL_SURFACE('',#15277,4.942);
#2021=CYLINDRICAL_SURFACE('',#15278,4.942);
#2022=CYLINDRICAL_SURFACE('',#15279,4.942);
#2023=CYLINDRICAL_SURFACE('',#15280,4.942);
#2024=CYLINDRICAL_SURFACE('',#15281,4.942);
#2025=CYLINDRICAL_SURFACE('',#15282,4.942);
#2026=CYLINDRICAL_SURFACE('',#15283,4.942);
#2027=CYLINDRICAL_SURFACE('',#15284,4.942);
#2028=CYLINDRICAL_SURFACE('',#15285,4.942);
#2029=CYLINDRICAL_SURFACE('',#15286,4.942);
#2030=CYLINDRICAL_SURFACE('',#15287,4.942);
#2031=CYLINDRICAL_SURFACE('',#15288,4.942);
#2032=CYLINDRICAL_SURFACE('',#15289,4.942);
#2033=CYLINDRICAL_SURFACE('',#15290,4.942);
#2034=CYLINDRICAL_SURFACE('',#15291,4.942);
#2035=CYLINDRICAL_SURFACE('',#15292,4.942);
#2036=CYLINDRICAL_SURFACE('',#15293,4.942);
#2037=CYLINDRICAL_SURFACE('',#15294,4.942);
#2038=CYLINDRICAL_SURFACE('',#15295,4.942);
#2039=CYLINDRICAL_SURFACE('',#15296,4.942);
#2040=CYLINDRICAL_SURFACE('',#15297,4.942);
#2041=CYLINDRICAL_SURFACE('',#15298,4.942);
#2042=CYLINDRICAL_SURFACE('',#15299,4.942);
#2043=CYLINDRICAL_SURFACE('',#15300,4.942);
#2044=CYLINDRICAL_SURFACE('',#15301,4.942);
#2045=CYLINDRICAL_SURFACE('',#15302,4.942);
#2046=CYLINDRICAL_SURFACE('',#15303,4.942);
#2047=CYLINDRICAL_SURFACE('',#15304,4.942);
#2048=CYLINDRICAL_SURFACE('',#15305,4.942);
#2049=CYLINDRICAL_SURFACE('',#15306,4.942);
#2050=CYLINDRICAL_SURFACE('',#15307,4.942);
#2051=CYLINDRICAL_SURFACE('',#15308,4.942);
#2052=CYLINDRICAL_SURFACE('',#15309,4.942);
#2053=CYLINDRICAL_SURFACE('',#15310,4.942);
#2054=CYLINDRICAL_SURFACE('',#15311,4.942);
#2055=CYLINDRICAL_SURFACE('',#15312,4.942);
#2056=CYLINDRICAL_SURFACE('',#15313,4.942);
#2057=CYLINDRICAL_SURFACE('',#15314,4.942);
#2058=CYLINDRICAL_SURFACE('',#15315,4.372);
#2059=CYLINDRICAL_SURFACE('',#15317,4.372);
#2060=CYLINDRICAL_SURFACE('',#15318,4.372);
#2061=CYLINDRICAL_SURFACE('',#15319,4.372);
#2062=CYLINDRICAL_SURFACE('',#15320,4.372);
#2063=CYLINDRICAL_SURFACE('',#15321,4.372);
#2064=CYLINDRICAL_SURFACE('',#15322,4.372);
#2065=CYLINDRICAL_SURFACE('',#15323,4.372);
#2066=CYLINDRICAL_SURFACE('',#15324,4.372);
#2067=CYLINDRICAL_SURFACE('',#15325,4.372);
#2068=CYLINDRICAL_SURFACE('',#15326,4.372);
#2069=CYLINDRICAL_SURFACE('',#15327,4.372);
#2070=CYLINDRICAL_SURFACE('',#15328,4.372);
#2071=CYLINDRICAL_SURFACE('',#15329,4.372);
#2072=CYLINDRICAL_SURFACE('',#15330,4.372);
#2073=CYLINDRICAL_SURFACE('',#15331,4.372);
#2074=CYLINDRICAL_SURFACE('',#15332,4.372);
#2075=CYLINDRICAL_SURFACE('',#15333,4.372);
#2076=CYLINDRICAL_SURFACE('',#15334,4.372);
#2077=CYLINDRICAL_SURFACE('',#15335,4.372);
#2078=CYLINDRICAL_SURFACE('',#15336,4.372);
#2079=CYLINDRICAL_SURFACE('',#15337,4.372);
#2080=CYLINDRICAL_SURFACE('',#15338,4.372);
#2081=CYLINDRICAL_SURFACE('',#15339,4.372);
#2082=CYLINDRICAL_SURFACE('',#15340,4.372);
#2083=CYLINDRICAL_SURFACE('',#15341,4.372);
#2084=CYLINDRICAL_SURFACE('',#15342,4.372);
#2085=CYLINDRICAL_SURFACE('',#15343,4.372);
#2086=CYLINDRICAL_SURFACE('',#15344,4.372);
#2087=CYLINDRICAL_SURFACE('',#15345,4.372);
#2088=CYLINDRICAL_SURFACE('',#15346,4.372);
#2089=CYLINDRICAL_SURFACE('',#15347,4.372);
#2090=CYLINDRICAL_SURFACE('',#15348,4.372);
#2091=CYLINDRICAL_SURFACE('',#15349,4.372);
#2092=CYLINDRICAL_SURFACE('',#15350,4.372);
#2093=CYLINDRICAL_SURFACE('',#15351,4.372);
#2094=CYLINDRICAL_SURFACE('',#15352,4.372);
#2095=CYLINDRICAL_SURFACE('',#15353,4.372);
#2096=CYLINDRICAL_SURFACE('',#15354,4.372);
#2097=CYLINDRICAL_SURFACE('',#15355,4.372);
#2098=CYLINDRICAL_SURFACE('',#15356,4.372);
#2099=CYLINDRICAL_SURFACE('',#15357,4.372);
#2100=CYLINDRICAL_SURFACE('',#15358,4.372);
#2101=CYLINDRICAL_SURFACE('',#15359,4.372);
#2102=CYLINDRICAL_SURFACE('',#15360,4.372);
#2103=CYLINDRICAL_SURFACE('',#15361,4.372);
#2104=CYLINDRICAL_SURFACE('',#15362,4.372);
#2105=CYLINDRICAL_SURFACE('',#15363,4.372);
#2106=CYLINDRICAL_SURFACE('',#15364,4.372);
#2107=CYLINDRICAL_SURFACE('',#15365,4.372);
#2108=CYLINDRICAL_SURFACE('',#15366,4.372);
#2109=CYLINDRICAL_SURFACE('',#15367,4.372);
#2110=CYLINDRICAL_SURFACE('',#15368,4.372);
#2111=CYLINDRICAL_SURFACE('',#15369,4.372);
#2112=CYLINDRICAL_SURFACE('',#15370,4.372);
#2113=CYLINDRICAL_SURFACE('',#15371,4.372);
#2114=CYLINDRICAL_SURFACE('',#15372,4.372);
#2115=CYLINDRICAL_SURFACE('',#15373,4.372);
#2116=CYLINDRICAL_SURFACE('',#15374,4.372);
#2117=CYLINDRICAL_SURFACE('',#15375,4.372);
#2118=CYLINDRICAL_SURFACE('',#15376,4.372);
#2119=CYLINDRICAL_SURFACE('',#15378,4.942);
#2120=CYLINDRICAL_SURFACE('',#15389,5.);
#2187=SHAPE_REPRESENTATION_RELATIONSHIP('SRR','None',#63872,#2203);
#2203=ADVANCED_BREP_SHAPE_REPRESENTATION('',(#2235),#63750);
#2219=STYLED_ITEM('',(#63963),#2235);
#2235=MANIFOLD_SOLID_BREP('Body1',#14320);
#2293=FACE_BOUND('',#3784,.T.);
#2294=FACE_BOUND('',#3786,.T.);
#2846=FACE_OUTER_BOUND('',#3659,.T.);
#2847=FACE_OUTER_BOUND('',#3660,.T.);
#2848=FACE_OUTER_BOUND('',#3661,.T.);
#2849=FACE_OUTER_BOUND('',#3662,.T.);
#2850=FACE_OUTER_BOUND('',#3663,.T.);
#2851=FACE_OUTER_BOUND('',#3664,.T.);
#2852=FACE_OUTER_BOUND('',#3665,.T.);
#2853=FACE_OUTER_BOUND('',#3666,.T.);
#2854=FACE_OUTER_BOUND('',#3667,.T.);
#2855=FACE_OUTER_BOUND('',#3668,.T.);
#2856=FACE_OUTER_BOUND('',#3669,.T.);
#2857=FACE_OUTER_BOUND('',#3670,.T.);
#2858=FACE_OUTER_BOUND('',#3671,.T.);
#2859=FACE_OUTER_BOUND('',#3672,.T.);
#2860=FACE_OUTER_BOUND('',#3673,.T.);
#2861=FACE_OUTER_BOUND('',#3674,.T.);
#2862=FACE_OUTER_BOUND('',#3675,.T.);
#2863=FACE_OUTER_BOUND('',#3676,.T.);
#2864=FACE_OUTER_BOUND('',#3677,.T.);
#2865=FACE_OUTER_BOUND('',#3678,.T.);
#2866=FACE_OUTER_BOUND('',#3679,.T.);
#2867=FACE_OUTER_BOUND('',#3680,.T.);
#2868=FACE_OUTER_BOUND('',#3681,.T.);
#2869=FACE_OUTER_BOUND('',#3682,.T.);
#2870=FACE_OUTER_BOUND('',#3683,.T.);
#2871=FACE_OUTER_BOUND('',#3684,.T.);
#2872=FACE_OUTER_BOUND('',#3685,.T.);
#2873=FACE_OUTER_BOUND('',#3686,.T.);
#2874=FACE_OUTER_BOUND('',#3687,.T.);
#2875=FACE_OUTER_BOUND('',#3688,.T.);
#2876=FACE_OUTER_BOUND('',#3689,.T.);
#2877=FACE_OUTER_BOUND('',#3690,.T.);
#2878=FACE_OUTER_BOUND('',#3691,.T.);
#2879=FACE_OUTER_BOUND('',#3692,.T.);
#2880=FACE_OUTER_BOUND('',#3693,.T.);
#2881=FACE_OUTER_BOUND('',#3694,.T.);
#2882=FACE_OUTER_BOUND('',#3695,.T.);
#2883=FACE_OUTER_BOUND('',#3696,.T.);
#2884=FACE_OUTER_BOUND('',#3697,.T.);
#2885=FACE_OUTER_BOUND('',#3698,.T.);
#2886=FACE_OUTER_BOUND('',#3699,.T.);
#2887=FACE_OUTER_BOUND('',#3700,.T.);
#2888=FACE_OUTER_BOUND('',#3701,.T.);
#2889=FACE_OUTER_BOUND('',#3702,.T.);
#2890=FACE_OUTER_BOUND('',#3703,.T.);
#2891=FACE_OUTER_BOUND('',#3704,.T.);
#2892=FACE_OUTER_BOUND('',#3705,.T.);
#2893=FACE_OUTER_BOUND('',#3706,.T.);
#2894=FACE_OUTER_BOUND('',#3707,.T.);
#2895=FACE_OUTER_BOUND('',#3708,.T.);
#2896=FACE_OUTER_BOUND('',#3709,.T.);
#2897=FACE_OUTER_BOUND('',#3710,.T.);
#2898=FACE_OUTER_BOUND('',#3711,.T.);
#2899=FACE_OUTER_BOUND('',#3712,.T.);
#2900=FACE_OUTER_BOUND('',#3713,.T.);
#2901=FACE_OUTER_BOUND('',#3714,.T.);
#2902=FACE_OUTER_BOUND('',#3715,.T.);
#2903=FACE_OUTER_BOUND('',#3716,.T.);
#2904=FACE_OUTER_BOUND('',#3717,.T.);
#2905=FACE_OUTER_BOUND('',#3718,.T.);
#2906=FACE_OUTER_BOUND('',#3719,.T.);
#2907=FACE_OUTER_BOUND('',#3720,.T.);
#2908=FACE_OUTER_BOUND('',#3721,.T.);
#2909=FACE_OUTER_BOUND('',#3722,.T.);
#2910=FACE_OUTER_BOUND('',#3723,.T.);
#2911=FACE_OUTER_BOUND('',#3724,.T.);
#2912=FACE_OUTER_BOUND('',#3725,.T.);
#2913=FACE_OUTER_BOUND('',#3726,.T.);
#2914=FACE_OUTER_BOUND('',#3727,.T.);
#2915=FACE_OUTER_BOUND('',#3728,.T.);
#2916=FACE_OUTER_BOUND('',#3729,.T.);
#2917=FACE_OUTER_BOUND('',#3730,.T.);
#2918=FACE_OUTER_BOUND('',#3731,.T.);
#2919=FACE_OUTER_BOUND('',#3732,.T.);
#2920=FACE_OUTER_BOUND('',#3733,.T.);
#2921=FACE_OUTER_BOUND('',#3734,.T.);
#2922=FACE_OUTER_BOUND('',#3735,.T.);
#2923=FACE_OUTER_BOUND('',#3736,.T.);
#2924=FACE_OUTER_BOUND('',#3737,.T.);
#2925=FACE_OUTER_BOUND('',#3738,.T.);
#2926=FACE_OUTER_BOUND('',#3739,.T.);
#2927=FACE_OUTER_BOUND('',#3740,.T.);
#2928=FACE_OUTER_BOUND('',#3741,.T.);
#2929=FACE_OUTER_BOUND('',#3742,.T.);
#2930=FACE_OUTER_BOUND('',#3743,.T.);
#2931=FACE_OUTER_BOUND('',#3744,.T.);
#2932=FACE_OUTER_BOUND('',#3745,.T.);
#2933=FACE_OUTER_BOUND('',#3746,.T.);
#2934=FACE_OUTER_BOUND('',#3747,.T.);
#2935=FACE_OUTER_BOUND('',#3748,.T.);
#2936=FACE_OUTER_BOUND('',#3749,.T.);
#2937=FACE_OUTER_BOUND('',#3750,.T.);
#2938=FACE_OUTER_BOUND('',#3751,.T.);
#2939=FACE_OUTER_BOUND('',#3752,.T.);
#2940=FACE_OUTER_BOUND('',#3753,.T.);
#2941=FACE_OUTER_BOUND('',#3754,.T.);
#2942=FACE_OUTER_BOUND('',#3755,.T.);
#2943=FACE_OUTER_BOUND('',#3756,.T.);
#2944=FACE_OUTER_BOUND('',#3757,.T.);
#2945=FACE_OUTER_BOUND('',#3758,.T.);
#2946=FACE_OUTER_BOUND('',#3759,.T.);
#2947=FACE_OUTER_BOUND('',#3760,.T.);
#2948=FACE_OUTER_BOUND('',#3761,.T.);
#2949=FACE_OUTER_BOUND('',#3762,.T.);
#2950=FACE_OUTER_BOUND('',#3763,.T.);
#2951=FACE_OUTER_BOUND('',#3764,.T.);
#2952=FACE_OUTER_BOUND('',#3765,.T.);
#2953=FACE_OUTER_BOUND('',#3766,.T.);
#2954=FACE_OUTER_BOUND('',#3767,.T.);
#2955=FACE_OUTER_BOUND('',#3768,.T.);
#2956=FACE_OUTER_BOUND('',#3769,.T.);
#2957=FACE_OUTER_BOUND('',#3770,.T.);
#2958=FACE_OUTER_BOUND('',#3771,.T.);
#2959=FACE_OUTER_BOUND('',#3772,.T.);
#2960=FACE_OUTER_BOUND('',#3773,.T.);
#2961=FACE_OUTER_BOUND('',#3774,.T.);
#2962=FACE_OUTER_BOUND('',#3775,.T.);
#2963=FACE_OUTER_BOUND('',#3776,.T.);
#2964=FACE_OUTER_BOUND('',#3777,.T.);
#2965=FACE_OUTER_BOUND('',#3778,.T.);
#2966=FACE_OUTER_BOUND('',#3779,.T.);
#2967=FACE_OUTER_BOUND('',#3780,.T.);
#2968=FACE_OUTER_BOUND('',#3781,.T.);
#2969=FACE_OUTER_BOUND('',#3782,.T.);
#2970=FACE_OUTER_BOUND('',#3783,.T.);
#2971=FACE_OUTER_BOUND('',#3785,.T.);
#2972=FACE_OUTER_BOUND('',#3787,.T.);
#2973=FACE_OUTER_BOUND('',#3788,.T.);
#2974=FACE_OUTER_BOUND('',#3789,.T.);
#2975=FACE_OUTER_BOUND('',#3790,.T.);
#2976=FACE_OUTER_BOUND('',#3791,.T.);
#2977=FACE_OUTER_BOUND('',#3792,.T.);
#2978=FACE_OUTER_BOUND('',#3793,.T.);
#2979=FACE_OUTER_BOUND('',#3794,.T.);
#2980=FACE_OUTER_BOUND('',#3795,.T.);
#3659=EDGE_LOOP('',(#12189,#12190,#12191,#12192));
#3660=EDGE_LOOP('',(#12193,#12194,#12195,#12196));
#3661=EDGE_LOOP('',(#12197,#12198,#12199,#12200));
#3662=EDGE_LOOP('',(#12201,#12202,#12203,#12204));
#3663=EDGE_LOOP('',(#12205,#12206,#12207,#12208));
#3664=EDGE_LOOP('',(#12209,#12210,#12211,#12212));
#3665=EDGE_LOOP('',(#12213,#12214,#12215,#12216));
#3666=EDGE_LOOP('',(#12217,#12218,#12219,#12220));
#3667=EDGE_LOOP('',(#12221,#12222,#12223,#12224));
#3668=EDGE_LOOP('',(#12225,#12226,#12227,#12228));
#3669=EDGE_LOOP('',(#12229,#12230,#12231,#12232));
#3670=EDGE_LOOP('',(#12233,#12234,#12235,#12236));
#3671=EDGE_LOOP('',(#12237,#12238,#12239,#12240));
#3672=EDGE_LOOP('',(#12241,#12242,#12243,#12244));
#3673=EDGE_LOOP('',(#12245,#12246,#12247,#12248));
#3674=EDGE_LOOP('',(#12249,#12250,#12251,#12252));
#3675=EDGE_LOOP('',(#12253,#12254,#12255,#12256));
#3676=EDGE_LOOP('',(#12257,#12258,#12259,#12260));
#3677=EDGE_LOOP('',(#12261,#12262,#12263,#12264));
#3678=EDGE_LOOP('',(#12265,#12266,#12267,#12268));
#3679=EDGE_LOOP('',(#12269,#12270,#12271,#12272));
#3680=EDGE_LOOP('',(#12273,#12274,#12275,#12276));
#3681=EDGE_LOOP('',(#12277,#12278,#12279,#12280));
#3682=EDGE_LOOP('',(#12281,#12282,#12283,#12284));
#3683=EDGE_LOOP('',(#12285,#12286,#12287,#12288));
#3684=EDGE_LOOP('',(#12289,#12290,#12291,#12292));
#3685=EDGE_LOOP('',(#12293,#12294,#12295,#12296));
#3686=EDGE_LOOP('',(#12297,#12298,#12299,#12300));
#3687=EDGE_LOOP('',(#12301,#12302,#12303,#12304));
#3688=EDGE_LOOP('',(#12305,#12306,#12307,#12308));
#3689=EDGE_LOOP('',(#12309,#12310,#12311,#12312));
#3690=EDGE_LOOP('',(#12313,#12314,#12315,#12316));
#3691=EDGE_LOOP('',(#12317,#12318,#12319,#12320));
#3692=EDGE_LOOP('',(#12321,#12322,#12323,#12324));
#3693=EDGE_LOOP('',(#12325,#12326,#12327,#12328));
#3694=EDGE_LOOP('',(#12329,#12330,#12331,#12332));
#3695=EDGE_LOOP('',(#12333,#12334,#12335,#12336));
#3696=EDGE_LOOP('',(#12337,#12338,#12339,#12340));
#3697=EDGE_LOOP('',(#12341,#12342,#12343,#12344));
#3698=EDGE_LOOP('',(#12345,#12346,#12347,#12348));
#3699=EDGE_LOOP('',(#12349,#12350,#12351,#12352));
#3700=EDGE_LOOP('',(#12353,#12354,#12355,#12356));
#3701=EDGE_LOOP('',(#12357,#12358,#12359,#12360));
#3702=EDGE_LOOP('',(#12361,#12362,#12363,#12364));
#3703=EDGE_LOOP('',(#12365,#12366,#12367,#12368));
#3704=EDGE_LOOP('',(#12369,#12370,#12371,#12372));
#3705=EDGE_LOOP('',(#12373,#12374,#12375,#12376));
#3706=EDGE_LOOP('',(#12377,#12378,#12379,#12380));
#3707=EDGE_LOOP('',(#12381,#12382,#12383,#12384));
#3708=EDGE_LOOP('',(#12385,#12386,#12387,#12388));
#3709=EDGE_LOOP('',(#12389,#12390,#12391,#12392));
#3710=EDGE_LOOP('',(#12393,#12394,#12395,#12396));
#3711=EDGE_LOOP('',(#12397,#12398,#12399,#12400));
#3712=EDGE_LOOP('',(#12401,#12402,#12403,#12404));
#3713=EDGE_LOOP('',(#12405,#12406,#12407,#12408));
#3714=EDGE_LOOP('',(#12409,#12410,#12411,#12412));
#3715=EDGE_LOOP('',(#12413,#12414,#12415,#12416));
#3716=EDGE_LOOP('',(#12417,#12418,#12419,#12420));
#3717=EDGE_LOOP('',(#12421,#12422,#12423,#12424));
#3718=EDGE_LOOP('',(#12425,#12426,#12427,#12428));
#3719=EDGE_LOOP('',(#12429,#12430,#12431,#12432));
#3720=EDGE_LOOP('',(#12433,#12434,#12435,#12436));
#3721=EDGE_LOOP('',(#12437,#12438,#12439,#12440));
#3722=EDGE_LOOP('',(#12441,#12442,#12443,#12444));
#3723=EDGE_LOOP('',(#12445,#12446,#12447,#12448));
#3724=EDGE_LOOP('',(#12449,#12450,#12451,#12452));
#3725=EDGE_LOOP('',(#12453,#12454,#12455,#12456));
#3726=EDGE_LOOP('',(#12457,#12458,#12459,#12460));
#3727=EDGE_LOOP('',(#12461,#12462,#12463,#12464));
#3728=EDGE_LOOP('',(#12465,#12466,#12467,#12468));
#3729=EDGE_LOOP('',(#12469,#12470,#12471,#12472));
#3730=EDGE_LOOP('',(#12473,#12474,#12475,#12476));
#3731=EDGE_LOOP('',(#12477,#12478,#12479,#12480));
#3732=EDGE_LOOP('',(#12481,#12482,#12483,#12484));
#3733=EDGE_LOOP('',(#12485,#12486,#12487,#12488));
#3734=EDGE_LOOP('',(#12489,#12490,#12491,#12492));
#3735=EDGE_LOOP('',(#12493,#12494,#12495,#12496));
#3736=EDGE_LOOP('',(#12497,#12498,#12499,#12500));
#3737=EDGE_LOOP('',(#12501,#12502,#12503,#12504));
#3738=EDGE_LOOP('',(#12505,#12506,#12507,#12508));
#3739=EDGE_LOOP('',(#12509,#12510,#12511,#12512));
#3740=EDGE_LOOP('',(#12513,#12514,#12515,#12516));
#3741=EDGE_LOOP('',(#12517,#12518,#12519,#12520));
#3742=EDGE_LOOP('',(#12521,#12522,#12523,#12524));
#3743=EDGE_LOOP('',(#12525,#12526,#12527,#12528));
#3744=EDGE_LOOP('',(#12529,#12530,#12531,#12532));
#3745=EDGE_LOOP('',(#12533,#12534,#12535,#12536));
#3746=EDGE_LOOP('',(#12537,#12538,#12539,#12540));
#3747=EDGE_LOOP('',(#12541,#12542,#12543,#12544));
#3748=EDGE_LOOP('',(#12545,#12546,#12547,#12548));
#3749=EDGE_LOOP('',(#12549,#12550,#12551,#12552));
#3750=EDGE_LOOP('',(#12553,#12554,#12555,#12556));
#3751=EDGE_LOOP('',(#12557,#12558,#12559,#12560));
#3752=EDGE_LOOP('',(#12561,#12562,#12563,#12564));
#3753=EDGE_LOOP('',(#12565,#12566,#12567,#12568));
#3754=EDGE_LOOP('',(#12569,#12570,#12571,#12572));
#3755=EDGE_LOOP('',(#12573,#12574,#12575,#12576));
#3756=EDGE_LOOP('',(#12577,#12578,#12579,#12580));
#3757=EDGE_LOOP('',(#12581,#12582,#12583,#12584));
#3758=EDGE_LOOP('',(#12585,#12586,#12587,#12588));
#3759=EDGE_LOOP('',(#12589,#12590,#12591,#12592));
#3760=EDGE_LOOP('',(#12593,#12594,#12595,#12596));
#3761=EDGE_LOOP('',(#12597,#12598,#12599,#12600));
#3762=EDGE_LOOP('',(#12601,#12602,#12603,#12604));
#3763=EDGE_LOOP('',(#12605,#12606,#12607,#12608));
#3764=EDGE_LOOP('',(#12609,#12610,#12611,#12612));
#3765=EDGE_LOOP('',(#12613,#12614,#12615,#12616));
#3766=EDGE_LOOP('',(#12617,#12618,#12619,#12620));
#3767=EDGE_LOOP('',(#12621,#12622,#12623,#12624));
#3768=EDGE_LOOP('',(#12625,#12626,#12627,#12628));
#3769=EDGE_LOOP('',(#12629,#12630,#12631,#12632));
#3770=EDGE_LOOP('',(#12633,#12634,#12635,#12636));
#3771=EDGE_LOOP('',(#12637,#12638,#12639,#12640));
#3772=EDGE_LOOP('',(#12641,#12642,#12643,#12644));
#3773=EDGE_LOOP('',(#12645,#12646,#12647,#12648));
#3774=EDGE_LOOP('',(#12649,#12650,#12651,#12652));
#3775=EDGE_LOOP('',(#12653,#12654,#12655,#12656));
#3776=EDGE_LOOP('',(#12657,#12658,#12659,#12660));
#3777=EDGE_LOOP('',(#12661,#12662,#12663,#12664));
#3778=EDGE_LOOP('',(#12665,#12666,#12667,#12668));
#3779=EDGE_LOOP('',(#12669,#12670,#12671,#12672,#12673,#12674,#12675,#12676,
#12677,#12678,#12679,#12680,#12681,#12682,#12683,#12684,#12685,#12686,#12687,
#12688,#12689,#12690,#12691,#12692,#12693,#12694,#12695,#12696,#12697,#12698,
#12699,#12700,#12701,#12702,#12703,#12704,#12705,#12706,#12707,#12708,#12709,
#12710,#12711,#12712,#12713,#12714,#12715,#12716,#12717,#12718,#12719,#12720,
#12721,#12722,#12723,#12724,#12725,#12726,#12727,#12728,#12729,#12730,#12731,
#12732,#12733,#12734,#12735,#12736,#12737,#12738,#12739,#12740,#12741,#12742,
#12743,#12744,#12745,#12746,#12747,#12748,#12749,#12750,#12751,#12752,#12753,
#12754,#12755,#12756,#12757,#12758,#12759,#12760,#12761,#12762,#12763,#12764,
#12765,#12766,#12767,#12768,#12769,#12770,#12771,#12772,#12773,#12774,#12775,
#12776,#12777,#12778,#12779,#12780,#12781,#12782,#12783,#12784,#12785,#12786,
#12787,#12788,#12789,#12790,#12791,#12792));
#3780=EDGE_LOOP('',(#12793,#12794,#12795,#12796));
#3781=EDGE_LOOP('',(#12797,#12798,#12799,#12800,#12801,#12802,#12803,#12804,
#12805,#12806,#12807,#12808,#12809,#12810,#12811,#12812,#12813,#12814,#12815,
#12816,#12817,#12818,#12819,#12820,#12821,#12822,#12823,#12824,#12825,#12826,
#12827,#12828,#12829,#12830,#12831,#12832,#12833,#12834,#12835,#12836,#12837,
#12838,#12839,#12840,#12841,#12842,#12843,#12844,#12845,#12846,#12847,#12848,
#12849,#12850,#12851,#12852,#12853,#12854,#12855,#12856,#12857,#12858,#12859,
#12860,#12861,#12862,#12863,#12864,#12865,#12866,#12867,#12868,#12869,#12870,
#12871,#12872,#12873,#12874,#12875,#12876,#12877,#12878,#12879,#12880,#12881,
#12882,#12883,#12884,#12885,#12886,#12887,#12888,#12889,#12890,#12891,#12892,
#12893,#12894,#12895,#12896,#12897,#12898,#12899,#12900,#12901,#12902,#12903,
#12904,#12905,#12906,#12907,#12908,#12909,#12910,#12911,#12912,#12913,#12914,
#12915,#12916,#12917,#12918,#12919,#12920));
#3782=EDGE_LOOP('',(#12921,#12922,#12923,#12924));
#3783=EDGE_LOOP('',(#12925,#12926,#12927,#12928,#12929,#12930));
#3784=EDGE_LOOP('',(#12931,#12932,#12933,#12934));
#3785=EDGE_LOOP('',(#12935,#12936,#12937,#12938,#12939,#12940));
#3786=EDGE_LOOP('',(#12941));
#3787=EDGE_LOOP('',(#12942,#12943,#12944,#12945));
#3788=EDGE_LOOP('',(#12946,#12947,#12948,#12949));
#3789=EDGE_LOOP('',(#12950,#12951,#12952,#12953));
#3790=EDGE_LOOP('',(#12954,#12955,#12956,#12957));
#3791=EDGE_LOOP('',(#12958,#12959,#12960,#12961));
#3792=EDGE_LOOP('',(#12962,#12963,#12964,#12965));
#3793=EDGE_LOOP('',(#12966,#12967,#12968,#12969));
#3794=EDGE_LOOP('',(#12970,#12971,#12972,#12973));
#3795=EDGE_LOOP('',(#12974,#12975,#12976));
#4495=LINE('',#51549,#5331);
#4496=LINE('',#51576,#5332);
#4497=LINE('',#51624,#5333);
#4498=LINE('',#51672,#5334);
#4499=LINE('',#51723,#5335);
#4500=LINE('',#51771,#5336);
#4501=LINE('',#51819,#5337);
#4502=LINE('',#51867,#5338);
#4503=LINE('',#51921,#5339);
#4504=LINE('',#51969,#5340);
#4505=LINE('',#52017,#5341);
#4506=LINE('',#52071,#5342);
#4507=LINE('',#52119,#5343);
#4508=LINE('',#52167,#5344);
#4509=LINE('',#52218,#5345);
#4510=LINE('',#52269,#5346);
#4511=LINE('',#52317,#5347);
#4512=LINE('',#52365,#5348);
#4513=LINE('',#52419,#5349);
#4514=LINE('',#52467,#5350);
#4515=LINE('',#52515,#5351);
#4516=LINE('',#52569,#5352);
#4517=LINE('',#52617,#5353);
#4518=LINE('',#52665,#5354);
#4519=LINE('',#52713,#5355);
#4520=LINE('',#52767,#5356);
#4521=LINE('',#52815,#5357);
#4522=LINE('',#52863,#5358);
#4523=LINE('',#52917,#5359);
#4524=LINE('',#52965,#5360);
#4525=LINE('',#53013,#5361);
#4526=LINE('',#53067,#5362);
#4527=LINE('',#53115,#5363);
#4528=LINE('',#53163,#5364);
#4529=LINE('',#53211,#5365);
#4530=LINE('',#53265,#5366);
#4531=LINE('',#53313,#5367);
#4532=LINE('',#53361,#5368);
#4533=LINE('',#53415,#5369);
#4534=LINE('',#53463,#5370);
#4535=LINE('',#53511,#5371);
#4536=LINE('',#53565,#5372);
#4537=LINE('',#53613,#5373);
#4538=LINE('',#53661,#5374);
#4539=LINE('',#53709,#5375);
#4540=LINE('',#53763,#5376);
#4541=LINE('',#53811,#5377);
#4542=LINE('',#53859,#5378);
#4543=LINE('',#53913,#5379);
#4544=LINE('',#53961,#5380);
#4545=LINE('',#54009,#5381);
#4546=LINE('',#54063,#5382);
#4547=LINE('',#54111,#5383);
#4548=LINE('',#54159,#5384);
#4549=LINE('',#54207,#5385);
#4550=LINE('',#54261,#5386);
#4551=LINE('',#54309,#5387);
#4552=LINE('',#54357,#5388);
#4553=LINE('',#54411,#5389);
#4554=LINE('',#54459,#5390);
#4555=LINE('',#54507,#5391);
#4556=LINE('',#54525,#5392);
#4557=LINE('',#54550,#5393);
#4558=LINE('',#54574,#5394);
#4559=LINE('',#54599,#5395);
#4560=LINE('',#54624,#5396);
#4561=LINE('',#54648,#5397);
#4562=LINE('',#54673,#5398);
#4563=LINE('',#54698,#5399);
#4564=LINE('',#54722,#5400);
#4565=LINE('',#54746,#5401);
#4566=LINE('',#54771,#5402);
#4567=LINE('',#54796,#5403);
#4568=LINE('',#54820,#5404);
#4569=LINE('',#54845,#5405);
#4570=LINE('',#54870,#5406);
#4571=LINE('',#54894,#5407);
#4572=LINE('',#54919,#5408);
#4573=LINE('',#54944,#5409);
#4574=LINE('',#54968,#5410);
#4575=LINE('',#54992,#5411);
#4576=LINE('',#55017,#5412);
#4577=LINE('',#55042,#5413);
#4578=LINE('',#55066,#5414);
#4579=LINE('',#55091,#5415);
#4580=LINE('',#55116,#5416);
#4581=LINE('',#55140,#5417);
#4582=LINE('',#55165,#5418);
#4583=LINE('',#55190,#5419);
#4584=LINE('',#55214,#5420);
#4585=LINE('',#55238,#5421);
#4586=LINE('',#55263,#5422);
#4587=LINE('',#55288,#5423);
#4588=LINE('',#55312,#5424);
#4589=LINE('',#55337,#5425);
#4590=LINE('',#55362,#5426);
#4591=LINE('',#55386,#5427);
#4592=LINE('',#55411,#5428);
#4593=LINE('',#55436,#5429);
#4594=LINE('',#55460,#5430);
#4595=LINE('',#55484,#5431);
#4596=LINE('',#55509,#5432);
#4597=LINE('',#55534,#5433);
#4598=LINE('',#55558,#5434);
#4599=LINE('',#55583,#5435);
#4600=LINE('',#55608,#5436);
#4601=LINE('',#55632,#5437);
#4602=LINE('',#55657,#5438);
#4603=LINE('',#55681,#5439);
#4604=LINE('',#55706,#5440);
#4605=LINE('',#55730,#5441);
#4606=LINE('',#55755,#5442);
#4607=LINE('',#55780,#5443);
#4608=LINE('',#55804,#5444);
#4609=LINE('',#55829,#5445);
#4610=LINE('',#55854,#5446);
#4611=LINE('',#55878,#5447);
#4612=LINE('',#55903,#5448);
#4613=LINE('',#55927,#5449);
#4614=LINE('',#55952,#5450);
#4615=LINE('',#59547,#5451);
#4616=LINE('',#59549,#5452);
#4617=LINE('',#59551,#5453);
#4618=LINE('',#59553,#5454);
#4619=LINE('',#59555,#5455);
#4620=LINE('',#59556,#5456);
#4621=LINE('',#59560,#5457);
#4622=LINE('',#59562,#5458);
#4623=LINE('',#59564,#5459);
#4624=LINE('',#59566,#5460);
#4625=LINE('',#59568,#5461);
#4626=LINE('',#59569,#5462);
#4627=LINE('',#59573,#5463);
#4628=LINE('',#59574,#5464);
#4629=LINE('',#59576,#5465);
#4630=LINE('',#59578,#5466);
#4631=LINE('',#59580,#5467);
#4632=LINE('',#59582,#5468);
#4633=LINE('',#59586,#5469);
#5331=VECTOR('',#17630,5.);
#5332=VECTOR('',#17635,5.);
#5333=VECTOR('',#17638,5.);
#5334=VECTOR('',#17641,5.);
#5335=VECTOR('',#17644,5.);
#5336=VECTOR('',#17647,5.);
#5337=VECTOR('',#17650,5.);
#5338=VECTOR('',#17653,5.);
#5339=VECTOR('',#17656,5.);
#5340=VECTOR('',#17659,5.);
#5341=VECTOR('',#17662,5.);
#5342=VECTOR('',#17665,5.);
#5343=VECTOR('',#17668,5.);
#5344=VECTOR('',#17671,5.);
#5345=VECTOR('',#17674,5.);
#5346=VECTOR('',#17677,5.);
#5347=VECTOR('',#17680,5.);
#5348=VECTOR('',#17683,5.);
#5349=VECTOR('',#17686,5.);
#5350=VECTOR('',#17689,5.);
#5351=VECTOR('',#17692,5.);
#5352=VECTOR('',#17695,5.);
#5353=VECTOR('',#17698,5.);
#5354=VECTOR('',#17701,5.);
#5355=VECTOR('',#17704,5.);
#5356=VECTOR('',#17707,5.);
#5357=VECTOR('',#17710,5.);
#5358=VECTOR('',#17713,5.);
#5359=VECTOR('',#17716,5.);
#5360=VECTOR('',#17719,5.);
#5361=VECTOR('',#17722,5.);
#5362=VECTOR('',#17725,5.);
#5363=VECTOR('',#17728,5.);
#5364=VECTOR('',#17731,5.);
#5365=VECTOR('',#17734,5.);
#5366=VECTOR('',#17737,5.);
#5367=VECTOR('',#17740,5.);
#5368=VECTOR('',#17743,5.);
#5369=VECTOR('',#17746,5.);
#5370=VECTOR('',#17749,5.);
#5371=VECTOR('',#17752,5.);
#5372=VECTOR('',#17755,5.);
#5373=VECTOR('',#17758,5.);
#5374=VECTOR('',#17761,5.);
#5375=VECTOR('',#17764,5.);
#5376=VECTOR('',#17767,5.);
#5377=VECTOR('',#17770,5.);
#5378=VECTOR('',#17773,5.);
#5379=VECTOR('',#17776,5.);
#5380=VECTOR('',#17779,5.);
#5381=VECTOR('',#17782,5.);
#5382=VECTOR('',#17785,5.);
#5383=VECTOR('',#17788,5.);
#5384=VECTOR('',#17791,5.);
#5385=VECTOR('',#17794,5.);
#5386=VECTOR('',#17797,5.);
#5387=VECTOR('',#17800,5.);
#5388=VECTOR('',#17803,5.);
#5389=VECTOR('',#17806,5.);
#5390=VECTOR('',#17809,5.);
#5391=VECTOR('',#17812,4.372);
#5392=VECTOR('',#17817,4.372);
#5393=VECTOR('',#17820,4.372);
#5394=VECTOR('',#17823,4.372);
#5395=VECTOR('',#17826,4.372);
#5396=VECTOR('',#17829,4.372);
#5397=VECTOR('',#17832,4.372);
#5398=VECTOR('',#17835,4.372);
#5399=VECTOR('',#17838,4.372);
#5400=VECTOR('',#17841,4.372);
#5401=VECTOR('',#17844,4.372);
#5402=VECTOR('',#17847,4.372);
#5403=VECTOR('',#17850,4.372);
#5404=VECTOR('',#17853,4.372);
#5405=VECTOR('',#17856,4.372);
#5406=VECTOR('',#17859,4.372);
#5407=VECTOR('',#17862,4.372);
#5408=VECTOR('',#17865,4.372);
#5409=VECTOR('',#17868,4.372);
#5410=VECTOR('',#17871,4.372);
#5411=VECTOR('',#17874,4.372);
#5412=VECTOR('',#17877,4.372);
#5413=VECTOR('',#17880,4.372);
#5414=VECTOR('',#17883,4.372);
#5415=VECTOR('',#17886,4.372);
#5416=VECTOR('',#17889,4.372);
#5417=VECTOR('',#17892,4.372);
#5418=VECTOR('',#17895,4.372);
#5419=VECTOR('',#17898,4.372);
#5420=VECTOR('',#17901,4.372);
#5421=VECTOR('',#17904,4.372);
#5422=VECTOR('',#17907,4.372);
#5423=VECTOR('',#17910,4.372);
#5424=VECTOR('',#17913,4.372);
#5425=VECTOR('',#17916,4.372);
#5426=VECTOR('',#17919,4.372);
#5427=VECTOR('',#17922,4.372);
#5428=VECTOR('',#17925,4.372);
#5429=VECTOR('',#17928,4.372);
#5430=VECTOR('',#17931,4.372);
#5431=VECTOR('',#17934,4.372);
#5432=VECTOR('',#17937,4.372);
#5433=VECTOR('',#17940,4.372);
#5434=VECTOR('',#17943,4.372);
#5435=VECTOR('',#17946,4.372);
#5436=VECTOR('',#17949,4.372);
#5437=VECTOR('',#17952,4.372);
#5438=VECTOR('',#17955,4.372);
#5439=VECTOR('',#17958,4.372);
#5440=VECTOR('',#17961,4.372);
#5441=VECTOR('',#17964,4.372);
#5442=VECTOR('',#17967,4.372);
#5443=VECTOR('',#17970,4.372);
#5444=VECTOR('',#17973,4.372);
#5445=VECTOR('',#17976,4.372);
#5446=VECTOR('',#17979,4.372);
#5447=VECTOR('',#17982,4.372);
#5448=VECTOR('',#17985,4.372);
#5449=VECTOR('',#17988,4.372);
#5450=VECTOR('',#17991,4.372);
#5451=VECTOR('',#18002,10.);
#5452=VECTOR('',#18003,10.);
#5453=VECTOR('',#18004,10.);
#5454=VECTOR('',#18005,10.);
#5455=VECTOR('',#18006,10.);
#5456=VECTOR('',#18007,10.);
#5457=VECTOR('',#18010,10.);
#5458=VECTOR('',#18011,10.);
#5459=VECTOR('',#18012,10.);
#5460=VECTOR('',#18013,10.);
#5461=VECTOR('',#18014,10.);
#5462=VECTOR('',#18015,10.);
#5463=VECTOR('',#18020,10.);
#5464=VECTOR('',#18021,10.);
#5465=VECTOR('',#18024,10.);
#5466=VECTOR('',#18027,10.);
#5467=VECTOR('',#18030,10.);
#5468=VECTOR('',#18033,10.);
#5469=VECTOR('',#18038,5.);
#6579=VERTEX_POINT('',#51547);
#6580=VERTEX_POINT('',#51548);
#6581=VERTEX_POINT('',#51550);
#6582=VERTEX_POINT('',#51561);
#6583=VERTEX_POINT('',#51574);
#6584=VERTEX_POINT('',#51575);
#6585=VERTEX_POINT('',#51622);
#6586=VERTEX_POINT('',#51623);
#6587=VERTEX_POINT('',#51670);
#6588=VERTEX_POINT('',#51671);
#6589=VERTEX_POINT('',#51721);
#6590=VERTEX_POINT('',#51722);
#6591=VERTEX_POINT('',#51769);
#6592=VERTEX_POINT('',#51770);
#6593=VERTEX_POINT('',#51817);
#6594=VERTEX_POINT('',#51818);
#6595=VERTEX_POINT('',#51865);
#6596=VERTEX_POINT('',#51866);
#6597=VERTEX_POINT('',#51919);
#6598=VERTEX_POINT('',#51920);
#6599=VERTEX_POINT('',#51967);
#6600=VERTEX_POINT('',#51968);
#6601=VERTEX_POINT('',#52015);
#6602=VERTEX_POINT('',#52016);
#6603=VERTEX_POINT('',#52069);
#6604=VERTEX_POINT('',#52070);
#6605=VERTEX_POINT('',#52117);
#6606=VERTEX_POINT('',#52118);
#6607=VERTEX_POINT('',#52165);
#6608=VERTEX_POINT('',#52166);
#6609=VERTEX_POINT('',#52216);
#6610=VERTEX_POINT('',#52217);
#6611=VERTEX_POINT('',#52267);
#6612=VERTEX_POINT('',#52268);
#6613=VERTEX_POINT('',#52315);
#6614=VERTEX_POINT('',#52316);
#6615=VERTEX_POINT('',#52363);
#6616=VERTEX_POINT('',#52364);
#6617=VERTEX_POINT('',#52417);
#6618=VERTEX_POINT('',#52418);
#6619=VERTEX_POINT('',#52465);
#6620=VERTEX_POINT('',#52466);
#6621=VERTEX_POINT('',#52513);
#6622=VERTEX_POINT('',#52514);
#6623=VERTEX_POINT('',#52567);
#6624=VERTEX_POINT('',#52568);
#6625=VERTEX_POINT('',#52615);
#6626=VERTEX_POINT('',#52616);
#6627=VERTEX_POINT('',#52663);
#6628=VERTEX_POINT('',#52664);
#6629=VERTEX_POINT('',#52711);
#6630=VERTEX_POINT('',#52712);
#6631=VERTEX_POINT('',#52765);
#6632=VERTEX_POINT('',#52766);
#6633=VERTEX_POINT('',#52813);
#6634=VERTEX_POINT('',#52814);
#6635=VERTEX_POINT('',#52861);
#6636=VERTEX_POINT('',#52862);
#6637=VERTEX_POINT('',#52915);
#6638=VERTEX_POINT('',#52916);
#6639=VERTEX_POINT('',#52963);
#6640=VERTEX_POINT('',#52964);
#6641=VERTEX_POINT('',#53011);
#6642=VERTEX_POINT('',#53012);
#6643=VERTEX_POINT('',#53065);
#6644=VERTEX_POINT('',#53066);
#6645=VERTEX_POINT('',#53113);
#6646=VERTEX_POINT('',#53114);
#6647=VERTEX_POINT('',#53161);
#6648=VERTEX_POINT('',#53162);
#6649=VERTEX_POINT('',#53209);
#6650=VERTEX_POINT('',#53210);
#6651=VERTEX_POINT('',#53263);
#6652=VERTEX_POINT('',#53264);
#6653=VERTEX_POINT('',#53311);
#6654=VERTEX_POINT('',#53312);
#6655=VERTEX_POINT('',#53359);
#6656=VERTEX_POINT('',#53360);
#6657=VERTEX_POINT('',#53413);
#6658=VERTEX_POINT('',#53414);
#6659=VERTEX_POINT('',#53461);
#6660=VERTEX_POINT('',#53462);
#6661=VERTEX_POINT('',#53509);
#6662=VERTEX_POINT('',#53510);
#6663=VERTEX_POINT('',#53563);
#6664=VERTEX_POINT('',#53564);
#6665=VERTEX_POINT('',#53611);
#6666=VERTEX_POINT('',#53612);
#6667=VERTEX_POINT('',#53659);
#6668=VERTEX_POINT('',#53660);
#6669=VERTEX_POINT('',#53707);
#6670=VERTEX_POINT('',#53708);
#6671=VERTEX_POINT('',#53761);
#6672=VERTEX_POINT('',#53762);
#6673=VERTEX_POINT('',#53809);
#6674=VERTEX_POINT('',#53810);
#6675=VERTEX_POINT('',#53857);
#6676=VERTEX_POINT('',#53858);
#6677=VERTEX_POINT('',#53911);
#6678=VERTEX_POINT('',#53912);
#6679=VERTEX_POINT('',#53959);
#6680=VERTEX_POINT('',#53960);
#6681=VERTEX_POINT('',#54007);
#6682=VERTEX_POINT('',#54008);
#6683=VERTEX_POINT('',#54061);
#6684=VERTEX_POINT('',#54062);
#6685=VERTEX_POINT('',#54109);
#6686=VERTEX_POINT('',#54110);
#6687=VERTEX_POINT('',#54157);
#6688=VERTEX_POINT('',#54158);
#6689=VERTEX_POINT('',#54205);
#6690=VERTEX_POINT('',#54206);
#6691=VERTEX_POINT('',#54259);
#6692=VERTEX_POINT('',#54260);
#6693=VERTEX_POINT('',#54307);
#6694=VERTEX_POINT('',#54308);
#6695=VERTEX_POINT('',#54355);
#6696=VERTEX_POINT('',#54356);
#6697=VERTEX_POINT('',#54409);
#6698=VERTEX_POINT('',#54410);
#6699=VERTEX_POINT('',#54457);
#6700=VERTEX_POINT('',#54458);
#6701=VERTEX_POINT('',#54505);
#6702=VERTEX_POINT('',#54506);
#6703=VERTEX_POINT('',#54508);
#6704=VERTEX_POINT('',#54515);
#6705=VERTEX_POINT('',#54523);
#6706=VERTEX_POINT('',#54524);
#6707=VERTEX_POINT('',#54548);
#6708=VERTEX_POINT('',#54549);
#6709=VERTEX_POINT('',#54572);
#6710=VERTEX_POINT('',#54573);
#6711=VERTEX_POINT('',#54597);
#6712=VERTEX_POINT('',#54598);
#6713=VERTEX_POINT('',#54622);
#6714=VERTEX_POINT('',#54623);
#6715=VERTEX_POINT('',#54646);
#6716=VERTEX_POINT('',#54647);
#6717=VERTEX_POINT('',#54671);
#6718=VERTEX_POINT('',#54672);
#6719=VERTEX_POINT('',#54696);
#6720=VERTEX_POINT('',#54697);
#6721=VERTEX_POINT('',#54720);
#6722=VERTEX_POINT('',#54721);
#6723=VERTEX_POINT('',#54744);
#6724=VERTEX_POINT('',#54745);
#6725=VERTEX_POINT('',#54769);
#6726=VERTEX_POINT('',#54770);
#6727=VERTEX_POINT('',#54794);
#6728=VERTEX_POINT('',#54795);
#6729=VERTEX_POINT('',#54818);
#6730=VERTEX_POINT('',#54819);
#6731=VERTEX_POINT('',#54843);
#6732=VERTEX_POINT('',#54844);
#6733=VERTEX_POINT('',#54868);
#6734=VERTEX_POINT('',#54869);
#6735=VERTEX_POINT('',#54892);
#6736=VERTEX_POINT('',#54893);
#6737=VERTEX_POINT('',#54917);
#6738=VERTEX_POINT('',#54918);
#6739=VERTEX_POINT('',#54942);
#6740=VERTEX_POINT('',#54943);
#6741=VERTEX_POINT('',#54966);
#6742=VERTEX_POINT('',#54967);
#6743=VERTEX_POINT('',#54990);
#6744=VERTEX_POINT('',#54991);
#6745=VERTEX_POINT('',#55015);
#6746=VERTEX_POINT('',#55016);
#6747=VERTEX_POINT('',#55040);
#6748=VERTEX_POINT('',#55041);
#6749=VERTEX_POINT('',#55064);
#6750=VERTEX_POINT('',#55065);
#6751=VERTEX_POINT('',#55089);
#6752=VERTEX_POINT('',#55090);
#6753=VERTEX_POINT('',#55114);
#6754=VERTEX_POINT('',#55115);
#6755=VERTEX_POINT('',#55138);
#6756=VERTEX_POINT('',#55139);
#6757=VERTEX_POINT('',#55163);
#6758=VERTEX_POINT('',#55164);
#6759=VERTEX_POINT('',#55188);
#6760=VERTEX_POINT('',#55189);
#6761=VERTEX_POINT('',#55212);
#6762=VERTEX_POINT('',#55213);
#6763=VERTEX_POINT('',#55236);
#6764=VERTEX_POINT('',#55237);
#6765=VERTEX_POINT('',#55261);
#6766=VERTEX_POINT('',#55262);
#6767=VERTEX_POINT('',#55286);
#6768=VERTEX_POINT('',#55287);
#6769=VERTEX_POINT('',#55310);
#6770=VERTEX_POINT('',#55311);
#6771=VERTEX_POINT('',#55335);
#6772=VERTEX_POINT('',#55336);
#6773=VERTEX_POINT('',#55360);
#6774=VERTEX_POINT('',#55361);
#6775=VERTEX_POINT('',#55384);
#6776=VERTEX_POINT('',#55385);
#6777=VERTEX_POINT('',#55409);
#6778=VERTEX_POINT('',#55410);
#6779=VERTEX_POINT('',#55434);
#6780=VERTEX_POINT('',#55435);
#6781=VERTEX_POINT('',#55458);
#6782=VERTEX_POINT('',#55459);
#6783=VERTEX_POINT('',#55482);
#6784=VERTEX_POINT('',#55483);
#6785=VERTEX_POINT('',#55507);
#6786=VERTEX_POINT('',#55508);
#6787=VERTEX_POINT('',#55532);
#6788=VERTEX_POINT('',#55533);
#6789=VERTEX_POINT('',#55556);
#6790=VERTEX_POINT('',#55557);
#6791=VERTEX_POINT('',#55581);
#6792=VERTEX_POINT('',#55582);
#6793=VERTEX_POINT('',#55606);
#6794=VERTEX_POINT('',#55607);
#6795=VERTEX_POINT('',#55630);
#6796=VERTEX_POINT('',#55631);
#6797=VERTEX_POINT('',#55655);
#6798=VERTEX_POINT('',#55656);
#6799=VERTEX_POINT('',#55679);
#6800=VERTEX_POINT('',#55680);
#6801=VERTEX_POINT('',#55704);
#6802=VERTEX_POINT('',#55705);
#6803=VERTEX_POINT('',#55728);
#6804=VERTEX_POINT('',#55729);
#6805=VERTEX_POINT('',#55753);
#6806=VERTEX_POINT('',#55754);
#6807=VERTEX_POINT('',#55778);
#6808=VERTEX_POINT('',#55779);
#6809=VERTEX_POINT('',#55802);
#6810=VERTEX_POINT('',#55803);
#6811=VERTEX_POINT('',#55827);
#6812=VERTEX_POINT('',#55828);
#6813=VERTEX_POINT('',#55852);
#6814=VERTEX_POINT('',#55853);
#6815=VERTEX_POINT('',#55876);
#6816=VERTEX_POINT('',#55877);
#6817=VERTEX_POINT('',#55901);
#6818=VERTEX_POINT('',#55902);
#6819=VERTEX_POINT('',#55925);
#6820=VERTEX_POINT('',#55926);
#6821=VERTEX_POINT('',#55950);
#6822=VERTEX_POINT('',#55951);
#6823=VERTEX_POINT('',#57513);
#6824=VERTEX_POINT('',#57642);
#6825=VERTEX_POINT('',#57759);
#6826=VERTEX_POINT('',#59310);
#6827=VERTEX_POINT('',#59545);
#6828=VERTEX_POINT('',#59546);
#6829=VERTEX_POINT('',#59548);
#6830=VERTEX_POINT('',#59550);
#6831=VERTEX_POINT('',#59552);
#6832=VERTEX_POINT('',#59554);
#6833=VERTEX_POINT('',#59558);
#6834=VERTEX_POINT('',#59559);
#6835=VERTEX_POINT('',#59561);
#6836=VERTEX_POINT('',#59563);
#6837=VERTEX_POINT('',#59565);
#6838=VERTEX_POINT('',#59567);
#6839=VERTEX_POINT('',#59570);
#6840=VERTEX_POINT('',#59585);
#6841=VERTEX_POINT('',#59590);
#8517=EDGE_CURVE('',#6579,#6580,#4495,.T.);
#8518=EDGE_CURVE('',#6579,#6581,#1233,.T.);
#8519=EDGE_CURVE('',#6581,#6582,#461,.F.);
#8520=EDGE_CURVE('',#6582,#6580,#1234,.T.);
#8521=EDGE_CURVE('',#6583,#6584,#4496,.T.);
#8522=EDGE_CURVE('',#6583,#6579,#1235,.T.);
#8523=EDGE_CURVE('',#6580,#6584,#1236,.T.);
#8524=EDGE_CURVE('',#6585,#6586,#4497,.T.);
#8525=EDGE_CURVE('',#6585,#6583,#1237,.T.);
#8526=EDGE_CURVE('',#6584,#6586,#1238,.T.);
#8527=EDGE_CURVE('',#6587,#6588,#4498,.T.);
#8528=EDGE_CURVE('',#6587,#6585,#1239,.T.);
#8529=EDGE_CURVE('',#6586,#6588,#1240,.T.);
#8530=EDGE_CURVE('',#6589,#6590,#4499,.T.);
#8531=EDGE_CURVE('',#6589,#6587,#1241,.T.);
#8532=EDGE_CURVE('',#6588,#6590,#1242,.T.);
#8533=EDGE_CURVE('',#6591,#6592,#4500,.T.);
#8534=EDGE_CURVE('',#6591,#6589,#1243,.T.);
#8535=EDGE_CURVE('',#6590,#6592,#1244,.T.);
#8536=EDGE_CURVE('',#6593,#6594,#4501,.T.);
#8537=EDGE_CURVE('',#6593,#6591,#1245,.T.);
#8538=EDGE_CURVE('',#6592,#6594,#1246,.T.);
#8539=EDGE_CURVE('',#6595,#6596,#4502,.T.);
#8540=EDGE_CURVE('',#6595,#6593,#1247,.T.);
#8541=EDGE_CURVE('',#6594,#6596,#1248,.T.);
#8542=EDGE_CURVE('',#6597,#6598,#4503,.T.);
#8543=EDGE_CURVE('',#6597,#6595,#1249,.T.);
#8544=EDGE_CURVE('',#6596,#6598,#1250,.T.);
#8545=EDGE_CURVE('',#6599,#6600,#4504,.T.);
#8546=EDGE_CURVE('',#6599,#6597,#1251,.T.);
#8547=EDGE_CURVE('',#6598,#6600,#1252,.T.);
#8548=EDGE_CURVE('',#6601,#6602,#4505,.T.);
#8549=EDGE_CURVE('',#6601,#6599,#1253,.T.);
#8550=EDGE_CURVE('',#6600,#6602,#1254,.T.);
#8551=EDGE_CURVE('',#6603,#6604,#4506,.T.);
#8552=EDGE_CURVE('',#6603,#6601,#1255,.T.);
#8553=EDGE_CURVE('',#6602,#6604,#1256,.T.);
#8554=EDGE_CURVE('',#6605,#6606,#4507,.T.);
#8555=EDGE_CURVE('',#6605,#6603,#1257,.T.);
#8556=EDGE_CURVE('',#6604,#6606,#1258,.T.);
#8557=EDGE_CURVE('',#6607,#6608,#4508,.T.);
#8558=EDGE_CURVE('',#6607,#6605,#1259,.T.);
#8559=EDGE_CURVE('',#6606,#6608,#1260,.T.);
#8560=EDGE_CURVE('',#6609,#6610,#4509,.T.);
#8561=EDGE_CURVE('',#6609,#6607,#1261,.T.);
#8562=EDGE_CURVE('',#6608,#6610,#1262,.T.);
#8563=EDGE_CURVE('',#6611,#6612,#4510,.T.);
#8564=EDGE_CURVE('',#6611,#6609,#1263,.T.);
#8565=EDGE_CURVE('',#6610,#6612,#1264,.T.);
#8566=EDGE_CURVE('',#6613,#6614,#4511,.T.);
#8567=EDGE_CURVE('',#6613,#6611,#1265,.T.);
#8568=EDGE_CURVE('',#6612,#6614,#1266,.T.);
#8569=EDGE_CURVE('',#6615,#6616,#4512,.T.);
#8570=EDGE_CURVE('',#6615,#6613,#1267,.T.);
#8571=EDGE_CURVE('',#6614,#6616,#1268,.T.);
#8572=EDGE_CURVE('',#6617,#6618,#4513,.T.);
#8573=EDGE_CURVE('',#6617,#6615,#1269,.T.);
#8574=EDGE_CURVE('',#6616,#6618,#1270,.T.);
#8575=EDGE_CURVE('',#6619,#6620,#4514,.T.);
#8576=EDGE_CURVE('',#6619,#6617,#1271,.T.);
#8577=EDGE_CURVE('',#6618,#6620,#1272,.T.);
#8578=EDGE_CURVE('',#6621,#6622,#4515,.T.);
#8579=EDGE_CURVE('',#6621,#6619,#1273,.T.);
#8580=EDGE_CURVE('',#6620,#6622,#1274,.T.);
#8581=EDGE_CURVE('',#6623,#6624,#4516,.T.);
#8582=EDGE_CURVE('',#6623,#6621,#1275,.T.);
#8583=EDGE_CURVE('',#6622,#6624,#1276,.T.);
#8584=EDGE_CURVE('',#6625,#6626,#4517,.T.);
#8585=EDGE_CURVE('',#6625,#6623,#1277,.T.);
#8586=EDGE_CURVE('',#6624,#6626,#1278,.T.);
#8587=EDGE_CURVE('',#6627,#6628,#4518,.T.);
#8588=EDGE_CURVE('',#6627,#6625,#1279,.T.);
#8589=EDGE_CURVE('',#6626,#6628,#1280,.T.);
#8590=EDGE_CURVE('',#6629,#6630,#4519,.T.);
#8591=EDGE_CURVE('',#6629,#6627,#1281,.T.);
#8592=EDGE_CURVE('',#6628,#6630,#1282,.T.);
#8593=EDGE_CURVE('',#6631,#6632,#4520,.T.);
#8594=EDGE_CURVE('',#6631,#6629,#1283,.T.);
#8595=EDGE_CURVE('',#6630,#6632,#1284,.T.);
#8596=EDGE_CURVE('',#6633,#6634,#4521,.T.);
#8597=EDGE_CURVE('',#6633,#6631,#1285,.T.);
#8598=EDGE_CURVE('',#6632,#6634,#1286,.T.);
#8599=EDGE_CURVE('',#6635,#6636,#4522,.T.);
#8600=EDGE_CURVE('',#6635,#6633,#1287,.T.);
#8601=EDGE_CURVE('',#6634,#6636,#1288,.T.);
#8602=EDGE_CURVE('',#6637,#6638,#4523,.T.);
#8603=EDGE_CURVE('',#6637,#6635,#1289,.T.);
#8604=EDGE_CURVE('',#6636,#6638,#1290,.T.);
#8605=EDGE_CURVE('',#6639,#6640,#4524,.T.);
#8606=EDGE_CURVE('',#6639,#6637,#1291,.T.);
#8607=EDGE_CURVE('',#6638,#6640,#1292,.T.);
#8608=EDGE_CURVE('',#6641,#6642,#4525,.T.);
#8609=EDGE_CURVE('',#6641,#6639,#1293,.T.);
#8610=EDGE_CURVE('',#6640,#6642,#1294,.T.);
#8611=EDGE_CURVE('',#6643,#6644,#4526,.T.);
#8612=EDGE_CURVE('',#6643,#6641,#1295,.T.);
#8613=EDGE_CURVE('',#6642,#6644,#1296,.T.);
#8614=EDGE_CURVE('',#6645,#6646,#4527,.T.);
#8615=EDGE_CURVE('',#6645,#6643,#1297,.T.);
#8616=EDGE_CURVE('',#6644,#6646,#1298,.T.);
#8617=EDGE_CURVE('',#6647,#6648,#4528,.T.);
#8618=EDGE_CURVE('',#6647,#6645,#1299,.T.);
#8619=EDGE_CURVE('',#6646,#6648,#1300,.T.);
#8620=EDGE_CURVE('',#6649,#6650,#4529,.T.);
#8621=EDGE_CURVE('',#6649,#6647,#1301,.T.);
#8622=EDGE_CURVE('',#6648,#6650,#1302,.T.);
#8623=EDGE_CURVE('',#6651,#6652,#4530,.T.);
#8624=EDGE_CURVE('',#6651,#6649,#1303,.T.);
#8625=EDGE_CURVE('',#6650,#6652,#1304,.T.);
#8626=EDGE_CURVE('',#6653,#6654,#4531,.T.);
#8627=EDGE_CURVE('',#6653,#6651,#1305,.T.);
#8628=EDGE_CURVE('',#6652,#6654,#1306,.T.);
#8629=EDGE_CURVE('',#6655,#6656,#4532,.T.);
#8630=EDGE_CURVE('',#6655,#6653,#1307,.T.);
#8631=EDGE_CURVE('',#6654,#6656,#1308,.T.);
#8632=EDGE_CURVE('',#6657,#6658,#4533,.T.);
#8633=EDGE_CURVE('',#6657,#6655,#1309,.T.);
#8634=EDGE_CURVE('',#6656,#6658,#1310,.T.);
#8635=EDGE_CURVE('',#6659,#6660,#4534,.T.);
#8636=EDGE_CURVE('',#6659,#6657,#1311,.T.);
#8637=EDGE_CURVE('',#6658,#6660,#1312,.T.);
#8638=EDGE_CURVE('',#6661,#6662,#4535,.T.);
#8639=EDGE_CURVE('',#6661,#6659,#1313,.T.);
#8640=EDGE_CURVE('',#6660,#6662,#1314,.T.);
#8641=EDGE_CURVE('',#6663,#6664,#4536,.T.);
#8642=EDGE_CURVE('',#6663,#6661,#1315,.T.);
#8643=EDGE_CURVE('',#6662,#6664,#1316,.T.);
#8644=EDGE_CURVE('',#6665,#6666,#4537,.T.);
#8645=EDGE_CURVE('',#6665,#6663,#1317,.T.);
#8646=EDGE_CURVE('',#6664,#6666,#1318,.T.);
#8647=EDGE_CURVE('',#6667,#6668,#4538,.T.);
#8648=EDGE_CURVE('',#6667,#6665,#1319,.T.);
#8649=EDGE_CURVE('',#6666,#6668,#1320,.T.);
#8650=EDGE_CURVE('',#6669,#6670,#4539,.T.);
#8651=EDGE_CURVE('',#6669,#6667,#1321,.T.);
#8652=EDGE_CURVE('',#6668,#6670,#1322,.T.);
#8653=EDGE_CURVE('',#6671,#6672,#4540,.T.);
#8654=EDGE_CURVE('',#6671,#6669,#1323,.T.);
#8655=EDGE_CURVE('',#6670,#6672,#1324,.T.);
#8656=EDGE_CURVE('',#6673,#6674,#4541,.T.);
#8657=EDGE_CURVE('',#6673,#6671,#1325,.T.);
#8658=EDGE_CURVE('',#6672,#6674,#1326,.T.);
#8659=EDGE_CURVE('',#6675,#6676,#4542,.T.);
#8660=EDGE_CURVE('',#6675,#6673,#1327,.T.);
#8661=EDGE_CURVE('',#6674,#6676,#1328,.T.);
#8662=EDGE_CURVE('',#6677,#6678,#4543,.T.);
#8663=EDGE_CURVE('',#6677,#6675,#1329,.T.);
#8664=EDGE_CURVE('',#6676,#6678,#1330,.T.);
#8665=EDGE_CURVE('',#6679,#6680,#4544,.T.);
#8666=EDGE_CURVE('',#6679,#6677,#1331,.T.);
#8667=EDGE_CURVE('',#6678,#6680,#1332,.T.);
#8668=EDGE_CURVE('',#6681,#6682,#4545,.T.);
#8669=EDGE_CURVE('',#6681,#6679,#1333,.T.);
#8670=EDGE_CURVE('',#6680,#6682,#1334,.T.);
#8671=EDGE_CURVE('',#6683,#6684,#4546,.T.);
#8672=EDGE_CURVE('',#6683,#6681,#1335,.T.);
#8673=EDGE_CURVE('',#6682,#6684,#1336,.T.);
#8674=EDGE_CURVE('',#6685,#6686,#4547,.T.);
#8675=EDGE_CURVE('',#6685,#6683,#1337,.T.);
#8676=EDGE_CURVE('',#6684,#6686,#1338,.T.);
#8677=EDGE_CURVE('',#6687,#6688,#4548,.T.);
#8678=EDGE_CURVE('',#6687,#6685,#1339,.T.);
#8679=EDGE_CURVE('',#6686,#6688,#1340,.T.);
#8680=EDGE_CURVE('',#6689,#6690,#4549,.T.);
#8681=EDGE_CURVE('',#6689,#6687,#1341,.T.);
#8682=EDGE_CURVE('',#6688,#6690,#1342,.T.);
#8683=EDGE_CURVE('',#6691,#6692,#4550,.T.);
#8684=EDGE_CURVE('',#6691,#6689,#1343,.T.);
#8685=EDGE_CURVE('',#6690,#6692,#1344,.T.);
#8686=EDGE_CURVE('',#6693,#6694,#4551,.T.);
#8687=EDGE_CURVE('',#6693,#6691,#1345,.T.);
#8688=EDGE_CURVE('',#6692,#6694,#1346,.T.);
#8689=EDGE_CURVE('',#6695,#6696,#4552,.T.);
#8690=EDGE_CURVE('',#6695,#6693,#1347,.T.);
#8691=EDGE_CURVE('',#6694,#6696,#1348,.T.);
#8692=EDGE_CURVE('',#6697,#6698,#4553,.T.);
#8693=EDGE_CURVE('',#6697,#6695,#1349,.T.);
#8694=EDGE_CURVE('',#6696,#6698,#1350,.T.);
#8695=EDGE_CURVE('',#6699,#6700,#4554,.T.);
#8696=EDGE_CURVE('',#6699,#6697,#1351,.T.);
#8697=EDGE_CURVE('',#6698,#6700,#1352,.T.);
#8698=EDGE_CURVE('',#6701,#6702,#4555,.T.);
#8699=EDGE_CURVE('',#6701,#6703,#1353,.T.);
#8700=EDGE_CURVE('',#6704,#6703,#462,.T.);
#8701=EDGE_CURVE('',#6702,#6704,#1354,.T.);
#8702=EDGE_CURVE('',#6705,#6706,#4556,.T.);
#8703=EDGE_CURVE('',#6705,#6701,#1355,.T.);
#8704=EDGE_CURVE('',#6706,#6702,#1356,.T.);
#8705=EDGE_CURVE('',#6707,#6708,#4557,.T.);
#8706=EDGE_CURVE('',#6707,#6705,#1357,.T.);
#8707=EDGE_CURVE('',#6708,#6706,#1358,.T.);
#8708=EDGE_CURVE('',#6709,#6710,#4558,.T.);
#8709=EDGE_CURVE('',#6709,#6707,#1359,.T.);
#8710=EDGE_CURVE('',#6710,#6708,#1360,.T.);
#8711=EDGE_CURVE('',#6711,#6712,#4559,.T.);
#8712=EDGE_CURVE('',#6711,#6709,#1361,.T.);
#8713=EDGE_CURVE('',#6712,#6710,#1362,.T.);
#8714=EDGE_CURVE('',#6713,#6714,#4560,.T.);
#8715=EDGE_CURVE('',#6713,#6711,#1363,.T.);
#8716=EDGE_CURVE('',#6714,#6712,#1364,.T.);
#8717=EDGE_CURVE('',#6715,#6716,#4561,.T.);
#8718=EDGE_CURVE('',#6715,#6713,#1365,.T.);
#8719=EDGE_CURVE('',#6716,#6714,#1366,.T.);
#8720=EDGE_CURVE('',#6717,#6718,#4562,.T.);
#8721=EDGE_CURVE('',#6717,#6715,#1367,.T.);
#8722=EDGE_CURVE('',#6718,#6716,#1368,.T.);
#8723=EDGE_CURVE('',#6719,#6720,#4563,.T.);
#8724=EDGE_CURVE('',#6719,#6717,#1369,.T.);
#8725=EDGE_CURVE('',#6720,#6718,#1370,.T.);
#8726=EDGE_CURVE('',#6721,#6722,#4564,.T.);
#8727=EDGE_CURVE('',#6721,#6719,#1371,.T.);
#8728=EDGE_CURVE('',#6722,#6720,#1372,.T.);
#8729=EDGE_CURVE('',#6723,#6724,#4565,.T.);
#8730=EDGE_CURVE('',#6723,#6721,#1373,.T.);
#8731=EDGE_CURVE('',#6724,#6722,#1374,.T.);
#8732=EDGE_CURVE('',#6725,#6726,#4566,.T.);
#8733=EDGE_CURVE('',#6725,#6723,#1375,.T.);
#8734=EDGE_CURVE('',#6726,#6724,#1376,.T.);
#8735=EDGE_CURVE('',#6727,#6728,#4567,.T.);
#8736=EDGE_CURVE('',#6727,#6725,#1377,.T.);
#8737=EDGE_CURVE('',#6728,#6726,#1378,.T.);
#8738=EDGE_CURVE('',#6729,#6730,#4568,.T.);
#8739=EDGE_CURVE('',#6729,#6727,#1379,.T.);
#8740=EDGE_CURVE('',#6730,#6728,#1380,.T.);
#8741=EDGE_CURVE('',#6731,#6732,#4569,.T.);
#8742=EDGE_CURVE('',#6731,#6729,#1381,.T.);
#8743=EDGE_CURVE('',#6732,#6730,#1382,.T.);
#8744=EDGE_CURVE('',#6733,#6734,#4570,.T.);
#8745=EDGE_CURVE('',#6733,#6731,#1383,.T.);
#8746=EDGE_CURVE('',#6734,#6732,#1384,.T.);
#8747=EDGE_CURVE('',#6735,#6736,#4571,.T.);
#8748=EDGE_CURVE('',#6735,#6733,#1385,.T.);
#8749=EDGE_CURVE('',#6736,#6734,#1386,.T.);
#8750=EDGE_CURVE('',#6737,#6738,#4572,.T.);
#8751=EDGE_CURVE('',#6737,#6735,#1387,.T.);
#8752=EDGE_CURVE('',#6738,#6736,#1388,.T.);
#8753=EDGE_CURVE('',#6739,#6740,#4573,.T.);
#8754=EDGE_CURVE('',#6739,#6737,#1389,.T.);
#8755=EDGE_CURVE('',#6740,#6738,#1390,.T.);
#8756=EDGE_CURVE('',#6741,#6742,#4574,.T.);
#8757=EDGE_CURVE('',#6741,#6739,#1391,.T.);
#8758=EDGE_CURVE('',#6742,#6740,#1392,.T.);
#8759=EDGE_CURVE('',#6743,#6744,#4575,.T.);
#8760=EDGE_CURVE('',#6743,#6741,#1393,.T.);
#8761=EDGE_CURVE('',#6744,#6742,#1394,.T.);
#8762=EDGE_CURVE('',#6745,#6746,#4576,.T.);
#8763=EDGE_CURVE('',#6745,#6743,#1395,.T.);
#8764=EDGE_CURVE('',#6746,#6744,#1396,.T.);
#8765=EDGE_CURVE('',#6747,#6748,#4577,.T.);
#8766=EDGE_CURVE('',#6747,#6745,#1397,.T.);
#8767=EDGE_CURVE('',#6748,#6746,#1398,.T.);
#8768=EDGE_CURVE('',#6749,#6750,#4578,.T.);
#8769=EDGE_CURVE('',#6749,#6747,#1399,.T.);
#8770=EDGE_CURVE('',#6750,#6748,#1400,.T.);
#8771=EDGE_CURVE('',#6751,#6752,#4579,.T.);
#8772=EDGE_CURVE('',#6751,#6749,#1401,.T.);
#8773=EDGE_CURVE('',#6752,#6750,#1402,.T.);
#8774=EDGE_CURVE('',#6753,#6754,#4580,.T.);
#8775=EDGE_CURVE('',#6753,#6751,#1403,.T.);
#8776=EDGE_CURVE('',#6754,#6752,#1404,.T.);
#8777=EDGE_CURVE('',#6755,#6756,#4581,.T.);
#8778=EDGE_CURVE('',#6755,#6753,#1405,.T.);
#8779=EDGE_CURVE('',#6756,#6754,#1406,.T.);
#8780=EDGE_CURVE('',#6757,#6758,#4582,.T.);
#8781=EDGE_CURVE('',#6757,#6755,#1407,.T.);
#8782=EDGE_CURVE('',#6758,#6756,#1408,.T.);
#8783=EDGE_CURVE('',#6759,#6760,#4583,.T.);
#8784=EDGE_CURVE('',#6759,#6757,#1409,.T.);
#8785=EDGE_CURVE('',#6760,#6758,#1410,.T.);
#8786=EDGE_CURVE('',#6761,#6762,#4584,.T.);
#8787=EDGE_CURVE('',#6761,#6759,#1411,.T.);
#8788=EDGE_CURVE('',#6762,#6760,#1412,.T.);
#8789=EDGE_CURVE('',#6763,#6764,#4585,.T.);
#8790=EDGE_CURVE('',#6763,#6761,#1413,.T.);
#8791=EDGE_CURVE('',#6764,#6762,#1414,.T.);
#8792=EDGE_CURVE('',#6765,#6766,#4586,.T.);
#8793=EDGE_CURVE('',#6765,#6763,#1415,.T.);
#8794=EDGE_CURVE('',#6766,#6764,#1416,.T.);
#8795=EDGE_CURVE('',#6767,#6768,#4587,.T.);
#8796=EDGE_CURVE('',#6767,#6765,#1417,.T.);
#8797=EDGE_CURVE('',#6768,#6766,#1418,.T.);
#8798=EDGE_CURVE('',#6769,#6770,#4588,.T.);
#8799=EDGE_CURVE('',#6769,#6767,#1419,.T.);
#8800=EDGE_CURVE('',#6770,#6768,#1420,.T.);
#8801=EDGE_CURVE('',#6771,#6772,#4589,.T.);
#8802=EDGE_CURVE('',#6771,#6769,#1421,.T.);
#8803=EDGE_CURVE('',#6772,#6770,#1422,.T.);
#8804=EDGE_CURVE('',#6773,#6774,#4590,.T.);
#8805=EDGE_CURVE('',#6773,#6771,#1423,.T.);
#8806=EDGE_CURVE('',#6774,#6772,#1424,.T.);
#8807=EDGE_CURVE('',#6775,#6776,#4591,.T.);
#8808=EDGE_CURVE('',#6775,#6773,#1425,.T.);
#8809=EDGE_CURVE('',#6776,#6774,#1426,.T.);
#8810=EDGE_CURVE('',#6777,#6778,#4592,.T.);
#8811=EDGE_CURVE('',#6777,#6775,#1427,.T.);
#8812=EDGE_CURVE('',#6778,#6776,#1428,.T.);
#8813=EDGE_CURVE('',#6779,#6780,#4593,.T.);
#8814=EDGE_CURVE('',#6779,#6777,#1429,.T.);
#8815=EDGE_CURVE('',#6780,#6778,#1430,.T.);
#8816=EDGE_CURVE('',#6781,#6782,#4594,.T.);
#8817=EDGE_CURVE('',#6781,#6779,#1431,.T.);
#8818=EDGE_CURVE('',#6782,#6780,#1432,.T.);
#8819=EDGE_CURVE('',#6783,#6784,#4595,.T.);
#8820=EDGE_CURVE('',#6783,#6781,#1433,.T.);
#8821=EDGE_CURVE('',#6784,#6782,#1434,.T.);
#8822=EDGE_CURVE('',#6785,#6786,#4596,.T.);
#8823=EDGE_CURVE('',#6785,#6783,#1435,.T.);
#8824=EDGE_CURVE('',#6786,#6784,#1436,.T.);
#8825=EDGE_CURVE('',#6787,#6788,#4597,.T.);
#8826=EDGE_CURVE('',#6787,#6785,#1437,.T.);
#8827=EDGE_CURVE('',#6788,#6786,#1438,.T.);
#8828=EDGE_CURVE('',#6789,#6790,#4598,.T.);
#8829=EDGE_CURVE('',#6789,#6787,#1439,.T.);
#8830=EDGE_CURVE('',#6790,#6788,#1440,.T.);
#8831=EDGE_CURVE('',#6791,#6792,#4599,.T.);
#8832=EDGE_CURVE('',#6791,#6789,#1441,.T.);
#8833=EDGE_CURVE('',#6792,#6790,#1442,.T.);
#8834=EDGE_CURVE('',#6793,#6794,#4600,.T.);
#8835=EDGE_CURVE('',#6793,#6791,#1443,.T.);
#8836=EDGE_CURVE('',#6794,#6792,#1444,.T.);
#8837=EDGE_CURVE('',#6795,#6796,#4601,.T.);
#8838=EDGE_CURVE('',#6795,#6793,#1445,.T.);
#8839=EDGE_CURVE('',#6796,#6794,#1446,.T.);
#8840=EDGE_CURVE('',#6797,#6798,#4602,.T.);
#8841=EDGE_CURVE('',#6797,#6795,#1447,.T.);
#8842=EDGE_CURVE('',#6798,#6796,#1448,.T.);
#8843=EDGE_CURVE('',#6799,#6800,#4603,.T.);
#8844=EDGE_CURVE('',#6799,#6797,#1449,.T.);
#8845=EDGE_CURVE('',#6800,#6798,#1450,.T.);
#8846=EDGE_CURVE('',#6801,#6802,#4604,.T.);
#8847=EDGE_CURVE('',#6801,#6799,#1451,.T.);
#8848=EDGE_CURVE('',#6802,#6800,#1452,.T.);
#8849=EDGE_CURVE('',#6803,#6804,#4605,.T.);
#8850=EDGE_CURVE('',#6803,#6801,#1453,.T.);
#8851=EDGE_CURVE('',#6804,#6802,#1454,.T.);
#8852=EDGE_CURVE('',#6805,#6806,#4606,.T.);
#8853=EDGE_CURVE('',#6805,#6803,#1455,.T.);
#8854=EDGE_CURVE('',#6806,#6804,#1456,.T.);
#8855=EDGE_CURVE('',#6807,#6808,#4607,.T.);
#8856=EDGE_CURVE('',#6807,#6805,#1457,.T.);
#8857=EDGE_CURVE('',#6808,#6806,#1458,.T.);
#8858=EDGE_CURVE('',#6809,#6810,#4608,.T.);
#8859=EDGE_CURVE('',#6809,#6807,#1459,.T.);
#8860=EDGE_CURVE('',#6810,#6808,#1460,.T.);
#8861=EDGE_CURVE('',#6811,#6812,#4609,.T.);
#8862=EDGE_CURVE('',#6811,#6809,#1461,.T.);
#8863=EDGE_CURVE('',#6812,#6810,#1462,.T.);
#8864=EDGE_CURVE('',#6813,#6814,#4610,.T.);
#8865=EDGE_CURVE('',#6813,#6811,#1463,.T.);
#8866=EDGE_CURVE('',#6814,#6812,#1464,.T.);
#8867=EDGE_CURVE('',#6815,#6816,#4611,.T.);
#8868=EDGE_CURVE('',#6815,#6813,#1465,.T.);
#8869=EDGE_CURVE('',#6816,#6814,#1466,.T.);
#8870=EDGE_CURVE('',#6817,#6818,#4612,.T.);
#8871=EDGE_CURVE('',#6817,#6815,#1467,.T.);
#8872=EDGE_CURVE('',#6818,#6816,#1468,.T.);
#8873=EDGE_CURVE('',#6819,#6820,#4613,.T.);
#8874=EDGE_CURVE('',#6819,#6817,#1469,.T.);
#8875=EDGE_CURVE('',#6820,#6818,#1470,.T.);
#8876=EDGE_CURVE('',#6821,#6822,#4614,.T.);
#8877=EDGE_CURVE('',#6821,#6819,#1471,.T.);
#8878=EDGE_CURVE('',#6822,#6820,#1472,.T.);
#8879=EDGE_CURVE('',#6823,#6704,#1473,.T.);
#8880=EDGE_CURVE('',#6700,#6823,#1474,.T.);
#8881=EDGE_CURVE('',#6824,#6582,#1475,.T.);
#8882=EDGE_CURVE('',#6824,#6822,#1476,.T.);
#8883=EDGE_CURVE('',#6825,#6824,#463,.T.);
#8884=EDGE_CURVE('',#6825,#6821,#1477,.T.);
#8885=EDGE_CURVE('',#6703,#6826,#1478,.T.);
#8886=EDGE_CURVE('',#6581,#6825,#1479,.T.);
#8887=EDGE_CURVE('',#6826,#6699,#1480,.T.);
#8888=EDGE_CURVE('',#6826,#6823,#464,.F.);
#8889=EDGE_CURVE('',#6827,#6828,#4615,.T.);
#8890=EDGE_CURVE('',#6828,#6829,#4616,.T.);
#8891=EDGE_CURVE('',#6829,#6830,#4617,.T.);
#8892=EDGE_CURVE('',#6830,#6831,#4618,.T.);
#8893=EDGE_CURVE('',#6831,#6832,#4619,.T.);
#8894=EDGE_CURVE('',#6832,#6827,#4620,.T.);
#8895=EDGE_CURVE('',#6833,#6834,#4621,.T.);
#8896=EDGE_CURVE('',#6835,#6833,#4622,.T.);
#8897=EDGE_CURVE('',#6836,#6835,#4623,.T.);
#8898=EDGE_CURVE('',#6837,#6836,#4624,.T.);
#8899=EDGE_CURVE('',#6838,#6837,#4625,.T.);
#8900=EDGE_CURVE('',#6834,#6838,#4626,.T.);
#8901=EDGE_CURVE('',#6839,#6839,#465,.T.);
#8902=EDGE_CURVE('',#6833,#6827,#4627,.T.);
#8903=EDGE_CURVE('',#6835,#6832,#4628,.T.);
#8904=EDGE_CURVE('',#6836,#6831,#4629,.T.);
#8905=EDGE_CURVE('',#6837,#6830,#4630,.T.);
#8906=EDGE_CURVE('',#6838,#6829,#4631,.T.);
#8907=EDGE_CURVE('',#6834,#6828,#4632,.T.);
#8908=EDGE_CURVE('',#6839,#6840,#4633,.T.);
#8909=EDGE_CURVE('',#6840,#6840,#466,.T.);
#8910=EDGE_CURVE('',#6840,#6841,#467,.T.);
#12189=ORIENTED_EDGE('',*,*,#8517,.F.);
#12190=ORIENTED_EDGE('',*,*,#8518,.T.);
#12191=ORIENTED_EDGE('',*,*,#8519,.T.);
#12192=ORIENTED_EDGE('',*,*,#8520,.T.);
#12193=ORIENTED_EDGE('',*,*,#8521,.F.);
#12194=ORIENTED_EDGE('',*,*,#8522,.T.);
#12195=ORIENTED_EDGE('',*,*,#8517,.T.);
#12196=ORIENTED_EDGE('',*,*,#8523,.T.);
#12197=ORIENTED_EDGE('',*,*,#8524,.F.);
#12198=ORIENTED_EDGE('',*,*,#8525,.T.);
#12199=ORIENTED_EDGE('',*,*,#8521,.T.);
#12200=ORIENTED_EDGE('',*,*,#8526,.T.);
#12201=ORIENTED_EDGE('',*,*,#8527,.F.);
#12202=ORIENTED_EDGE('',*,*,#8528,.T.);
#12203=ORIENTED_EDGE('',*,*,#8524,.T.);
#12204=ORIENTED_EDGE('',*,*,#8529,.T.);
#12205=ORIENTED_EDGE('',*,*,#8530,.F.);
#12206=ORIENTED_EDGE('',*,*,#8531,.T.);
#12207=ORIENTED_EDGE('',*,*,#8527,.T.);
#12208=ORIENTED_EDGE('',*,*,#8532,.T.);
#12209=ORIENTED_EDGE('',*,*,#8533,.F.);
#12210=ORIENTED_EDGE('',*,*,#8534,.T.);
#12211=ORIENTED_EDGE('',*,*,#8530,.T.);
#12212=ORIENTED_EDGE('',*,*,#8535,.T.);
#12213=ORIENTED_EDGE('',*,*,#8536,.F.);
#12214=ORIENTED_EDGE('',*,*,#8537,.T.);
#12215=ORIENTED_EDGE('',*,*,#8533,.T.);
#12216=ORIENTED_EDGE('',*,*,#8538,.T.);
#12217=ORIENTED_EDGE('',*,*,#8539,.F.);
#12218=ORIENTED_EDGE('',*,*,#8540,.T.);
#12219=ORIENTED_EDGE('',*,*,#8536,.T.);
#12220=ORIENTED_EDGE('',*,*,#8541,.T.);
#12221=ORIENTED_EDGE('',*,*,#8542,.F.);
#12222=ORIENTED_EDGE('',*,*,#8543,.T.);
#12223=ORIENTED_EDGE('',*,*,#8539,.T.);
#12224=ORIENTED_EDGE('',*,*,#8544,.T.);
#12225=ORIENTED_EDGE('',*,*,#8545,.F.);
#12226=ORIENTED_EDGE('',*,*,#8546,.T.);
#12227=ORIENTED_EDGE('',*,*,#8542,.T.);
#12228=ORIENTED_EDGE('',*,*,#8547,.T.);
#12229=ORIENTED_EDGE('',*,*,#8548,.F.);
#12230=ORIENTED_EDGE('',*,*,#8549,.T.);
#12231=ORIENTED_EDGE('',*,*,#8545,.T.);
#12232=ORIENTED_EDGE('',*,*,#8550,.T.);
#12233=ORIENTED_EDGE('',*,*,#8551,.F.);
#12234=ORIENTED_EDGE('',*,*,#8552,.T.);
#12235=ORIENTED_EDGE('',*,*,#8548,.T.);
#12236=ORIENTED_EDGE('',*,*,#8553,.T.);
#12237=ORIENTED_EDGE('',*,*,#8554,.F.);
#12238=ORIENTED_EDGE('',*,*,#8555,.T.);
#12239=ORIENTED_EDGE('',*,*,#8551,.T.);
#12240=ORIENTED_EDGE('',*,*,#8556,.T.);
#12241=ORIENTED_EDGE('',*,*,#8557,.F.);
#12242=ORIENTED_EDGE('',*,*,#8558,.T.);
#12243=ORIENTED_EDGE('',*,*,#8554,.T.);
#12244=ORIENTED_EDGE('',*,*,#8559,.T.);
#12245=ORIENTED_EDGE('',*,*,#8560,.F.);
#12246=ORIENTED_EDGE('',*,*,#8561,.T.);
#12247=ORIENTED_EDGE('',*,*,#8557,.T.);
#12248=ORIENTED_EDGE('',*,*,#8562,.T.);
#12249=ORIENTED_EDGE('',*,*,#8563,.F.);
#12250=ORIENTED_EDGE('',*,*,#8564,.T.);
#12251=ORIENTED_EDGE('',*,*,#8560,.T.);
#12252=ORIENTED_EDGE('',*,*,#8565,.T.);
#12253=ORIENTED_EDGE('',*,*,#8566,.F.);
#12254=ORIENTED_EDGE('',*,*,#8567,.T.);
#12255=ORIENTED_EDGE('',*,*,#8563,.T.);
#12256=ORIENTED_EDGE('',*,*,#8568,.T.);
#12257=ORIENTED_EDGE('',*,*,#8569,.F.);
#12258=ORIENTED_EDGE('',*,*,#8570,.T.);
#12259=ORIENTED_EDGE('',*,*,#8566,.T.);
#12260=ORIENTED_EDGE('',*,*,#8571,.T.);
#12261=ORIENTED_EDGE('',*,*,#8572,.F.);
#12262=ORIENTED_EDGE('',*,*,#8573,.T.);
#12263=ORIENTED_EDGE('',*,*,#8569,.T.);
#12264=ORIENTED_EDGE('',*,*,#8574,.T.);
#12265=ORIENTED_EDGE('',*,*,#8575,.F.);
#12266=ORIENTED_EDGE('',*,*,#8576,.T.);
#12267=ORIENTED_EDGE('',*,*,#8572,.T.);
#12268=ORIENTED_EDGE('',*,*,#8577,.T.);
#12269=ORIENTED_EDGE('',*,*,#8578,.F.);
#12270=ORIENTED_EDGE('',*,*,#8579,.T.);
#12271=ORIENTED_EDGE('',*,*,#8575,.T.);
#12272=ORIENTED_EDGE('',*,*,#8580,.T.);
#12273=ORIENTED_EDGE('',*,*,#8581,.F.);
#12274=ORIENTED_EDGE('',*,*,#8582,.T.);
#12275=ORIENTED_EDGE('',*,*,#8578,.T.);
#12276=ORIENTED_EDGE('',*,*,#8583,.T.);
#12277=ORIENTED_EDGE('',*,*,#8584,.F.);
#12278=ORIENTED_EDGE('',*,*,#8585,.T.);
#12279=ORIENTED_EDGE('',*,*,#8581,.T.);
#12280=ORIENTED_EDGE('',*,*,#8586,.T.);
#12281=ORIENTED_EDGE('',*,*,#8587,.F.);
#12282=ORIENTED_EDGE('',*,*,#8588,.T.);
#12283=ORIENTED_EDGE('',*,*,#8584,.T.);
#12284=ORIENTED_EDGE('',*,*,#8589,.T.);
#12285=ORIENTED_EDGE('',*,*,#8590,.F.);
#12286=ORIENTED_EDGE('',*,*,#8591,.T.);
#12287=ORIENTED_EDGE('',*,*,#8587,.T.);
#12288=ORIENTED_EDGE('',*,*,#8592,.T.);
#12289=ORIENTED_EDGE('',*,*,#8593,.F.);
#12290=ORIENTED_EDGE('',*,*,#8594,.T.);
#12291=ORIENTED_EDGE('',*,*,#8590,.T.);
#12292=ORIENTED_EDGE('',*,*,#8595,.T.);
#12293=ORIENTED_EDGE('',*,*,#8596,.F.);
#12294=ORIENTED_EDGE('',*,*,#8597,.T.);
#12295=ORIENTED_EDGE('',*,*,#8593,.T.);
#12296=ORIENTED_EDGE('',*,*,#8598,.T.);
#12297=ORIENTED_EDGE('',*,*,#8599,.F.);
#12298=ORIENTED_EDGE('',*,*,#8600,.T.);
#12299=ORIENTED_EDGE('',*,*,#8596,.T.);
#12300=ORIENTED_EDGE('',*,*,#8601,.T.);
#12301=ORIENTED_EDGE('',*,*,#8602,.F.);
#12302=ORIENTED_EDGE('',*,*,#8603,.T.);
#12303=ORIENTED_EDGE('',*,*,#8599,.T.);
#12304=ORIENTED_EDGE('',*,*,#8604,.T.);
#12305=ORIENTED_EDGE('',*,*,#8605,.F.);
#12306=ORIENTED_EDGE('',*,*,#8606,.T.);
#12307=ORIENTED_EDGE('',*,*,#8602,.T.);
#12308=ORIENTED_EDGE('',*,*,#8607,.T.);
#12309=ORIENTED_EDGE('',*,*,#8608,.F.);
#12310=ORIENTED_EDGE('',*,*,#8609,.T.);
#12311=ORIENTED_EDGE('',*,*,#8605,.T.);
#12312=ORIENTED_EDGE('',*,*,#8610,.T.);
#12313=ORIENTED_EDGE('',*,*,#8611,.F.);
#12314=ORIENTED_EDGE('',*,*,#8612,.T.);
#12315=ORIENTED_EDGE('',*,*,#8608,.T.);
#12316=ORIENTED_EDGE('',*,*,#8613,.T.);
#12317=ORIENTED_EDGE('',*,*,#8614,.F.);
#12318=ORIENTED_EDGE('',*,*,#8615,.T.);
#12319=ORIENTED_EDGE('',*,*,#8611,.T.);
#12320=ORIENTED_EDGE('',*,*,#8616,.T.);
#12321=ORIENTED_EDGE('',*,*,#8617,.F.);
#12322=ORIENTED_EDGE('',*,*,#8618,.T.);
#12323=ORIENTED_EDGE('',*,*,#8614,.T.);
#12324=ORIENTED_EDGE('',*,*,#8619,.T.);
#12325=ORIENTED_EDGE('',*,*,#8620,.F.);
#12326=ORIENTED_EDGE('',*,*,#8621,.T.);
#12327=ORIENTED_EDGE('',*,*,#8617,.T.);
#12328=ORIENTED_EDGE('',*,*,#8622,.T.);
#12329=ORIENTED_EDGE('',*,*,#8623,.F.);
#12330=ORIENTED_EDGE('',*,*,#8624,.T.);
#12331=ORIENTED_EDGE('',*,*,#8620,.T.);
#12332=ORIENTED_EDGE('',*,*,#8625,.T.);
#12333=ORIENTED_EDGE('',*,*,#8626,.F.);
#12334=ORIENTED_EDGE('',*,*,#8627,.T.);
#12335=ORIENTED_EDGE('',*,*,#8623,.T.);
#12336=ORIENTED_EDGE('',*,*,#8628,.T.);
#12337=ORIENTED_EDGE('',*,*,#8629,.F.);
#12338=ORIENTED_EDGE('',*,*,#8630,.T.);
#12339=ORIENTED_EDGE('',*,*,#8626,.T.);
#12340=ORIENTED_EDGE('',*,*,#8631,.T.);
#12341=ORIENTED_EDGE('',*,*,#8632,.F.);
#12342=ORIENTED_EDGE('',*,*,#8633,.T.);
#12343=ORIENTED_EDGE('',*,*,#8629,.T.);
#12344=ORIENTED_EDGE('',*,*,#8634,.T.);
#12345=ORIENTED_EDGE('',*,*,#8635,.F.);
#12346=ORIENTED_EDGE('',*,*,#8636,.T.);
#12347=ORIENTED_EDGE('',*,*,#8632,.T.);
#12348=ORIENTED_EDGE('',*,*,#8637,.T.);
#12349=ORIENTED_EDGE('',*,*,#8638,.F.);
#12350=ORIENTED_EDGE('',*,*,#8639,.T.);
#12351=ORIENTED_EDGE('',*,*,#8635,.T.);
#12352=ORIENTED_EDGE('',*,*,#8640,.T.);
#12353=ORIENTED_EDGE('',*,*,#8641,.F.);
#12354=ORIENTED_EDGE('',*,*,#8642,.T.);
#12355=ORIENTED_EDGE('',*,*,#8638,.T.);
#12356=ORIENTED_EDGE('',*,*,#8643,.T.);
#12357=ORIENTED_EDGE('',*,*,#8644,.F.);
#12358=ORIENTED_EDGE('',*,*,#8645,.T.);
#12359=ORIENTED_EDGE('',*,*,#8641,.T.);
#12360=ORIENTED_EDGE('',*,*,#8646,.T.);
#12361=ORIENTED_EDGE('',*,*,#8647,.F.);
#12362=ORIENTED_EDGE('',*,*,#8648,.T.);
#12363=ORIENTED_EDGE('',*,*,#8644,.T.);
#12364=ORIENTED_EDGE('',*,*,#8649,.T.);
#12365=ORIENTED_EDGE('',*,*,#8650,.F.);
#12366=ORIENTED_EDGE('',*,*,#8651,.T.);
#12367=ORIENTED_EDGE('',*,*,#8647,.T.);
#12368=ORIENTED_EDGE('',*,*,#8652,.T.);
#12369=ORIENTED_EDGE('',*,*,#8653,.F.);
#12370=ORIENTED_EDGE('',*,*,#8654,.T.);
#12371=ORIENTED_EDGE('',*,*,#8650,.T.);
#12372=ORIENTED_EDGE('',*,*,#8655,.T.);
#12373=ORIENTED_EDGE('',*,*,#8656,.F.);
#12374=ORIENTED_EDGE('',*,*,#8657,.T.);
#12375=ORIENTED_EDGE('',*,*,#8653,.T.);
#12376=ORIENTED_EDGE('',*,*,#8658,.T.);
#12377=ORIENTED_EDGE('',*,*,#8659,.F.);
#12378=ORIENTED_EDGE('',*,*,#8660,.T.);
#12379=ORIENTED_EDGE('',*,*,#8656,.T.);
#12380=ORIENTED_EDGE('',*,*,#8661,.T.);
#12381=ORIENTED_EDGE('',*,*,#8662,.F.);
#12382=ORIENTED_EDGE('',*,*,#8663,.T.);
#12383=ORIENTED_EDGE('',*,*,#8659,.T.);
#12384=ORIENTED_EDGE('',*,*,#8664,.T.);
#12385=ORIENTED_EDGE('',*,*,#8665,.F.);
#12386=ORIENTED_EDGE('',*,*,#8666,.T.);
#12387=ORIENTED_EDGE('',*,*,#8662,.T.);
#12388=ORIENTED_EDGE('',*,*,#8667,.T.);
#12389=ORIENTED_EDGE('',*,*,#8668,.F.);
#12390=ORIENTED_EDGE('',*,*,#8669,.T.);
#12391=ORIENTED_EDGE('',*,*,#8665,.T.);
#12392=ORIENTED_EDGE('',*,*,#8670,.T.);
#12393=ORIENTED_EDGE('',*,*,#8671,.F.);
#12394=ORIENTED_EDGE('',*,*,#8672,.T.);
#12395=ORIENTED_EDGE('',*,*,#8668,.T.);
#12396=ORIENTED_EDGE('',*,*,#8673,.T.);
#12397=ORIENTED_EDGE('',*,*,#8674,.F.);
#12398=ORIENTED_EDGE('',*,*,#8675,.T.);
#12399=ORIENTED_EDGE('',*,*,#8671,.T.);
#12400=ORIENTED_EDGE('',*,*,#8676,.T.);
#12401=ORIENTED_EDGE('',*,*,#8677,.F.);
#12402=ORIENTED_EDGE('',*,*,#8678,.T.);
#12403=ORIENTED_EDGE('',*,*,#8674,.T.);
#12404=ORIENTED_EDGE('',*,*,#8679,.T.);
#12405=ORIENTED_EDGE('',*,*,#8680,.F.);
#12406=ORIENTED_EDGE('',*,*,#8681,.T.);
#12407=ORIENTED_EDGE('',*,*,#8677,.T.);
#12408=ORIENTED_EDGE('',*,*,#8682,.T.);
#12409=ORIENTED_EDGE('',*,*,#8683,.F.);
#12410=ORIENTED_EDGE('',*,*,#8684,.T.);
#12411=ORIENTED_EDGE('',*,*,#8680,.T.);
#12412=ORIENTED_EDGE('',*,*,#8685,.T.);
#12413=ORIENTED_EDGE('',*,*,#8686,.F.);
#12414=ORIENTED_EDGE('',*,*,#8687,.T.);
#12415=ORIENTED_EDGE('',*,*,#8683,.T.);
#12416=ORIENTED_EDGE('',*,*,#8688,.T.);
#12417=ORIENTED_EDGE('',*,*,#8689,.F.);
#12418=ORIENTED_EDGE('',*,*,#8690,.T.);
#12419=ORIENTED_EDGE('',*,*,#8686,.T.);
#12420=ORIENTED_EDGE('',*,*,#8691,.T.);
#12421=ORIENTED_EDGE('',*,*,#8692,.F.);
#12422=ORIENTED_EDGE('',*,*,#8693,.T.);
#12423=ORIENTED_EDGE('',*,*,#8689,.T.);
#12424=ORIENTED_EDGE('',*,*,#8694,.T.);
#12425=ORIENTED_EDGE('',*,*,#8695,.F.);
#12426=ORIENTED_EDGE('',*,*,#8696,.T.);
#12427=ORIENTED_EDGE('',*,*,#8692,.T.);
#12428=ORIENTED_EDGE('',*,*,#8697,.T.);
#12429=ORIENTED_EDGE('',*,*,#8698,.F.);
#12430=ORIENTED_EDGE('',*,*,#8699,.T.);
#12431=ORIENTED_EDGE('',*,*,#8700,.F.);
#12432=ORIENTED_EDGE('',*,*,#8701,.F.);
#12433=ORIENTED_EDGE('',*,*,#8702,.F.);
#12434=ORIENTED_EDGE('',*,*,#8703,.T.);
#12435=ORIENTED_EDGE('',*,*,#8698,.T.);
#12436=ORIENTED_EDGE('',*,*,#8704,.F.);
#12437=ORIENTED_EDGE('',*,*,#8705,.F.);
#12438=ORIENTED_EDGE('',*,*,#8706,.T.);
#12439=ORIENTED_EDGE('',*,*,#8702,.T.);
#12440=ORIENTED_EDGE('',*,*,#8707,.F.);
#12441=ORIENTED_EDGE('',*,*,#8708,.F.);
#12442=ORIENTED_EDGE('',*,*,#8709,.T.);
#12443=ORIENTED_EDGE('',*,*,#8705,.T.);
#12444=ORIENTED_EDGE('',*,*,#8710,.F.);
#12445=ORIENTED_EDGE('',*,*,#8711,.F.);
#12446=ORIENTED_EDGE('',*,*,#8712,.T.);
#12447=ORIENTED_EDGE('',*,*,#8708,.T.);
#12448=ORIENTED_EDGE('',*,*,#8713,.F.);
#12449=ORIENTED_EDGE('',*,*,#8714,.F.);
#12450=ORIENTED_EDGE('',*,*,#8715,.T.);
#12451=ORIENTED_EDGE('',*,*,#8711,.T.);
#12452=ORIENTED_EDGE('',*,*,#8716,.F.);
#12453=ORIENTED_EDGE('',*,*,#8717,.F.);
#12454=ORIENTED_EDGE('',*,*,#8718,.T.);
#12455=ORIENTED_EDGE('',*,*,#8714,.T.);
#12456=ORIENTED_EDGE('',*,*,#8719,.F.);
#12457=ORIENTED_EDGE('',*,*,#8720,.F.);
#12458=ORIENTED_EDGE('',*,*,#8721,.T.);
#12459=ORIENTED_EDGE('',*,*,#8717,.T.);
#12460=ORIENTED_EDGE('',*,*,#8722,.F.);
#12461=ORIENTED_EDGE('',*,*,#8723,.F.);
#12462=ORIENTED_EDGE('',*,*,#8724,.T.);
#12463=ORIENTED_EDGE('',*,*,#8720,.T.);
#12464=ORIENTED_EDGE('',*,*,#8725,.F.);
#12465=ORIENTED_EDGE('',*,*,#8726,.F.);
#12466=ORIENTED_EDGE('',*,*,#8727,.T.);
#12467=ORIENTED_EDGE('',*,*,#8723,.T.);
#12468=ORIENTED_EDGE('',*,*,#8728,.F.);
#12469=ORIENTED_EDGE('',*,*,#8729,.F.);
#12470=ORIENTED_EDGE('',*,*,#8730,.T.);
#12471=ORIENTED_EDGE('',*,*,#8726,.T.);
#12472=ORIENTED_EDGE('',*,*,#8731,.F.);
#12473=ORIENTED_EDGE('',*,*,#8732,.F.);
#12474=ORIENTED_EDGE('',*,*,#8733,.T.);
#12475=ORIENTED_EDGE('',*,*,#8729,.T.);
#12476=ORIENTED_EDGE('',*,*,#8734,.F.);
#12477=ORIENTED_EDGE('',*,*,#8735,.F.);
#12478=ORIENTED_EDGE('',*,*,#8736,.T.);
#12479=ORIENTED_EDGE('',*,*,#8732,.T.);
#12480=ORIENTED_EDGE('',*,*,#8737,.F.);
#12481=ORIENTED_EDGE('',*,*,#8738,.F.);
#12482=ORIENTED_EDGE('',*,*,#8739,.T.);
#12483=ORIENTED_EDGE('',*,*,#8735,.T.);
#12484=ORIENTED_EDGE('',*,*,#8740,.F.);
#12485=ORIENTED_EDGE('',*,*,#8741,.F.);
#12486=ORIENTED_EDGE('',*,*,#8742,.T.);
#12487=ORIENTED_EDGE('',*,*,#8738,.T.);
#12488=ORIENTED_EDGE('',*,*,#8743,.F.);
#12489=ORIENTED_EDGE('',*,*,#8744,.F.);
#12490=ORIENTED_EDGE('',*,*,#8745,.T.);
#12491=ORIENTED_EDGE('',*,*,#8741,.T.);
#12492=ORIENTED_EDGE('',*,*,#8746,.F.);
#12493=ORIENTED_EDGE('',*,*,#8747,.F.);
#12494=ORIENTED_EDGE('',*,*,#8748,.T.);
#12495=ORIENTED_EDGE('',*,*,#8744,.T.);
#12496=ORIENTED_EDGE('',*,*,#8749,.F.);
#12497=ORIENTED_EDGE('',*,*,#8750,.F.);
#12498=ORIENTED_EDGE('',*,*,#8751,.T.);
#12499=ORIENTED_EDGE('',*,*,#8747,.T.);
#12500=ORIENTED_EDGE('',*,*,#8752,.F.);
#12501=ORIENTED_EDGE('',*,*,#8753,.F.);
#12502=ORIENTED_EDGE('',*,*,#8754,.T.);
#12503=ORIENTED_EDGE('',*,*,#8750,.T.);
#12504=ORIENTED_EDGE('',*,*,#8755,.F.);
#12505=ORIENTED_EDGE('',*,*,#8756,.F.);
#12506=ORIENTED_EDGE('',*,*,#8757,.T.);
#12507=ORIENTED_EDGE('',*,*,#8753,.T.);
#12508=ORIENTED_EDGE('',*,*,#8758,.F.);
#12509=ORIENTED_EDGE('',*,*,#8759,.F.);
#12510=ORIENTED_EDGE('',*,*,#8760,.T.);
#12511=ORIENTED_EDGE('',*,*,#8756,.T.);
#12512=ORIENTED_EDGE('',*,*,#8761,.F.);
#12513=ORIENTED_EDGE('',*,*,#8762,.F.);
#12514=ORIENTED_EDGE('',*,*,#8763,.T.);
#12515=ORIENTED_EDGE('',*,*,#8759,.T.);
#12516=ORIENTED_EDGE('',*,*,#8764,.F.);
#12517=ORIENTED_EDGE('',*,*,#8765,.F.);
#12518=ORIENTED_EDGE('',*,*,#8766,.T.);
#12519=ORIENTED_EDGE('',*,*,#8762,.T.);
#12520=ORIENTED_EDGE('',*,*,#8767,.F.);
#12521=ORIENTED_EDGE('',*,*,#8768,.F.);
#12522=ORIENTED_EDGE('',*,*,#8769,.T.);
#12523=ORIENTED_EDGE('',*,*,#8765,.T.);
#12524=ORIENTED_EDGE('',*,*,#8770,.F.);
#12525=ORIENTED_EDGE('',*,*,#8771,.F.);
#12526=ORIENTED_EDGE('',*,*,#8772,.T.);
#12527=ORIENTED_EDGE('',*,*,#8768,.T.);
#12528=ORIENTED_EDGE('',*,*,#8773,.F.);
#12529=ORIENTED_EDGE('',*,*,#8774,.F.);
#12530=ORIENTED_EDGE('',*,*,#8775,.T.);
#12531=ORIENTED_EDGE('',*,*,#8771,.T.);
#12532=ORIENTED_EDGE('',*,*,#8776,.F.);
#12533=ORIENTED_EDGE('',*,*,#8777,.F.);
#12534=ORIENTED_EDGE('',*,*,#8778,.T.);
#12535=ORIENTED_EDGE('',*,*,#8774,.T.);
#12536=ORIENTED_EDGE('',*,*,#8779,.F.);
#12537=ORIENTED_EDGE('',*,*,#8780,.F.);
#12538=ORIENTED_EDGE('',*,*,#8781,.T.);
#12539=ORIENTED_EDGE('',*,*,#8777,.T.);
#12540=ORIENTED_EDGE('',*,*,#8782,.F.);
#12541=ORIENTED_EDGE('',*,*,#8783,.F.);
#12542=ORIENTED_EDGE('',*,*,#8784,.T.);
#12543=ORIENTED_EDGE('',*,*,#8780,.T.);
#12544=ORIENTED_EDGE('',*,*,#8785,.F.);
#12545=ORIENTED_EDGE('',*,*,#8786,.F.);
#12546=ORIENTED_EDGE('',*,*,#8787,.T.);
#12547=ORIENTED_EDGE('',*,*,#8783,.T.);
#12548=ORIENTED_EDGE('',*,*,#8788,.F.);
#12549=ORIENTED_EDGE('',*,*,#8789,.F.);
#12550=ORIENTED_EDGE('',*,*,#8790,.T.);
#12551=ORIENTED_EDGE('',*,*,#8786,.T.);
#12552=ORIENTED_EDGE('',*,*,#8791,.F.);
#12553=ORIENTED_EDGE('',*,*,#8792,.F.);
#12554=ORIENTED_EDGE('',*,*,#8793,.T.);
#12555=ORIENTED_EDGE('',*,*,#8789,.T.);
#12556=ORIENTED_EDGE('',*,*,#8794,.F.);
#12557=ORIENTED_EDGE('',*,*,#8795,.F.);
#12558=ORIENTED_EDGE('',*,*,#8796,.T.);
#12559=ORIENTED_EDGE('',*,*,#8792,.T.);
#12560=ORIENTED_EDGE('',*,*,#8797,.F.);
#12561=ORIENTED_EDGE('',*,*,#8798,.F.);
#12562=ORIENTED_EDGE('',*,*,#8799,.T.);
#12563=ORIENTED_EDGE('',*,*,#8795,.T.);
#12564=ORIENTED_EDGE('',*,*,#8800,.F.);
#12565=ORIENTED_EDGE('',*,*,#8801,.F.);
#12566=ORIENTED_EDGE('',*,*,#8802,.T.);
#12567=ORIENTED_EDGE('',*,*,#8798,.T.);
#12568=ORIENTED_EDGE('',*,*,#8803,.F.);
#12569=ORIENTED_EDGE('',*,*,#8804,.F.);
#12570=ORIENTED_EDGE('',*,*,#8805,.T.);
#12571=ORIENTED_EDGE('',*,*,#8801,.T.);
#12572=ORIENTED_EDGE('',*,*,#8806,.F.);
#12573=ORIENTED_EDGE('',*,*,#8807,.F.);
#12574=ORIENTED_EDGE('',*,*,#8808,.T.);
#12575=ORIENTED_EDGE('',*,*,#8804,.T.);
#12576=ORIENTED_EDGE('',*,*,#8809,.F.);
#12577=ORIENTED_EDGE('',*,*,#8810,.F.);
#12578=ORIENTED_EDGE('',*,*,#8811,.T.);
#12579=ORIENTED_EDGE('',*,*,#8807,.T.);
#12580=ORIENTED_EDGE('',*,*,#8812,.F.);
#12581=ORIENTED_EDGE('',*,*,#8813,.F.);
#12582=ORIENTED_EDGE('',*,*,#8814,.T.);
#12583=ORIENTED_EDGE('',*,*,#8810,.T.);
#12584=ORIENTED_EDGE('',*,*,#8815,.F.);
#12585=ORIENTED_EDGE('',*,*,#8816,.F.);
#12586=ORIENTED_EDGE('',*,*,#8817,.T.);
#12587=ORIENTED_EDGE('',*,*,#8813,.T.);
#12588=ORIENTED_EDGE('',*,*,#8818,.F.);
#12589=ORIENTED_EDGE('',*,*,#8819,.F.);
#12590=ORIENTED_EDGE('',*,*,#8820,.T.);
#12591=ORIENTED_EDGE('',*,*,#8816,.T.);
#12592=ORIENTED_EDGE('',*,*,#8821,.F.);
#12593=ORIENTED_EDGE('',*,*,#8822,.F.);
#12594=ORIENTED_EDGE('',*,*,#8823,.T.);
#12595=ORIENTED_EDGE('',*,*,#8819,.T.);
#12596=ORIENTED_EDGE('',*,*,#8824,.F.);
#12597=ORIENTED_EDGE('',*,*,#8825,.F.);
#12598=ORIENTED_EDGE('',*,*,#8826,.T.);
#12599=ORIENTED_EDGE('',*,*,#8822,.T.);
#12600=ORIENTED_EDGE('',*,*,#8827,.F.);
#12601=ORIENTED_EDGE('',*,*,#8828,.F.);
#12602=ORIENTED_EDGE('',*,*,#8829,.T.);
#12603=ORIENTED_EDGE('',*,*,#8825,.T.);
#12604=ORIENTED_EDGE('',*,*,#8830,.F.);
#12605=ORIENTED_EDGE('',*,*,#8831,.F.);
#12606=ORIENTED_EDGE('',*,*,#8832,.T.);
#12607=ORIENTED_EDGE('',*,*,#8828,.T.);
#12608=ORIENTED_EDGE('',*,*,#8833,.F.);
#12609=ORIENTED_EDGE('',*,*,#8834,.F.);
#12610=ORIENTED_EDGE('',*,*,#8835,.T.);
#12611=ORIENTED_EDGE('',*,*,#8831,.T.);
#12612=ORIENTED_EDGE('',*,*,#8836,.F.);
#12613=ORIENTED_EDGE('',*,*,#8837,.F.);
#12614=ORIENTED_EDGE('',*,*,#8838,.T.);
#12615=ORIENTED_EDGE('',*,*,#8834,.T.);
#12616=ORIENTED_EDGE('',*,*,#8839,.F.);
#12617=ORIENTED_EDGE('',*,*,#8840,.F.);
#12618=ORIENTED_EDGE('',*,*,#8841,.T.);
#12619=ORIENTED_EDGE('',*,*,#8837,.T.);
#12620=ORIENTED_EDGE('',*,*,#8842,.F.);
#12621=ORIENTED_EDGE('',*,*,#8843,.F.);
#12622=ORIENTED_EDGE('',*,*,#8844,.T.);
#12623=ORIENTED_EDGE('',*,*,#8840,.T.);
#12624=ORIENTED_EDGE('',*,*,#8845,.F.);
#12625=ORIENTED_EDGE('',*,*,#8846,.F.);
#12626=ORIENTED_EDGE('',*,*,#8847,.T.);
#12627=ORIENTED_EDGE('',*,*,#8843,.T.);
#12628=ORIENTED_EDGE('',*,*,#8848,.F.);
#12629=ORIENTED_EDGE('',*,*,#8849,.F.);
#12630=ORIENTED_EDGE('',*,*,#8850,.T.);
#12631=ORIENTED_EDGE('',*,*,#8846,.T.);
#12632=ORIENTED_EDGE('',*,*,#8851,.F.);
#12633=ORIENTED_EDGE('',*,*,#8852,.F.);
#12634=ORIENTED_EDGE('',*,*,#8853,.T.);
#12635=ORIENTED_EDGE('',*,*,#8849,.T.);
#12636=ORIENTED_EDGE('',*,*,#8854,.F.);
#12637=ORIENTED_EDGE('',*,*,#8855,.F.);
#12638=ORIENTED_EDGE('',*,*,#8856,.T.);
#12639=ORIENTED_EDGE('',*,*,#8852,.T.);
#12640=ORIENTED_EDGE('',*,*,#8857,.F.);
#12641=ORIENTED_EDGE('',*,*,#8858,.F.);
#12642=ORIENTED_EDGE('',*,*,#8859,.T.);
#12643=ORIENTED_EDGE('',*,*,#8855,.T.);
#12644=ORIENTED_EDGE('',*,*,#8860,.F.);
#12645=ORIENTED_EDGE('',*,*,#8861,.F.);
#12646=ORIENTED_EDGE('',*,*,#8862,.T.);
#12647=ORIENTED_EDGE('',*,*,#8858,.T.);
#12648=ORIENTED_EDGE('',*,*,#8863,.F.);
#12649=ORIENTED_EDGE('',*,*,#8864,.F.);
#12650=ORIENTED_EDGE('',*,*,#8865,.T.);
#12651=ORIENTED_EDGE('',*,*,#8861,.T.);
#12652=ORIENTED_EDGE('',*,*,#8866,.F.);
#12653=ORIENTED_EDGE('',*,*,#8867,.F.);
#12654=ORIENTED_EDGE('',*,*,#8868,.T.);
#12655=ORIENTED_EDGE('',*,*,#8864,.T.);
#12656=ORIENTED_EDGE('',*,*,#8869,.F.);
#12657=ORIENTED_EDGE('',*,*,#8870,.F.);
#12658=ORIENTED_EDGE('',*,*,#8871,.T.);
#12659=ORIENTED_EDGE('',*,*,#8867,.T.);
#12660=ORIENTED_EDGE('',*,*,#8872,.F.);
#12661=ORIENTED_EDGE('',*,*,#8873,.F.);
#12662=ORIENTED_EDGE('',*,*,#8874,.T.);
#12663=ORIENTED_EDGE('',*,*,#8870,.T.);
#12664=ORIENTED_EDGE('',*,*,#8875,.F.);
#12665=ORIENTED_EDGE('',*,*,#8876,.F.);
#12666=ORIENTED_EDGE('',*,*,#8877,.T.);
#12667=ORIENTED_EDGE('',*,*,#8873,.T.);
#12668=ORIENTED_EDGE('',*,*,#8878,.F.);
#12669=ORIENTED_EDGE('',*,*,#8879,.F.);
#12670=ORIENTED_EDGE('',*,*,#8880,.F.);
#12671=ORIENTED_EDGE('',*,*,#8697,.F.);
#12672=ORIENTED_EDGE('',*,*,#8694,.F.);
#12673=ORIENTED_EDGE('',*,*,#8691,.F.);
#12674=ORIENTED_EDGE('',*,*,#8688,.F.);
#12675=ORIENTED_EDGE('',*,*,#8685,.F.);
#12676=ORIENTED_EDGE('',*,*,#8682,.F.);
#12677=ORIENTED_EDGE('',*,*,#8679,.F.);
#12678=ORIENTED_EDGE('',*,*,#8676,.F.);
#12679=ORIENTED_EDGE('',*,*,#8673,.F.);
#12680=ORIENTED_EDGE('',*,*,#8670,.F.);
#12681=ORIENTED_EDGE('',*,*,#8667,.F.);
#12682=ORIENTED_EDGE('',*,*,#8664,.F.);
#12683=ORIENTED_EDGE('',*,*,#8661,.F.);
#12684=ORIENTED_EDGE('',*,*,#8658,.F.);
#12685=ORIENTED_EDGE('',*,*,#8655,.F.);
#12686=ORIENTED_EDGE('',*,*,#8652,.F.);
#12687=ORIENTED_EDGE('',*,*,#8649,.F.);
#12688=ORIENTED_EDGE('',*,*,#8646,.F.);
#12689=ORIENTED_EDGE('',*,*,#8643,.F.);
#12690=ORIENTED_EDGE('',*,*,#8640,.F.);
#12691=ORIENTED_EDGE('',*,*,#8637,.F.);
#12692=ORIENTED_EDGE('',*,*,#8634,.F.);
#12693=ORIENTED_EDGE('',*,*,#8631,.F.);
#12694=ORIENTED_EDGE('',*,*,#8628,.F.);
#12695=ORIENTED_EDGE('',*,*,#8625,.F.);
#12696=ORIENTED_EDGE('',*,*,#8622,.F.);
#12697=ORIENTED_EDGE('',*,*,#8619,.F.);
#12698=ORIENTED_EDGE('',*,*,#8616,.F.);
#12699=ORIENTED_EDGE('',*,*,#8613,.F.);
#12700=ORIENTED_EDGE('',*,*,#8610,.F.);
#12701=ORIENTED_EDGE('',*,*,#8607,.F.);
#12702=ORIENTED_EDGE('',*,*,#8604,.F.);
#12703=ORIENTED_EDGE('',*,*,#8601,.F.);
#12704=ORIENTED_EDGE('',*,*,#8598,.F.);
#12705=ORIENTED_EDGE('',*,*,#8595,.F.);
#12706=ORIENTED_EDGE('',*,*,#8592,.F.);
#12707=ORIENTED_EDGE('',*,*,#8589,.F.);
#12708=ORIENTED_EDGE('',*,*,#8586,.F.);
#12709=ORIENTED_EDGE('',*,*,#8583,.F.);
#12710=ORIENTED_EDGE('',*,*,#8580,.F.);
#12711=ORIENTED_EDGE('',*,*,#8577,.F.);
#12712=ORIENTED_EDGE('',*,*,#8574,.F.);
#12713=ORIENTED_EDGE('',*,*,#8571,.F.);
#12714=ORIENTED_EDGE('',*,*,#8568,.F.);
#12715=ORIENTED_EDGE('',*,*,#8565,.F.);
#12716=ORIENTED_EDGE('',*,*,#8562,.F.);
#12717=ORIENTED_EDGE('',*,*,#8559,.F.);
#12718=ORIENTED_EDGE('',*,*,#8556,.F.);
#12719=ORIENTED_EDGE('',*,*,#8553,.F.);
#12720=ORIENTED_EDGE('',*,*,#8550,.F.);
#12721=ORIENTED_EDGE('',*,*,#8547,.F.);
#12722=ORIENTED_EDGE('',*,*,#8544,.F.);
#12723=ORIENTED_EDGE('',*,*,#8541,.F.);
#12724=ORIENTED_EDGE('',*,*,#8538,.F.);
#12725=ORIENTED_EDGE('',*,*,#8535,.F.);
#12726=ORIENTED_EDGE('',*,*,#8532,.F.);
#12727=ORIENTED_EDGE('',*,*,#8529,.F.);
#12728=ORIENTED_EDGE('',*,*,#8526,.F.);
#12729=ORIENTED_EDGE('',*,*,#8523,.F.);
#12730=ORIENTED_EDGE('',*,*,#8520,.F.);
#12731=ORIENTED_EDGE('',*,*,#8881,.F.);
#12732=ORIENTED_EDGE('',*,*,#8882,.T.);
#12733=ORIENTED_EDGE('',*,*,#8878,.T.);
#12734=ORIENTED_EDGE('',*,*,#8875,.T.);
#12735=ORIENTED_EDGE('',*,*,#8872,.T.);
#12736=ORIENTED_EDGE('',*,*,#8869,.T.);
#12737=ORIENTED_EDGE('',*,*,#8866,.T.);
#12738=ORIENTED_EDGE('',*,*,#8863,.T.);
#12739=ORIENTED_EDGE('',*,*,#8860,.T.);
#12740=ORIENTED_EDGE('',*,*,#8857,.T.);
#12741=ORIENTED_EDGE('',*,*,#8854,.T.);
#12742=ORIENTED_EDGE('',*,*,#8851,.T.);
#12743=ORIENTED_EDGE('',*,*,#8848,.T.);
#12744=ORIENTED_EDGE('',*,*,#8845,.T.);
#12745=ORIENTED_EDGE('',*,*,#8842,.T.);
#12746=ORIENTED_EDGE('',*,*,#8839,.T.);
#12747=ORIENTED_EDGE('',*,*,#8836,.T.);
#12748=ORIENTED_EDGE('',*,*,#8833,.T.);
#12749=ORIENTED_EDGE('',*,*,#8830,.T.);
#12750=ORIENTED_EDGE('',*,*,#8827,.T.);
#12751=ORIENTED_EDGE('',*,*,#8824,.T.);
#12752=ORIENTED_EDGE('',*,*,#8821,.T.);
#12753=ORIENTED_EDGE('',*,*,#8818,.T.);
#12754=ORIENTED_EDGE('',*,*,#8815,.T.);
#12755=ORIENTED_EDGE('',*,*,#8812,.T.);
#12756=ORIENTED_EDGE('',*,*,#8809,.T.);
#12757=ORIENTED_EDGE('',*,*,#8806,.T.);
#12758=ORIENTED_EDGE('',*,*,#8803,.T.);
#12759=ORIENTED_EDGE('',*,*,#8800,.T.);
#12760=ORIENTED_EDGE('',*,*,#8797,.T.);
#12761=ORIENTED_EDGE('',*,*,#8794,.T.);
#12762=ORIENTED_EDGE('',*,*,#8791,.T.);
#12763=ORIENTED_EDGE('',*,*,#8788,.T.);
#12764=ORIENTED_EDGE('',*,*,#8785,.T.);
#12765=ORIENTED_EDGE('',*,*,#8782,.T.);
#12766=ORIENTED_EDGE('',*,*,#8779,.T.);
#12767=ORIENTED_EDGE('',*,*,#8776,.T.);
#12768=ORIENTED_EDGE('',*,*,#8773,.T.);
#12769=ORIENTED_EDGE('',*,*,#8770,.T.);
#12770=ORIENTED_EDGE('',*,*,#8767,.T.);
#12771=ORIENTED_EDGE('',*,*,#8764,.T.);
#12772=ORIENTED_EDGE('',*,*,#8761,.T.);
#12773=ORIENTED_EDGE('',*,*,#8758,.T.);
#12774=ORIENTED_EDGE('',*,*,#8755,.T.);
#12775=ORIENTED_EDGE('',*,*,#8752,.T.);
#12776=ORIENTED_EDGE('',*,*,#8749,.T.);
#12777=ORIENTED_EDGE('',*,*,#8746,.T.);
#12778=ORIENTED_EDGE('',*,*,#8743,.T.);
#12779=ORIENTED_EDGE('',*,*,#8740,.T.);
#12780=ORIENTED_EDGE('',*,*,#8737,.T.);
#12781=ORIENTED_EDGE('',*,*,#8734,.T.);
#12782=ORIENTED_EDGE('',*,*,#8731,.T.);
#12783=ORIENTED_EDGE('',*,*,#8728,.T.);
#12784=ORIENTED_EDGE('',*,*,#8725,.T.);
#12785=ORIENTED_EDGE('',*,*,#8722,.T.);
#12786=ORIENTED_EDGE('',*,*,#8719,.T.);
#12787=ORIENTED_EDGE('',*,*,#8716,.T.);
#12788=ORIENTED_EDGE('',*,*,#8713,.T.);
#12789=ORIENTED_EDGE('',*,*,#8710,.T.);
#12790=ORIENTED_EDGE('',*,*,#8707,.T.);
#12791=ORIENTED_EDGE('',*,*,#8704,.T.);
#12792=ORIENTED_EDGE('',*,*,#8701,.T.);
#12793=ORIENTED_EDGE('',*,*,#8876,.T.);
#12794=ORIENTED_EDGE('',*,*,#8882,.F.);
#12795=ORIENTED_EDGE('',*,*,#8883,.F.);
#12796=ORIENTED_EDGE('',*,*,#8884,.T.);
#12797=ORIENTED_EDGE('',*,*,#8885,.F.);
#12798=ORIENTED_EDGE('',*,*,#8699,.F.);
#12799=ORIENTED_EDGE('',*,*,#8703,.F.);
#12800=ORIENTED_EDGE('',*,*,#8706,.F.);
#12801=ORIENTED_EDGE('',*,*,#8709,.F.);
#12802=ORIENTED_EDGE('',*,*,#8712,.F.);
#12803=ORIENTED_EDGE('',*,*,#8715,.F.);
#12804=ORIENTED_EDGE('',*,*,#8718,.F.);
#12805=ORIENTED_EDGE('',*,*,#8721,.F.);
#12806=ORIENTED_EDGE('',*,*,#8724,.F.);
#12807=ORIENTED_EDGE('',*,*,#8727,.F.);
#12808=ORIENTED_EDGE('',*,*,#8730,.F.);
#12809=ORIENTED_EDGE('',*,*,#8733,.F.);
#12810=ORIENTED_EDGE('',*,*,#8736,.F.);
#12811=ORIENTED_EDGE('',*,*,#8739,.F.);
#12812=ORIENTED_EDGE('',*,*,#8742,.F.);
#12813=ORIENTED_EDGE('',*,*,#8745,.F.);
#12814=ORIENTED_EDGE('',*,*,#8748,.F.);
#12815=ORIENTED_EDGE('',*,*,#8751,.F.);
#12816=ORIENTED_EDGE('',*,*,#8754,.F.);
#12817=ORIENTED_EDGE('',*,*,#8757,.F.);
#12818=ORIENTED_EDGE('',*,*,#8760,.F.);
#12819=ORIENTED_EDGE('',*,*,#8763,.F.);
#12820=ORIENTED_EDGE('',*,*,#8766,.F.);
#12821=ORIENTED_EDGE('',*,*,#8769,.F.);
#12822=ORIENTED_EDGE('',*,*,#8772,.F.);
#12823=ORIENTED_EDGE('',*,*,#8775,.F.);
#12824=ORIENTED_EDGE('',*,*,#8778,.F.);
#12825=ORIENTED_EDGE('',*,*,#8781,.F.);
#12826=ORIENTED_EDGE('',*,*,#8784,.F.);
#12827=ORIENTED_EDGE('',*,*,#8787,.F.);
#12828=ORIENTED_EDGE('',*,*,#8790,.F.);
#12829=ORIENTED_EDGE('',*,*,#8793,.F.);
#12830=ORIENTED_EDGE('',*,*,#8796,.F.);
#12831=ORIENTED_EDGE('',*,*,#8799,.F.);
#12832=ORIENTED_EDGE('',*,*,#8802,.F.);
#12833=ORIENTED_EDGE('',*,*,#8805,.F.);
#12834=ORIENTED_EDGE('',*,*,#8808,.F.);
#12835=ORIENTED_EDGE('',*,*,#8811,.F.);
#12836=ORIENTED_EDGE('',*,*,#8814,.F.);
#12837=ORIENTED_EDGE('',*,*,#8817,.F.);
#12838=ORIENTED_EDGE('',*,*,#8820,.F.);
#12839=ORIENTED_EDGE('',*,*,#8823,.F.);
#12840=ORIENTED_EDGE('',*,*,#8826,.F.);
#12841=ORIENTED_EDGE('',*,*,#8829,.F.);
#12842=ORIENTED_EDGE('',*,*,#8832,.F.);
#12843=ORIENTED_EDGE('',*,*,#8835,.F.);
#12844=ORIENTED_EDGE('',*,*,#8838,.F.);
#12845=ORIENTED_EDGE('',*,*,#8841,.F.);
#12846=ORIENTED_EDGE('',*,*,#8844,.F.);
#12847=ORIENTED_EDGE('',*,*,#8847,.F.);
#12848=ORIENTED_EDGE('',*,*,#8850,.F.);
#12849=ORIENTED_EDGE('',*,*,#8853,.F.);
#12850=ORIENTED_EDGE('',*,*,#8856,.F.);
#12851=ORIENTED_EDGE('',*,*,#8859,.F.);
#12852=ORIENTED_EDGE('',*,*,#8862,.F.);
#12853=ORIENTED_EDGE('',*,*,#8865,.F.);
#12854=ORIENTED_EDGE('',*,*,#8868,.F.);
#12855=ORIENTED_EDGE('',*,*,#8871,.F.);
#12856=ORIENTED_EDGE('',*,*,#8874,.F.);
#12857=ORIENTED_EDGE('',*,*,#8877,.F.);
#12858=ORIENTED_EDGE('',*,*,#8884,.F.);
#12859=ORIENTED_EDGE('',*,*,#8886,.F.);
#12860=ORIENTED_EDGE('',*,*,#8518,.F.);
#12861=ORIENTED_EDGE('',*,*,#8522,.F.);
#12862=ORIENTED_EDGE('',*,*,#8525,.F.);
#12863=ORIENTED_EDGE('',*,*,#8528,.F.);
#12864=ORIENTED_EDGE('',*,*,#8531,.F.);
#12865=ORIENTED_EDGE('',*,*,#8534,.F.);
#12866=ORIENTED_EDGE('',*,*,#8537,.F.);
#12867=ORIENTED_EDGE('',*,*,#8540,.F.);
#12868=ORIENTED_EDGE('',*,*,#8543,.F.);
#12869=ORIENTED_EDGE('',*,*,#8546,.F.);
#12870=ORIENTED_EDGE('',*,*,#8549,.F.);
#12871=ORIENTED_EDGE('',*,*,#8552,.F.);
#12872=ORIENTED_EDGE('',*,*,#8555,.F.);
#12873=ORIENTED_EDGE('',*,*,#8558,.F.);
#12874=ORIENTED_EDGE('',*,*,#8561,.F.);
#12875=ORIENTED_EDGE('',*,*,#8564,.F.);
#12876=ORIENTED_EDGE('',*,*,#8567,.F.);
#12877=ORIENTED_EDGE('',*,*,#8570,.F.);
#12878=ORIENTED_EDGE('',*,*,#8573,.F.);
#12879=ORIENTED_EDGE('',*,*,#8576,.F.);
#12880=ORIENTED_EDGE('',*,*,#8579,.F.);
#12881=ORIENTED_EDGE('',*,*,#8582,.F.);
#12882=ORIENTED_EDGE('',*,*,#8585,.F.);
#12883=ORIENTED_EDGE('',*,*,#8588,.F.);
#12884=ORIENTED_EDGE('',*,*,#8591,.F.);
#12885=ORIENTED_EDGE('',*,*,#8594,.F.);
#12886=ORIENTED_EDGE('',*,*,#8597,.F.);
#12887=ORIENTED_EDGE('',*,*,#8600,.F.);
#12888=ORIENTED_EDGE('',*,*,#8603,.F.);
#12889=ORIENTED_EDGE('',*,*,#8606,.F.);
#12890=ORIENTED_EDGE('',*,*,#8609,.F.);
#12891=ORIENTED_EDGE('',*,*,#8612,.F.);
#12892=ORIENTED_EDGE('',*,*,#8615,.F.);
#12893=ORIENTED_EDGE('',*,*,#8618,.F.);
#12894=ORIENTED_EDGE('',*,*,#8621,.F.);
#12895=ORIENTED_EDGE('',*,*,#8624,.F.);
#12896=ORIENTED_EDGE('',*,*,#8627,.F.);
#12897=ORIENTED_EDGE('',*,*,#8630,.F.);
#12898=ORIENTED_EDGE('',*,*,#8633,.F.);
#12899=ORIENTED_EDGE('',*,*,#8636,.F.);
#12900=ORIENTED_EDGE('',*,*,#8639,.F.);
#12901=ORIENTED_EDGE('',*,*,#8642,.F.);
#12902=ORIENTED_EDGE('',*,*,#8645,.F.);
#12903=ORIENTED_EDGE('',*,*,#8648,.F.);
#12904=ORIENTED_EDGE('',*,*,#8651,.F.);
#12905=ORIENTED_EDGE('',*,*,#8654,.F.);
#12906=ORIENTED_EDGE('',*,*,#8657,.F.);
#12907=ORIENTED_EDGE('',*,*,#8660,.F.);
#12908=ORIENTED_EDGE('',*,*,#8663,.F.);
#12909=ORIENTED_EDGE('',*,*,#8666,.F.);
#12910=ORIENTED_EDGE('',*,*,#8669,.F.);
#12911=ORIENTED_EDGE('',*,*,#8672,.F.);
#12912=ORIENTED_EDGE('',*,*,#8675,.F.);
#12913=ORIENTED_EDGE('',*,*,#8678,.F.);
#12914=ORIENTED_EDGE('',*,*,#8681,.F.);
#12915=ORIENTED_EDGE('',*,*,#8684,.F.);
#12916=ORIENTED_EDGE('',*,*,#8687,.F.);
#12917=ORIENTED_EDGE('',*,*,#8690,.F.);
#12918=ORIENTED_EDGE('',*,*,#8693,.F.);
#12919=ORIENTED_EDGE('',*,*,#8696,.F.);
#12920=ORIENTED_EDGE('',*,*,#8887,.F.);
#12921=ORIENTED_EDGE('',*,*,#8695,.T.);
#12922=ORIENTED_EDGE('',*,*,#8880,.T.);
#12923=ORIENTED_EDGE('',*,*,#8888,.F.);
#12924=ORIENTED_EDGE('',*,*,#8887,.T.);
#12925=ORIENTED_EDGE('',*,*,#8889,.T.);
#12926=ORIENTED_EDGE('',*,*,#8890,.T.);
#12927=ORIENTED_EDGE('',*,*,#8891,.T.);
#12928=ORIENTED_EDGE('',*,*,#8892,.T.);
#12929=ORIENTED_EDGE('',*,*,#8893,.T.);
#12930=ORIENTED_EDGE('',*,*,#8894,.T.);
#12931=ORIENTED_EDGE('',*,*,#8886,.T.);
#12932=ORIENTED_EDGE('',*,*,#8883,.T.);
#12933=ORIENTED_EDGE('',*,*,#8881,.T.);
#12934=ORIENTED_EDGE('',*,*,#8519,.F.);
#12935=ORIENTED_EDGE('',*,*,#8895,.F.);
#12936=ORIENTED_EDGE('',*,*,#8896,.F.);
#12937=ORIENTED_EDGE('',*,*,#8897,.F.);
#12938=ORIENTED_EDGE('',*,*,#8898,.F.);
#12939=ORIENTED_EDGE('',*,*,#8899,.F.);
#12940=ORIENTED_EDGE('',*,*,#8900,.F.);
#12941=ORIENTED_EDGE('',*,*,#8901,.F.);
#12942=ORIENTED_EDGE('',*,*,#8896,.T.);
#12943=ORIENTED_EDGE('',*,*,#8902,.T.);
#12944=ORIENTED_EDGE('',*,*,#8894,.F.);
#12945=ORIENTED_EDGE('',*,*,#8903,.F.);
#12946=ORIENTED_EDGE('',*,*,#8897,.T.);
#12947=ORIENTED_EDGE('',*,*,#8903,.T.);
#12948=ORIENTED_EDGE('',*,*,#8893,.F.);
#12949=ORIENTED_EDGE('',*,*,#8904,.F.);
#12950=ORIENTED_EDGE('',*,*,#8898,.T.);
#12951=ORIENTED_EDGE('',*,*,#8904,.T.);
#12952=ORIENTED_EDGE('',*,*,#8892,.F.);
#12953=ORIENTED_EDGE('',*,*,#8905,.F.);
#12954=ORIENTED_EDGE('',*,*,#8899,.T.);
#12955=ORIENTED_EDGE('',*,*,#8905,.T.);
#12956=ORIENTED_EDGE('',*,*,#8891,.F.);
#12957=ORIENTED_EDGE('',*,*,#8906,.F.);
#12958=ORIENTED_EDGE('',*,*,#8900,.T.);
#12959=ORIENTED_EDGE('',*,*,#8906,.T.);
#12960=ORIENTED_EDGE('',*,*,#8890,.F.);
#12961=ORIENTED_EDGE('',*,*,#8907,.F.);
#12962=ORIENTED_EDGE('',*,*,#8895,.T.);
#12963=ORIENTED_EDGE('',*,*,#8907,.T.);
#12964=ORIENTED_EDGE('',*,*,#8889,.F.);
#12965=ORIENTED_EDGE('',*,*,#8902,.F.);
#12966=ORIENTED_EDGE('',*,*,#8901,.T.);
#12967=ORIENTED_EDGE('',*,*,#8908,.T.);
#12968=ORIENTED_EDGE('',*,*,#8909,.F.);
#12969=ORIENTED_EDGE('',*,*,#8908,.F.);
#12970=ORIENTED_EDGE('',*,*,#8885,.T.);
#12971=ORIENTED_EDGE('',*,*,#8888,.T.);
#12972=ORIENTED_EDGE('',*,*,#8879,.T.);
#12973=ORIENTED_EDGE('',*,*,#8700,.T.);
#12974=ORIENTED_EDGE('',*,*,#8909,.T.);
#12975=ORIENTED_EDGE('',*,*,#8910,.T.);
#12976=ORIENTED_EDGE('',*,*,#8910,.F.);
#13518=PLANE('',#15380);
#13519=PLANE('',#15381);
#13520=PLANE('',#15383);
#13521=PLANE('',#15384);
#13522=PLANE('',#15385);
#13523=PLANE('',#15386);
#13524=PLANE('',#15387);
#13525=PLANE('',#15388);
#13526=PLANE('',#15391);
#14092=ADVANCED_FACE('',(#2846),#1998,.T.);
#14093=ADVANCED_FACE('',(#2847),#1999,.T.);
#14094=ADVANCED_FACE('',(#2848),#2000,.T.);
#14095=ADVANCED_FACE('',(#2849),#2001,.T.);
#14096=ADVANCED_FACE('',(#2850),#2002,.T.);
#14097=ADVANCED_FACE('',(#2851),#2003,.T.);
#14098=ADVANCED_FACE('',(#2852),#2004,.T.);
#14099=ADVANCED_FACE('',(#2853),#2005,.T.);
#14100=ADVANCED_FACE('',(#2854),#2006,.T.);
#14101=ADVANCED_FACE('',(#2855),#2007,.T.);
#14102=ADVANCED_FACE('',(#2856),#2008,.T.);
#14103=ADVANCED_FACE('',(#2857),#2009,.T.);
#14104=ADVANCED_FACE('',(#2858),#2010,.T.);
#14105=ADVANCED_FACE('',(#2859),#2011,.T.);
#14106=ADVANCED_FACE('',(#2860),#2012,.T.);
#14107=ADVANCED_FACE('',(#2861),#2013,.T.);
#14108=ADVANCED_FACE('',(#2862),#2014,.T.);
#14109=ADVANCED_FACE('',(#2863),#2015,.T.);
#14110=ADVANCED_FACE('',(#2864),#2016,.T.);
#14111=ADVANCED_FACE('',(#2865),#2017,.T.);
#14112=ADVANCED_FACE('',(#2866),#2018,.T.);
#14113=ADVANCED_FACE('',(#2867),#2019,.T.);
#14114=ADVANCED_FACE('',(#2868),#2020,.T.);
#14115=ADVANCED_FACE('',(#2869),#2021,.T.);
#14116=ADVANCED_FACE('',(#2870),#2022,.T.);
#14117=ADVANCED_FACE('',(#2871),#2023,.T.);
#14118=ADVANCED_FACE('',(#2872),#2024,.T.);
#14119=ADVANCED_FACE('',(#2873),#2025,.T.);
#14120=ADVANCED_FACE('',(#2874),#2026,.T.);
#14121=ADVANCED_FACE('',(#2875),#2027,.T.);
#14122=ADVANCED_FACE('',(#2876),#2028,.T.);
#14123=ADVANCED_FACE('',(#2877),#2029,.T.);
#14124=ADVANCED_FACE('',(#2878),#2030,.T.);
#14125=ADVANCED_FACE('',(#2879),#2031,.T.);
#14126=ADVANCED_FACE('',(#2880),#2032,.T.);
#14127=ADVANCED_FACE('',(#2881),#2033,.T.);
#14128=ADVANCED_FACE('',(#2882),#2034,.T.);
#14129=ADVANCED_FACE('',(#2883),#2035,.T.);
#14130=ADVANCED_FACE('',(#2884),#2036,.T.);
#14131=ADVANCED_FACE('',(#2885),#2037,.T.);
#14132=ADVANCED_FACE('',(#2886),#2038,.T.);
#14133=ADVANCED_FACE('',(#2887),#2039,.T.);
#14134=ADVANCED_FACE('',(#2888),#2040,.T.);
#14135=ADVANCED_FACE('',(#2889),#2041,.T.);
#14136=ADVANCED_FACE('',(#2890),#2042,.T.);
#14137=ADVANCED_FACE('',(#2891),#2043,.T.);
#14138=ADVANCED_FACE('',(#2892),#2044,.T.);
#14139=ADVANCED_FACE('',(#2893),#2045,.T.);
#14140=ADVANCED_FACE('',(#2894),#2046,.T.);
#14141=ADVANCED_FACE('',(#2895),#2047,.T.);
#14142=ADVANCED_FACE('',(#2896),#2048,.T.);
#14143=ADVANCED_FACE('',(#2897),#2049,.T.);
#14144=ADVANCED_FACE('',(#2898),#2050,.T.);
#14145=ADVANCED_FACE('',(#2899),#2051,.T.);
#14146=ADVANCED_FACE('',(#2900),#2052,.T.);
#14147=ADVANCED_FACE('',(#2901),#2053,.T.);
#14148=ADVANCED_FACE('',(#2902),#2054,.T.);
#14149=ADVANCED_FACE('',(#2903),#2055,.T.);
#14150=ADVANCED_FACE('',(#2904),#2056,.T.);
#14151=ADVANCED_FACE('',(#2905),#2057,.T.);
#14152=ADVANCED_FACE('',(#2906),#2058,.T.);
#14153=ADVANCED_FACE('',(#2907),#2059,.T.);
#14154=ADVANCED_FACE('',(#2908),#2060,.T.);
#14155=ADVANCED_FACE('',(#2909),#2061,.T.);
#14156=ADVANCED_FACE('',(#2910),#2062,.T.);
#14157=ADVANCED_FACE('',(#2911),#2063,.T.);
#14158=ADVANCED_FACE('',(#2912),#2064,.T.);
#14159=ADVANCED_FACE('',(#2913),#2065,.T.);
#14160=ADVANCED_FACE('',(#2914),#2066,.T.);
#14161=ADVANCED_FACE('',(#2915),#2067,.T.);
#14162=ADVANCED_FACE('',(#2916),#2068,.T.);
#14163=ADVANCED_FACE('',(#2917),#2069,.T.);
#14164=ADVANCED_FACE('',(#2918),#2070,.T.);
#14165=ADVANCED_FACE('',(#2919),#2071,.T.);
#14166=ADVANCED_FACE('',(#2920),#2072,.T.);
#14167=ADVANCED_FACE('',(#2921),#2073,.T.);
#14168=ADVANCED_FACE('',(#2922),#2074,.T.);
#14169=ADVANCED_FACE('',(#2923),#2075,.T.);
#14170=ADVANCED_FACE('',(#2924),#2076,.T.);
#14171=ADVANCED_FACE('',(#2925),#2077,.T.);
#14172=ADVANCED_FACE('',(#2926),#2078,.T.);
#14173=ADVANCED_FACE('',(#2927),#2079,.T.);
#14174=ADVANCED_FACE('',(#2928),#2080,.T.);
#14175=ADVANCED_FACE('',(#2929),#2081,.T.);
#14176=ADVANCED_FACE('',(#2930),#2082,.T.);
#14177=ADVANCED_FACE('',(#2931),#2083,.T.);
#14178=ADVANCED_FACE('',(#2932),#2084,.T.);
#14179=ADVANCED_FACE('',(#2933),#2085,.T.);
#14180=ADVANCED_FACE('',(#2934),#2086,.T.);
#14181=ADVANCED_FACE('',(#2935),#2087,.T.);
#14182=ADVANCED_FACE('',(#2936),#2088,.T.);
#14183=ADVANCED_FACE('',(#2937),#2089,.T.);
#14184=ADVANCED_FACE('',(#2938),#2090,.T.);
#14185=ADVANCED_FACE('',(#2939),#2091,.T.);
#14186=ADVANCED_FACE('',(#2940),#2092,.T.);
#14187=ADVANCED_FACE('',(#2941),#2093,.T.);
#14188=ADVANCED_FACE('',(#2942),#2094,.T.);
#14189=ADVANCED_FACE('',(#2943),#2095,.T.);
#14190=ADVANCED_FACE('',(#2944),#2096,.T.);
#14191=ADVANCED_FACE('',(#2945),#2097,.T.);
#14192=ADVANCED_FACE('',(#2946),#2098,.T.);
#14193=ADVANCED_FACE('',(#2947),#2099,.T.);
#14194=ADVANCED_FACE('',(#2948),#2100,.T.);
#14195=ADVANCED_FACE('',(#2949),#2101,.T.);
#14196=ADVANCED_FACE('',(#2950),#2102,.T.);
#14197=ADVANCED_FACE('',(#2951),#2103,.T.);
#14198=ADVANCED_FACE('',(#2952),#2104,.T.);
#14199=ADVANCED_FACE('',(#2953),#2105,.T.);
#14200=ADVANCED_FACE('',(#2954),#2106,.T.);
#14201=ADVANCED_FACE('',(#2955),#2107,.T.);
#14202=ADVANCED_FACE('',(#2956),#2108,.T.);
#14203=ADVANCED_FACE('',(#2957),#2109,.T.);
#14204=ADVANCED_FACE('',(#2958),#2110,.T.);
#14205=ADVANCED_FACE('',(#2959),#2111,.T.);
#14206=ADVANCED_FACE('',(#2960),#2112,.T.);
#14207=ADVANCED_FACE('',(#2961),#2113,.T.);
#14208=ADVANCED_FACE('',(#2962),#2114,.T.);
#14209=ADVANCED_FACE('',(#2963),#2115,.T.);
#14210=ADVANCED_FACE('',(#2964),#2116,.T.);
#14211=ADVANCED_FACE('',(#2965),#2117,.T.);
#14212=ADVANCED_FACE('',(#2966),#279,.F.);
#14213=ADVANCED_FACE('',(#2967),#2118,.T.);
#14214=ADVANCED_FACE('',(#2968),#280,.F.);
#14215=ADVANCED_FACE('',(#2969),#2119,.T.);
#14216=ADVANCED_FACE('',(#2970,#2293),#13518,.T.);
#14217=ADVANCED_FACE('',(#2971,#2294),#13519,.F.);
#14218=ADVANCED_FACE('',(#2972),#13520,.T.);
#14219=ADVANCED_FACE('',(#2973),#13521,.T.);
#14220=ADVANCED_FACE('',(#2974),#13522,.T.);
#14221=ADVANCED_FACE('',(#2975),#13523,.T.);
#14222=ADVANCED_FACE('',(#2976),#13524,.T.);
#14223=ADVANCED_FACE('',(#2977),#13525,.T.);
#14224=ADVANCED_FACE('',(#2978),#2120,.T.);
#14225=ADVANCED_FACE('',(#2979),#13526,.T.);
#14226=ADVANCED_FACE('',(#2980),#13,.T.);
#14320=CLOSED_SHELL('',(#14092,#14093,#14094,#14095,#14096,#14097,#14098,
#14099,#14100,#14101,#14102,#14103,#14104,#14105,#14106,#14107,#14108,#14109,
#14110,#14111,#14112,#14113,#14114,#14115,#14116,#14117,#14118,#14119,#14120,
#14121,#14122,#14123,#14124,#14125,#14126,#14127,#14128,#14129,#14130,#14131,
#14132,#14133,#14134,#14135,#14136,#14137,#14138,#14139,#14140,#14141,#14142,
#14143,#14144,#14145,#14146,#14147,#14148,#14149,#14150,#14151,#14152,#14153,
#14154,#14155,#14156,#14157,#14158,#14159,#14160,#14161,#14162,#14163,#14164,
#14165,#14166,#14167,#14168,#14169,#14170,#14171,#14172,#14173,#14174,#14175,
#14176,#14177,#14178,#14179,#14180,#14181,#14182,#14183,#14184,#14185,#14186,
#14187,#14188,#14189,#14190,#14191,#14192,#14193,#14194,#14195,#14196,#14197,
#14198,#14199,#14200,#14201,#14202,#14203,#14204,#14205,#14206,#14207,#14208,
#14209,#14210,#14211,#14212,#14213,#14214,#14215,#14216,#14217,#14218,#14219,
#14220,#14221,#14222,#14223,#14224,#14225,#14226));
#15253=AXIS2_PLACEMENT_3D('',#51545,#17626,#17627);
#15254=AXIS2_PLACEMENT_3D('',#51546,#17628,#17629);
#15255=AXIS2_PLACEMENT_3D('',#51562,#17631,#17632);
#15256=AXIS2_PLACEMENT_3D('',#51573,#17633,#17634);
#15257=AXIS2_PLACEMENT_3D('',#51621,#17636,#17637);
#15258=AXIS2_PLACEMENT_3D('',#51669,#17639,#17640);
#15259=AXIS2_PLACEMENT_3D('',#51720,#17642,#17643);
#15260=AXIS2_PLACEMENT_3D('',#51768,#17645,#17646);
#15261=AXIS2_PLACEMENT_3D('',#51816,#17648,#17649);
#15262=AXIS2_PLACEMENT_3D('',#51864,#17651,#17652);
#15263=AXIS2_PLACEMENT_3D('',#51918,#17654,#17655);
#15264=AXIS2_PLACEMENT_3D('',#51966,#17657,#17658);
#15265=AXIS2_PLACEMENT_3D('',#52014,#17660,#17661);
#15266=AXIS2_PLACEMENT_3D('',#52068,#17663,#17664);
#15267=AXIS2_PLACEMENT_3D('',#52116,#17666,#17667);
#15268=AXIS2_PLACEMENT_3D('',#52164,#17669,#17670);
#15269=AXIS2_PLACEMENT_3D('',#52215,#17672,#17673);
#15270=AXIS2_PLACEMENT_3D('',#52266,#17675,#17676);
#15271=AXIS2_PLACEMENT_3D('',#52314,#17678,#17679);
#15272=AXIS2_PLACEMENT_3D('',#52362,#17681,#17682);
#15273=AXIS2_PLACEMENT_3D('',#52416,#17684,#17685);
#15274=AXIS2_PLACEMENT_3D('',#52464,#17687,#17688);
#15275=AXIS2_PLACEMENT_3D('',#52512,#17690,#17691);
#15276=AXIS2_PLACEMENT_3D('',#52566,#17693,#17694);
#15277=AXIS2_PLACEMENT_3D('',#52614,#17696,#17697);
#15278=AXIS2_PLACEMENT_3D('',#52662,#17699,#17700);
#15279=AXIS2_PLACEMENT_3D('',#52710,#17702,#17703);
#15280=AXIS2_PLACEMENT_3D('',#52764,#17705,#17706);
#15281=AXIS2_PLACEMENT_3D('',#52812,#17708,#17709);
#15282=AXIS2_PLACEMENT_3D('',#52860,#17711,#17712);
#15283=AXIS2_PLACEMENT_3D('',#52914,#17714,#17715);
#15284=AXIS2_PLACEMENT_3D('',#52962,#17717,#17718);
#15285=AXIS2_PLACEMENT_3D('',#53010,#17720,#17721);
#15286=AXIS2_PLACEMENT_3D('',#53064,#17723,#17724);
#15287=AXIS2_PLACEMENT_3D('',#53112,#17726,#17727);
#15288=AXIS2_PLACEMENT_3D('',#53160,#17729,#17730);
#15289=AXIS2_PLACEMENT_3D('',#53208,#17732,#17733);
#15290=AXIS2_PLACEMENT_3D('',#53262,#17735,#17736);
#15291=AXIS2_PLACEMENT_3D('',#53310,#17738,#17739);
#15292=AXIS2_PLACEMENT_3D('',#53358,#17741,#17742);
#15293=AXIS2_PLACEMENT_3D('',#53412,#17744,#17745);
#15294=AXIS2_PLACEMENT_3D('',#53460,#17747,#17748);
#15295=AXIS2_PLACEMENT_3D('',#53508,#17750,#17751);
#15296=AXIS2_PLACEMENT_3D('',#53562,#17753,#17754);
#15297=AXIS2_PLACEMENT_3D('',#53610,#17756,#17757);
#15298=AXIS2_PLACEMENT_3D('',#53658,#17759,#17760);
#15299=AXIS2_PLACEMENT_3D('',#53706,#17762,#17763);
#15300=AXIS2_PLACEMENT_3D('',#53760,#17765,#17766);
#15301=AXIS2_PLACEMENT_3D('',#53808,#17768,#17769);
#15302=AXIS2_PLACEMENT_3D('',#53856,#17771,#17772);
#15303=AXIS2_PLACEMENT_3D('',#53910,#17774,#17775);
#15304=AXIS2_PLACEMENT_3D('',#53958,#17777,#17778);
#15305=AXIS2_PLACEMENT_3D('',#54006,#17780,#17781);
#15306=AXIS2_PLACEMENT_3D('',#54060,#17783,#17784);
#15307=AXIS2_PLACEMENT_3D('',#54108,#17786,#17787);
#15308=AXIS2_PLACEMENT_3D('',#54156,#17789,#17790);
#15309=AXIS2_PLACEMENT_3D('',#54204,#17792,#17793);
#15310=AXIS2_PLACEMENT_3D('',#54258,#17795,#17796);
#15311=AXIS2_PLACEMENT_3D('',#54306,#17798,#17799);
#15312=AXIS2_PLACEMENT_3D('',#54354,#17801,#17802);
#15313=AXIS2_PLACEMENT_3D('',#54408,#17804,#17805);
#15314=AXIS2_PLACEMENT_3D('',#54456,#17807,#17808);
#15315=AXIS2_PLACEMENT_3D('',#54504,#17810,#17811);
#15316=AXIS2_PLACEMENT_3D('',#54516,#17813,#17814);
#15317=AXIS2_PLACEMENT_3D('',#54522,#17815,#17816);
#15318=AXIS2_PLACEMENT_3D('',#54547,#17818,#17819);
#15319=AXIS2_PLACEMENT_3D('',#54571,#17821,#17822);
#15320=AXIS2_PLACEMENT_3D('',#54596,#17824,#17825);
#15321=AXIS2_PLACEMENT_3D('',#54621,#17827,#17828);
#15322=AXIS2_PLACEMENT_3D('',#54645,#17830,#17831);
#15323=AXIS2_PLACEMENT_3D('',#54670,#17833,#17834);
#15324=AXIS2_PLACEMENT_3D('',#54695,#17836,#17837);
#15325=AXIS2_PLACEMENT_3D('',#54719,#17839,#17840);
#15326=AXIS2_PLACEMENT_3D('',#54743,#17842,#17843);
#15327=AXIS2_PLACEMENT_3D('',#54768,#17845,#17846);
#15328=AXIS2_PLACEMENT_3D('',#54793,#17848,#17849);
#15329=AXIS2_PLACEMENT_3D('',#54817,#17851,#17852);
#15330=AXIS2_PLACEMENT_3D('',#54842,#17854,#17855);
#15331=AXIS2_PLACEMENT_3D('',#54867,#17857,#17858);
#15332=AXIS2_PLACEMENT_3D('',#54891,#17860,#17861);
#15333=AXIS2_PLACEMENT_3D('',#54916,#17863,#17864);
#15334=AXIS2_PLACEMENT_3D('',#54941,#17866,#17867);
#15335=AXIS2_PLACEMENT_3D('',#54965,#17869,#17870);
#15336=AXIS2_PLACEMENT_3D('',#54989,#17872,#17873);
#15337=AXIS2_PLACEMENT_3D('',#55014,#17875,#17876);
#15338=AXIS2_PLACEMENT_3D('',#55039,#17878,#17879);
#15339=AXIS2_PLACEMENT_3D('',#55063,#17881,#17882);
#15340=AXIS2_PLACEMENT_3D('',#55088,#17884,#17885);
#15341=AXIS2_PLACEMENT_3D('',#55113,#17887,#17888);
#15342=AXIS2_PLACEMENT_3D('',#55137,#17890,#17891);
#15343=AXIS2_PLACEMENT_3D('',#55162,#17893,#17894);
#15344=AXIS2_PLACEMENT_3D('',#55187,#17896,#17897);
#15345=AXIS2_PLACEMENT_3D('',#55211,#17899,#17900);
#15346=AXIS2_PLACEMENT_3D('',#55235,#17902,#17903);
#15347=AXIS2_PLACEMENT_3D('',#55260,#17905,#17906);
#15348=AXIS2_PLACEMENT_3D('',#55285,#17908,#17909);
#15349=AXIS2_PLACEMENT_3D('',#55309,#17911,#17912);
#15350=AXIS2_PLACEMENT_3D('',#55334,#17914,#17915);
#15351=AXIS2_PLACEMENT_3D('',#55359,#17917,#17918);
#15352=AXIS2_PLACEMENT_3D('',#55383,#17920,#17921);
#15353=AXIS2_PLACEMENT_3D('',#55408,#17923,#17924);
#15354=AXIS2_PLACEMENT_3D('',#55433,#17926,#17927);
#15355=AXIS2_PLACEMENT_3D('',#55457,#17929,#17930);
#15356=AXIS2_PLACEMENT_3D('',#55481,#17932,#17933);
#15357=AXIS2_PLACEMENT_3D('',#55506,#17935,#17936);
#15358=AXIS2_PLACEMENT_3D('',#55531,#17938,#17939);
#15359=AXIS2_PLACEMENT_3D('',#55555,#17941,#17942);
#15360=AXIS2_PLACEMENT_3D('',#55580,#17944,#17945);
#15361=AXIS2_PLACEMENT_3D('',#55605,#17947,#17948);
#15362=AXIS2_PLACEMENT_3D('',#55629,#17950,#17951);
#15363=AXIS2_PLACEMENT_3D('',#55654,#17953,#17954);
#15364=AXIS2_PLACEMENT_3D('',#55678,#17956,#17957);
#15365=AXIS2_PLACEMENT_3D('',#55703,#17959,#17960);
#15366=AXIS2_PLACEMENT_3D('',#55727,#17962,#17963);
#15367=AXIS2_PLACEMENT_3D('',#55752,#17965,#17966);
#15368=AXIS2_PLACEMENT_3D('',#55777,#17968,#17969);
#15369=AXIS2_PLACEMENT_3D('',#55801,#17971,#17972);
#15370=AXIS2_PLACEMENT_3D('',#55826,#17974,#17975);
#15371=AXIS2_PLACEMENT_3D('',#55851,#17977,#17978);
#15372=AXIS2_PLACEMENT_3D('',#55875,#17980,#17981);
#15373=AXIS2_PLACEMENT_3D('',#55900,#17983,#17984);
#15374=AXIS2_PLACEMENT_3D('',#55924,#17986,#17987);
#15375=AXIS2_PLACEMENT_3D('',#55949,#17989,#17990);
#15376=AXIS2_PLACEMENT_3D('',#57758,#17992,#17993);
#15377=AXIS2_PLACEMENT_3D('',#57760,#17994,#17995);
#15378=AXIS2_PLACEMENT_3D('',#59542,#17996,#17997);
#15379=AXIS2_PLACEMENT_3D('',#59543,#17998,#17999);
#15380=AXIS2_PLACEMENT_3D('',#59544,#18000,#18001);
#15381=AXIS2_PLACEMENT_3D('',#59557,#18008,#18009);
#15382=AXIS2_PLACEMENT_3D('',#59571,#18016,#18017);
#15383=AXIS2_PLACEMENT_3D('',#59572,#18018,#18019);
#15384=AXIS2_PLACEMENT_3D('',#59575,#18022,#18023);
#15385=AXIS2_PLACEMENT_3D('',#59577,#18025,#18026);
#15386=AXIS2_PLACEMENT_3D('',#59579,#18028,#18029);
#15387=AXIS2_PLACEMENT_3D('',#59581,#18031,#18032);
#15388=AXIS2_PLACEMENT_3D('',#59583,#18034,#18035);
#15389=AXIS2_PLACEMENT_3D('',#59584,#18036,#18037);
#15390=AXIS2_PLACEMENT_3D('',#59587,#18039,#18040);
#15391=AXIS2_PLACEMENT_3D('',#59588,#18041,#18042);
#15392=AXIS2_PLACEMENT_3D('',#59589,#18043,#18044);
#15393=AXIS2_PLACEMENT_3D('',#59591,#18045,#18046);
#17626=DIRECTION('axis',(0.,0.,1.));
#17627=DIRECTION('refdir',(1.,0.,0.));
#17628=DIRECTION('center_axis',(0.,0.,1.));
#17629=DIRECTION('ref_axis',(1.,0.,0.));
#17630=DIRECTION('',(0.,0.,-1.));
#17631=DIRECTION('center_axis',(0.,0.,-1.));
#17632=DIRECTION('ref_axis',(1.,0.,0.));
#17633=DIRECTION('center_axis',(0.,0.,1.));
#17634=DIRECTION('ref_axis',(1.,0.,0.));
#17635=DIRECTION('',(0.,0.,-1.));
#17636=DIRECTION('center_axis',(0.,0.,1.));
#17637=DIRECTION('ref_axis',(1.,0.,0.));
#17638=DIRECTION('',(0.,0.,-1.));
#17639=DIRECTION('center_axis',(0.,0.,1.));
#17640=DIRECTION('ref_axis',(1.,0.,0.));
#17641=DIRECTION('',(0.,0.,-1.));
#17642=DIRECTION('center_axis',(0.,0.,1.));
#17643=DIRECTION('ref_axis',(1.,0.,0.));
#17644=DIRECTION('',(0.,0.,-1.));
#17645=DIRECTION('center_axis',(0.,0.,1.));
#17646=DIRECTION('ref_axis',(1.,0.,0.));
#17647=DIRECTION('',(0.,0.,-1.));
#17648=DIRECTION('center_axis',(0.,0.,1.));
#17649=DIRECTION('ref_axis',(1.,0.,0.));
#17650=DIRECTION('',(0.,0.,-1.));
#17651=DIRECTION('center_axis',(0.,0.,1.));
#17652=DIRECTION('ref_axis',(1.,0.,0.));
#17653=DIRECTION('',(0.,0.,-1.));
#17654=DIRECTION('center_axis',(0.,0.,1.));
#17655=DIRECTION('ref_axis',(1.,0.,0.));
#17656=DIRECTION('',(0.,0.,-1.));
#17657=DIRECTION('center_axis',(0.,0.,1.));
#17658=DIRECTION('ref_axis',(1.,0.,0.));
#17659=DIRECTION('',(0.,0.,-1.));
#17660=DIRECTION('center_axis',(0.,0.,1.));
#17661=DIRECTION('ref_axis',(1.,0.,0.));
#17662=DIRECTION('',(0.,0.,-1.));
#17663=DIRECTION('center_axis',(0.,0.,1.));
#17664=DIRECTION('ref_axis',(1.,0.,0.));
#17665=DIRECTION('',(0.,0.,-1.));
#17666=DIRECTION('center_axis',(0.,0.,1.));
#17667=DIRECTION('ref_axis',(1.,0.,0.));
#17668=DIRECTION('',(0.,0.,-1.));
#17669=DIRECTION('center_axis',(0.,0.,1.));
#17670=DIRECTION('ref_axis',(1.,0.,0.));
#17671=DIRECTION('',(0.,0.,-1.));
#17672=DIRECTION('center_axis',(0.,0.,1.));
#17673=DIRECTION('ref_axis',(1.,0.,0.));
#17674=DIRECTION('',(0.,0.,-1.));
#17675=DIRECTION('center_axis',(0.,0.,1.));
#17676=DIRECTION('ref_axis',(1.,0.,0.));
#17677=DIRECTION('',(0.,0.,-1.));
#17678=DIRECTION('center_axis',(0.,0.,1.));
#17679=DIRECTION('ref_axis',(1.,0.,0.));
#17680=DIRECTION('',(0.,0.,-1.));
#17681=DIRECTION('center_axis',(0.,0.,1.));
#17682=DIRECTION('ref_axis',(1.,0.,0.));
#17683=DIRECTION('',(0.,0.,-1.));
#17684=DIRECTION('center_axis',(0.,0.,1.));
#17685=DIRECTION('ref_axis',(1.,0.,0.));
#17686=DIRECTION('',(0.,0.,-1.));
#17687=DIRECTION('center_axis',(0.,0.,1.));
#17688=DIRECTION('ref_axis',(1.,0.,0.));
#17689=DIRECTION('',(0.,0.,-1.));
#17690=DIRECTION('center_axis',(0.,0.,1.));
#17691=DIRECTION('ref_axis',(1.,0.,0.));
#17692=DIRECTION('',(0.,0.,-1.));
#17693=DIRECTION('center_axis',(0.,0.,1.));
#17694=DIRECTION('ref_axis',(1.,0.,0.));
#17695=DIRECTION('',(0.,0.,-1.));
#17696=DIRECTION('center_axis',(0.,0.,1.));
#17697=DIRECTION('ref_axis',(1.,0.,0.));
#17698=DIRECTION('',(0.,0.,-1.));
#17699=DIRECTION('center_axis',(0.,0.,1.));
#17700=DIRECTION('ref_axis',(1.,0.,0.));
#17701=DIRECTION('',(0.,0.,-1.));
#17702=DIRECTION('center_axis',(0.,0.,1.));
#17703=DIRECTION('ref_axis',(1.,0.,0.));
#17704=DIRECTION('',(0.,0.,-1.));
#17705=DIRECTION('center_axis',(0.,0.,1.));
#17706=DIRECTION('ref_axis',(1.,0.,0.));
#17707=DIRECTION('',(0.,0.,-1.));
#17708=DIRECTION('center_axis',(0.,0.,1.));
#17709=DIRECTION('ref_axis',(1.,0.,0.));
#17710=DIRECTION('',(0.,0.,-1.));
#17711=DIRECTION('center_axis',(0.,0.,1.));
#17712=DIRECTION('ref_axis',(1.,0.,0.));
#17713=DIRECTION('',(0.,0.,-1.));
#17714=DIRECTION('center_axis',(0.,0.,1.));
#17715=DIRECTION('ref_axis',(1.,0.,0.));
#17716=DIRECTION('',(0.,0.,-1.));
#17717=DIRECTION('center_axis',(0.,0.,1.));
#17718=DIRECTION('ref_axis',(1.,0.,0.));
#17719=DIRECTION('',(0.,0.,-1.));
#17720=DIRECTION('center_axis',(0.,0.,1.));
#17721=DIRECTION('ref_axis',(1.,0.,0.));
#17722=DIRECTION('',(0.,0.,-1.));
#17723=DIRECTION('center_axis',(0.,0.,1.));
#17724=DIRECTION('ref_axis',(1.,0.,0.));
#17725=DIRECTION('',(0.,0.,-1.));
#17726=DIRECTION('center_axis',(0.,0.,1.));
#17727=DIRECTION('ref_axis',(1.,0.,0.));
#17728=DIRECTION('',(0.,0.,-1.));
#17729=DIRECTION('center_axis',(0.,0.,1.));
#17730=DIRECTION('ref_axis',(1.,0.,0.));
#17731=DIRECTION('',(0.,0.,-1.));
#17732=DIRECTION('center_axis',(0.,0.,1.));
#17733=DIRECTION('ref_axis',(1.,0.,0.));
#17734=DIRECTION('',(0.,0.,-1.));
#17735=DIRECTION('center_axis',(0.,0.,1.));
#17736=DIRECTION('ref_axis',(1.,0.,0.));
#17737=DIRECTION('',(0.,0.,-1.));
#17738=DIRECTION('center_axis',(0.,0.,1.));
#17739=DIRECTION('ref_axis',(1.,0.,0.));
#17740=DIRECTION('',(0.,0.,-1.));
#17741=DIRECTION('center_axis',(0.,0.,1.));
#17742=DIRECTION('ref_axis',(1.,0.,0.));
#17743=DIRECTION('',(0.,0.,-1.));
#17744=DIRECTION('center_axis',(0.,0.,1.));
#17745=DIRECTION('ref_axis',(1.,0.,0.));
#17746=DIRECTION('',(0.,0.,-1.));
#17747=DIRECTION('center_axis',(0.,0.,1.));
#17748=DIRECTION('ref_axis',(1.,0.,0.));
#17749=DIRECTION('',(0.,0.,-1.));
#17750=DIRECTION('center_axis',(0.,0.,1.));
#17751=DIRECTION('ref_axis',(1.,0.,0.));
#17752=DIRECTION('',(0.,0.,-1.));
#17753=DIRECTION('center_axis',(0.,0.,1.));
#17754=DIRECTION('ref_axis',(1.,0.,0.));
#17755=DIRECTION('',(0.,0.,-1.));
#17756=DIRECTION('center_axis',(0.,0.,1.));
#17757=DIRECTION('ref_axis',(1.,0.,0.));
#17758=DIRECTION('',(0.,0.,-1.));
#17759=DIRECTION('center_axis',(0.,0.,1.));
#17760=DIRECTION('ref_axis',(1.,0.,0.));
#17761=DIRECTION('',(0.,0.,-1.));
#17762=DIRECTION('center_axis',(0.,0.,1.));
#17763=DIRECTION('ref_axis',(1.,0.,0.));
#17764=DIRECTION('',(0.,0.,-1.));
#17765=DIRECTION('center_axis',(0.,0.,1.));
#17766=DIRECTION('ref_axis',(1.,0.,0.));
#17767=DIRECTION('',(0.,0.,-1.));
#17768=DIRECTION('center_axis',(0.,0.,1.));
#17769=DIRECTION('ref_axis',(1.,0.,0.));
#17770=DIRECTION('',(0.,0.,-1.));
#17771=DIRECTION('center_axis',(0.,0.,1.));
#17772=DIRECTION('ref_axis',(1.,0.,0.));
#17773=DIRECTION('',(0.,0.,-1.));
#17774=DIRECTION('center_axis',(0.,0.,1.));
#17775=DIRECTION('ref_axis',(1.,0.,0.));
#17776=DIRECTION('',(0.,0.,-1.));
#17777=DIRECTION('center_axis',(0.,0.,1.));
#17778=DIRECTION('ref_axis',(1.,0.,0.));
#17779=DIRECTION('',(0.,0.,-1.));
#17780=DIRECTION('center_axis',(0.,0.,1.));
#17781=DIRECTION('ref_axis',(1.,0.,0.));
#17782=DIRECTION('',(0.,0.,-1.));
#17783=DIRECTION('center_axis',(0.,0.,1.));
#17784=DIRECTION('ref_axis',(1.,0.,0.));
#17785=DIRECTION('',(0.,0.,-1.));
#17786=DIRECTION('center_axis',(0.,0.,1.));
#17787=DIRECTION('ref_axis',(1.,0.,0.));
#17788=DIRECTION('',(0.,0.,-1.));
#17789=DIRECTION('center_axis',(0.,0.,1.));
#17790=DIRECTION('ref_axis',(1.,0.,0.));
#17791=DIRECTION('',(0.,0.,-1.));
#17792=DIRECTION('center_axis',(0.,0.,1.));
#17793=DIRECTION('ref_axis',(1.,0.,0.));
#17794=DIRECTION('',(0.,0.,-1.));
#17795=DIRECTION('center_axis',(0.,0.,1.));
#17796=DIRECTION('ref_axis',(1.,0.,0.));
#17797=DIRECTION('',(0.,0.,-1.));
#17798=DIRECTION('center_axis',(0.,0.,1.));
#17799=DIRECTION('ref_axis',(1.,0.,0.));
#17800=DIRECTION('',(0.,0.,-1.));
#17801=DIRECTION('center_axis',(0.,0.,1.));
#17802=DIRECTION('ref_axis',(1.,0.,0.));
#17803=DIRECTION('',(0.,0.,-1.));
#17804=DIRECTION('center_axis',(0.,0.,1.));
#17805=DIRECTION('ref_axis',(1.,0.,0.));
#17806=DIRECTION('',(0.,0.,-1.));
#17807=DIRECTION('center_axis',(0.,0.,1.));
#17808=DIRECTION('ref_axis',(1.,0.,0.));
#17809=DIRECTION('',(0.,0.,-1.));
#17810=DIRECTION('center_axis',(0.,0.,1.));
#17811=DIRECTION('ref_axis',(-0.457630590434842,-0.889142419805881,0.));
#17812=DIRECTION('',(0.,0.,1.));
#17813=DIRECTION('center_axis',(0.,0.,1.));
#17814=DIRECTION('ref_axis',(1.,-8.75189148499889E-13,0.));
#17815=DIRECTION('center_axis',(0.,0.,1.));
#17816=DIRECTION('ref_axis',(1.,-8.75189148499889E-13,0.));
#17817=DIRECTION('',(0.,0.,1.));
#17818=DIRECTION('center_axis',(0.,0.,1.));
#17819=DIRECTION('ref_axis',(1.,-8.75189148499889E-13,0.));
#17820=DIRECTION('',(0.,0.,1.));
#17821=DIRECTION('center_axis',(0.,0.,1.));
#17822=DIRECTION('ref_axis',(1.,-8.75189148499889E-13,0.));
#17823=DIRECTION('',(0.,0.,1.));
#17824=DIRECTION('center_axis',(0.,0.,1.));
#17825=DIRECTION('ref_axis',(1.,-8.75189148499889E-13,0.));
#17826=DIRECTION('',(0.,0.,1.));
#17827=DIRECTION('center_axis',(0.,0.,1.));
#17828=DIRECTION('ref_axis',(1.,-8.75189148499889E-13,0.));
#17829=DIRECTION('',(0.,0.,1.));
#17830=DIRECTION('center_axis',(0.,0.,1.));
#17831=DIRECTION('ref_axis',(1.,-8.75189148499889E-13,0.));
#17832=DIRECTION('',(0.,0.,1.));
#17833=DIRECTION('center_axis',(0.,0.,1.));
#17834=DIRECTION('ref_axis',(1.,-8.75189148499889E-13,0.));
#17835=DIRECTION('',(0.,0.,1.));
#17836=DIRECTION('center_axis',(0.,0.,1.));
#17837=DIRECTION('ref_axis',(1.,-8.75189148499889E-13,0.));
#17838=DIRECTION('',(0.,0.,1.));
#17839=DIRECTION('center_axis',(0.,0.,1.));
#17840=DIRECTION('ref_axis',(1.,-8.75189148499889E-13,0.));
#17841=DIRECTION('',(0.,0.,1.));
#17842=DIRECTION('center_axis',(0.,0.,1.));
#17843=DIRECTION('ref_axis',(1.,-8.75189148499889E-13,0.));
#17844=DIRECTION('',(0.,0.,1.));
#17845=DIRECTION('center_axis',(0.,0.,1.));
#17846=DIRECTION('ref_axis',(1.,-8.75189148499889E-13,0.));
#17847=DIRECTION('',(0.,0.,1.));
#17848=DIRECTION('center_axis',(0.,0.,1.));
#17849=DIRECTION('ref_axis',(1.,-8.75189148499889E-13,0.));
#17850=DIRECTION('',(0.,0.,1.));
#17851=DIRECTION('center_axis',(0.,0.,1.));
#17852=DIRECTION('ref_axis',(1.,-8.75189148499889E-13,0.));
#17853=DIRECTION('',(0.,0.,1.));
#17854=DIRECTION('center_axis',(0.,0.,1.));
#17855=DIRECTION('ref_axis',(1.,-8.75189148499889E-13,0.));
#17856=DIRECTION('',(0.,0.,1.));
#17857=DIRECTION('center_axis',(0.,0.,1.));
#17858=DIRECTION('ref_axis',(1.,-8.75189148499889E-13,0.));
#17859=DIRECTION('',(0.,0.,1.));
#17860=DIRECTION('center_axis',(0.,0.,1.));
#17861=DIRECTION('ref_axis',(1.,-8.75189148499889E-13,0.));
#17862=DIRECTION('',(0.,0.,1.));
#17863=DIRECTION('center_axis',(0.,0.,1.));
#17864=DIRECTION('ref_axis',(1.,-8.75189148499889E-13,0.));
#17865=DIRECTION('',(0.,0.,1.));
#17866=DIRECTION('center_axis',(0.,0.,1.));
#17867=DIRECTION('ref_axis',(1.,-8.75189148499889E-13,0.));
#17868=DIRECTION('',(0.,0.,1.));
#17869=DIRECTION('center_axis',(0.,0.,1.));
#17870=DIRECTION('ref_axis',(1.,-8.75189148499889E-13,0.));
#17871=DIRECTION('',(0.,0.,1.));
#17872=DIRECTION('center_axis',(0.,0.,1.));
#17873=DIRECTION('ref_axis',(1.,-8.75189148499889E-13,0.));
#17874=DIRECTION('',(0.,0.,1.));
#17875=DIRECTION('center_axis',(0.,0.,1.));
#17876=DIRECTION('ref_axis',(1.,-8.75189148499889E-13,0.));
#17877=DIRECTION('',(0.,0.,1.));
#17878=DIRECTION('center_axis',(0.,0.,1.));
#17879=DIRECTION('ref_axis',(1.,-8.75189148499889E-13,0.));
#17880=DIRECTION('',(0.,0.,1.));
#17881=DIRECTION('center_axis',(0.,0.,1.));
#17882=DIRECTION('ref_axis',(1.,-8.75189148499889E-13,0.));
#17883=DIRECTION('',(0.,0.,1.));
#17884=DIRECTION('center_axis',(0.,0.,1.));
#17885=DIRECTION('ref_axis',(1.,-8.75189148499889E-13,0.));
#17886=DIRECTION('',(0.,0.,1.));
#17887=DIRECTION('center_axis',(0.,0.,1.));
#17888=DIRECTION('ref_axis',(1.,-8.75189148499889E-13,0.));
#17889=DIRECTION('',(0.,0.,1.));
#17890=DIRECTION('center_axis',(0.,0.,1.));
#17891=DIRECTION('ref_axis',(1.,-8.75189148499889E-13,0.));
#17892=DIRECTION('',(0.,0.,1.));
#17893=DIRECTION('center_axis',(0.,0.,1.));
#17894=DIRECTION('ref_axis',(1.,-8.75189148499889E-13,0.));
#17895=DIRECTION('',(0.,0.,1.));
#17896=DIRECTION('center_axis',(0.,0.,1.));
#17897=DIRECTION('ref_axis',(1.,-8.75189148499889E-13,0.));
#17898=DIRECTION('',(0.,0.,1.));
#17899=DIRECTION('center_axis',(0.,0.,1.));
#17900=DIRECTION('ref_axis',(1.,-8.75189148499889E-13,0.));
#17901=DIRECTION('',(0.,0.,1.));
#17902=DIRECTION('center_axis',(0.,0.,1.));
#17903=DIRECTION('ref_axis',(1.,-8.75189148499889E-13,0.));
#17904=DIRECTION('',(0.,0.,1.));
#17905=DIRECTION('center_axis',(0.,0.,1.));
#17906=DIRECTION('ref_axis',(1.,-8.75189148499889E-13,0.));
#17907=DIRECTION('',(0.,0.,1.));
#17908=DIRECTION('center_axis',(0.,0.,1.));
#17909=DIRECTION('ref_axis',(1.,-8.75189148499889E-13,0.));
#17910=DIRECTION('',(0.,0.,1.));
#17911=DIRECTION('center_axis',(0.,0.,1.));
#17912=DIRECTION('ref_axis',(1.,-8.75189148499889E-13,0.));
#17913=DIRECTION('',(0.,0.,1.));
#17914=DIRECTION('center_axis',(0.,0.,1.));
#17915=DIRECTION('ref_axis',(1.,-8.75189148499889E-13,0.));
#17916=DIRECTION('',(0.,0.,1.));
#17917=DIRECTION('center_axis',(0.,0.,1.));
#17918=DIRECTION('ref_axis',(1.,-8.75189148499889E-13,0.));
#17919=DIRECTION('',(0.,0.,1.));
#17920=DIRECTION('center_axis',(0.,0.,1.));
#17921=DIRECTION('ref_axis',(1.,-8.75189148499889E-13,0.));
#17922=DIRECTION('',(0.,0.,1.));
#17923=DIRECTION('center_axis',(0.,0.,1.));
#17924=DIRECTION('ref_axis',(1.,-8.75189148499889E-13,0.));
#17925=DIRECTION('',(0.,0.,1.));
#17926=DIRECTION('center_axis',(0.,0.,1.));
#17927=DIRECTION('ref_axis',(1.,-8.75189148499889E-13,0.));
#17928=DIRECTION('',(0.,0.,1.));
#17929=DIRECTION('center_axis',(0.,0.,1.));
#17930=DIRECTION('ref_axis',(1.,-8.75189148499889E-13,0.));
#17931=DIRECTION('',(0.,0.,1.));
#17932=DIRECTION('center_axis',(0.,0.,1.));
#17933=DIRECTION('ref_axis',(1.,-8.75189148499889E-13,0.));
#17934=DIRECTION('',(0.,0.,1.));
#17935=DIRECTION('center_axis',(0.,0.,1.));
#17936=DIRECTION('ref_axis',(1.,-8.75189148499889E-13,0.));
#17937=DIRECTION('',(0.,0.,1.));
#17938=DIRECTION('center_axis',(0.,0.,1.));
#17939=DIRECTION('ref_axis',(1.,-8.75189148499889E-13,0.));
#17940=DIRECTION('',(0.,0.,1.));
#17941=DIRECTION('center_axis',(0.,0.,1.));
#17942=DIRECTION('ref_axis',(1.,-8.75189148499889E-13,0.));
#17943=DIRECTION('',(0.,0.,1.));
#17944=DIRECTION('center_axis',(0.,0.,1.));
#17945=DIRECTION('ref_axis',(1.,-8.75189148499889E-13,0.));
#17946=DIRECTION('',(0.,0.,1.));
#17947=DIRECTION('center_axis',(0.,0.,1.));
#17948=DIRECTION('ref_axis',(1.,-8.75189148499889E-13,0.));
#17949=DIRECTION('',(0.,0.,1.));
#17950=DIRECTION('center_axis',(0.,0.,1.));
#17951=DIRECTION('ref_axis',(1.,-8.75189148499889E-13,0.));
#17952=DIRECTION('',(0.,0.,1.));
#17953=DIRECTION('center_axis',(0.,0.,1.));
#17954=DIRECTION('ref_axis',(1.,-8.75189148499889E-13,0.));
#17955=DIRECTION('',(0.,0.,1.));
#17956=DIRECTION('center_axis',(0.,0.,1.));
#17957=DIRECTION('ref_axis',(1.,-8.75189148499889E-13,0.));
#17958=DIRECTION('',(0.,0.,1.));
#17959=DIRECTION('center_axis',(0.,0.,1.));
#17960=DIRECTION('ref_axis',(1.,-8.75189148499889E-13,0.));
#17961=DIRECTION('',(0.,0.,1.));
#17962=DIRECTION('center_axis',(0.,0.,1.));
#17963=DIRECTION('ref_axis',(1.,-8.75189148499889E-13,0.));
#17964=DIRECTION('',(0.,0.,1.));
#17965=DIRECTION('center_axis',(0.,0.,1.));
#17966=DIRECTION('ref_axis',(1.,-8.75189148499889E-13,0.));
#17967=DIRECTION('',(0.,0.,1.));
#17968=DIRECTION('center_axis',(0.,0.,1.));
#17969=DIRECTION('ref_axis',(1.,-8.75189148499889E-13,0.));
#17970=DIRECTION('',(0.,0.,1.));
#17971=DIRECTION('center_axis',(0.,0.,1.));
#17972=DIRECTION('ref_axis',(1.,-8.75189148499889E-13,0.));
#17973=DIRECTION('',(0.,0.,1.));
#17974=DIRECTION('center_axis',(0.,0.,1.));
#17975=DIRECTION('ref_axis',(1.,-8.75189148499889E-13,0.));
#17976=DIRECTION('',(0.,0.,1.));
#17977=DIRECTION('center_axis',(0.,0.,1.));
#17978=DIRECTION('ref_axis',(1.,-8.75189148499889E-13,0.));
#17979=DIRECTION('',(0.,0.,1.));
#17980=DIRECTION('center_axis',(0.,0.,1.));
#17981=DIRECTION('ref_axis',(1.,-8.75189148499889E-13,0.));
#17982=DIRECTION('',(0.,0.,1.));
#17983=DIRECTION('center_axis',(0.,0.,1.));
#17984=DIRECTION('ref_axis',(1.,-8.75189148499889E-13,0.));
#17985=DIRECTION('',(0.,0.,1.));
#17986=DIRECTION('center_axis',(0.,0.,1.));
#17987=DIRECTION('ref_axis',(1.,-8.75189148499889E-13,0.));
#17988=DIRECTION('',(0.,0.,1.));
#17989=DIRECTION('center_axis',(0.,0.,1.));
#17990=DIRECTION('ref_axis',(1.,-8.75189148499889E-13,0.));
#17991=DIRECTION('',(0.,0.,1.));
#17992=DIRECTION('center_axis',(0.,0.,1.));
#17993=DIRECTION('ref_axis',(1.,-8.75189148499889E-13,0.));
#17994=DIRECTION('center_axis',(0.,0.,-1.));
#17995=DIRECTION('ref_axis',(1.,-8.75189148499889E-13,0.));
#17996=DIRECTION('center_axis',(0.,0.,1.));
#17997=DIRECTION('ref_axis',(1.,0.,0.));
#17998=DIRECTION('center_axis',(0.,0.,-1.));
#17999=DIRECTION('ref_axis',(1.,0.,0.));
#18000=DIRECTION('center_axis',(0.,0.,1.));
#18001=DIRECTION('ref_axis',(1.,0.,0.));
#18002=DIRECTION('',(0.5,0.866025403784439,0.));
#18003=DIRECTION('',(-0.5,0.866025403784439,0.));
#18004=DIRECTION('',(-1.,1.20185167898973E-16,0.));
#18005=DIRECTION('',(-0.5,-0.866025403784439,0.));
#18006=DIRECTION('',(0.5,-0.866025403784439,0.));
#18007=DIRECTION('',(1.,-2.40370335797945E-16,0.));
#18008=DIRECTION('center_axis',(0.,0.,1.));
#18009=DIRECTION('ref_axis',(1.,0.,0.));
#18010=DIRECTION('',(0.5,0.866025403784439,0.));
#18011=DIRECTION('',(1.,-2.40370335797945E-16,0.));
#18012=DIRECTION('',(0.5,-0.866025403784439,0.));
#18013=DIRECTION('',(-0.5,-0.866025403784439,0.));
#18014=DIRECTION('',(-1.,1.20185167898973E-16,0.));
#18015=DIRECTION('',(-0.5,0.866025403784439,0.));
#18016=DIRECTION('center_axis',(0.,0.,-1.));
#18017=DIRECTION('ref_axis',(1.,0.,0.));
#18018=DIRECTION('center_axis',(-2.40370335797945E-16,-1.,0.));
#18019=DIRECTION('ref_axis',(1.,-2.40370335797945E-16,0.));
#18020=DIRECTION('',(0.,0.,1.));
#18021=DIRECTION('',(0.,0.,1.));
#18022=DIRECTION('center_axis',(-0.866025403784439,-0.5,0.));
#18023=DIRECTION('ref_axis',(0.5,-0.866025403784439,0.));
#18024=DIRECTION('',(0.,0.,1.));
#18025=DIRECTION('center_axis',(-0.866025403784439,0.5,0.));
#18026=DIRECTION('ref_axis',(-0.5,-0.866025403784439,0.));
#18027=DIRECTION('',(0.,0.,1.));
#18028=DIRECTION('center_axis',(1.20185167898973E-16,1.,0.));
#18029=DIRECTION('ref_axis',(-1.,1.20185167898973E-16,0.));
#18030=DIRECTION('',(0.,0.,1.));
#18031=DIRECTION('center_axis',(0.866025403784439,0.5,0.));
#18032=DIRECTION('ref_axis',(-0.5,0.866025403784439,0.));
#18033=DIRECTION('',(0.,0.,1.));
#18034=DIRECTION('center_axis',(0.866025403784439,-0.5,0.));
#18035=DIRECTION('ref_axis',(0.5,0.866025403784439,0.));
#18036=DIRECTION('center_axis',(0.,0.,1.));
#18037=DIRECTION('ref_axis',(1.,0.,0.));
#18038=DIRECTION('',(0.,0.,-1.));
#18039=DIRECTION('center_axis',(0.,0.,-1.));
#18040=DIRECTION('ref_axis',(1.,0.,0.));
#18041=DIRECTION('center_axis',(0.,0.,1.));
#18042=DIRECTION('ref_axis',(1.,0.,0.));
#18043=DIRECTION('center_axis',(6.12323399573677E-17,0.,1.));
#18044=DIRECTION('ref_axis',(1.,0.,0.));
#18045=DIRECTION('center_axis',(1.22464679914735E-16,-1.,0.));
#18046=DIRECTION('ref_axis',(-1.,-1.22464679914735E-16,0.));
#51545=CARTESIAN_POINT('',(0.,0.,0.));
#51546=CARTESIAN_POINT('Origin',(0.,0.,16.));
#51547=CARTESIAN_POINT('',(-4.94751652564198,0.00256483971322934,26.3223204546569));
#51548=CARTESIAN_POINT('',(-4.94433041235646,0.00147179461986118,26.1776795453432));
#51549=CARTESIAN_POINT('',(-4.942,-6.05220448138622E-16,16.));
#51550=CARTESIAN_POINT('',(2.16917135428601,4.44050218283304,26.));
#51551=CARTESIAN_POINT('Ctrl Pts',(-4.94751652564198,0.00256483971322934,
26.3223204546569));
#51552=CARTESIAN_POINT('Ctrl Pts',(-4.94869886604438,0.171401137605494,
26.3168647682864));
#51553=CARTESIAN_POINT('Ctrl Pts',(-4.9408321732254,0.340133662244093,26.311409081916));
#51554=CARTESIAN_POINT('Ctrl Pts',(-4.92355817442292,0.507901950004805,
26.3059533955455));
#51555=CARTESIAN_POINT('Ctrl Pts',(-4.75600008116697,2.13525730225587,26.2530331414635));
#51556=CARTESIAN_POINT('Ctrl Pts',(-3.70330534691493,3.67188727651734,26.2001128873815));
#51557=CARTESIAN_POINT('Ctrl Pts',(-2.24451326222463,4.41286251356918,26.1471926332996));
#51558=CARTESIAN_POINT('Ctrl Pts',(-0.892016301737719,5.09984646860033,
26.0981284221997));
#51559=CARTESIAN_POINT('Ctrl Pts',(0.80955341496604,5.10290231670094,26.0490642110999));
#51560=CARTESIAN_POINT('Ctrl Pts',(2.17574200330363,4.4448669900444,26.));
#51561=CARTESIAN_POINT('',(-2.16917135428577,4.44050218283316,26.));
#51562=CARTESIAN_POINT('Origin',(0.,0.,26.));
#51563=CARTESIAN_POINT('Ctrl Pts',(-2.16917135428577,4.44050218283316,26.));
#51564=CARTESIAN_POINT('Ctrl Pts',(-2.90742207776898,4.07986902565299,26.026460127041));
#51565=CARTESIAN_POINT('Ctrl Pts',(-3.54838487149729,3.53163056089739,26.0529202540819));
#51566=CARTESIAN_POINT('Ctrl Pts',(-4.02597159025063,2.86203897562359,26.0793803811229));
#51567=CARTESIAN_POINT('Ctrl Pts',(-4.50355830900396,2.19244739034978,26.1058405081639));
#51568=CARTESIAN_POINT('Ctrl Pts',(-4.81776895278232,1.40150268455777,26.1323006352049));
#51569=CARTESIAN_POINT('Ctrl Pts',(-4.91302280979298,0.586752670320857,
26.1587607622459));
#51570=CARTESIAN_POINT('Ctrl Pts',(-4.93572472976967,0.39257271577962,26.1650670232783));
#51571=CARTESIAN_POINT('Ctrl Pts',(-4.94598956917588,0.197040583288091,
26.1713732843108));
#51572=CARTESIAN_POINT('Ctrl Pts',(-4.94433041235646,0.00147179461986118,
26.1776795453432));
#51573=CARTESIAN_POINT('Origin',(0.,0.,16.));
#51574=CARTESIAN_POINT('',(-4.93516121822955,0.00250487983550263,27.3223204546569));
#51575=CARTESIAN_POINT('',(-4.93474635697119,0.00209204260276723,27.1776795453432));
#51576=CARTESIAN_POINT('',(-4.942,-6.05220448138622E-16,16.));
#51577=CARTESIAN_POINT('Ctrl Pts',(-4.93516121822955,0.00250487983550263,
27.3223204546569));
#51578=CARTESIAN_POINT('Ctrl Pts',(-4.93820686879495,0.665010559781625,
27.3010529594449));
#51579=CARTESIAN_POINT('Ctrl Pts',(-4.81416865933799,1.32642295622759,27.2797854642328));
#51580=CARTESIAN_POINT('Ctrl Pts',(-4.55764236207275,1.93168318346768,27.2585179690208));
#51581=CARTESIAN_POINT('Ctrl Pts',(-3.91932380623715,3.43776204663053,27.2055977149389));
#51582=CARTESIAN_POINT('Ctrl Pts',(-2.46067639950694,4.59616252449921,27.1526774608569));
#51583=CARTESIAN_POINT('Ctrl Pts',(-0.849145821918294,4.87674835967949,
27.0997572067749));
#51584=CARTESIAN_POINT('Ctrl Pts',(0.762384755670364,5.15733419485977,27.046836952693));
#51585=CARTESIAN_POINT('Ctrl Pts',(2.52679850411746,4.56010538735165,26.993916698611));
#51586=CARTESIAN_POINT('Ctrl Pts',(3.63656998987608,3.35842905030792,26.940996444529));
#51587=CARTESIAN_POINT('Ctrl Pts',(4.7463414756347,2.15675271326421,26.8880761904471));
#51588=CARTESIAN_POINT('Ctrl Pts',(5.20147069870486,0.350628846684903,26.8351559363651));
#51589=CARTESIAN_POINT('Ctrl Pts',(4.79388038130065,-1.23355926618448,26.7822356822831));
#51590=CARTESIAN_POINT('Ctrl Pts',(4.38629006389643,-2.81774737905389,26.7293154282012));
#51591=CARTESIAN_POINT('Ctrl Pts',(3.11598020601782,-4.17999973821337,26.6763951741192));
#51592=CARTESIAN_POINT('Ctrl Pts',(1.56388702368888,-4.69668637868557,26.6234749200373));
#51593=CARTESIAN_POINT('Ctrl Pts',(0.011793841359943,-5.21337301915776,
26.5705546659553));
#51594=CARTESIAN_POINT('Ctrl Pts',(-1.82208266541932,-4.88449394094269,
26.5176344118733));
#51595=CARTESIAN_POINT('Ctrl Pts',(-3.09781019267902,-3.86101403671482,
26.4647141577914));
#51596=CARTESIAN_POINT('Ctrl Pts',(-4.24201965745686,-2.94304733269382,
26.4172495900799));
#51597=CARTESIAN_POINT('Ctrl Pts',(-4.93723014327371,-1.46631393177114,
26.3697850223684));
#51598=CARTESIAN_POINT('Ctrl Pts',(-4.94751652564198,0.00256483971322934,
26.3223204546569));
#51599=CARTESIAN_POINT('Ctrl Pts',(-4.94433041235646,0.00147179461986118,
26.1776795453432));
#51600=CARTESIAN_POINT('Ctrl Pts',(-4.93206642200618,-1.44411412527272,
26.2242935383928));
#51601=CARTESIAN_POINT('Ctrl Pts',(-4.26830822622625,-2.89170283737207,
26.2709075314422));
#51602=CARTESIAN_POINT('Ctrl Pts',(-3.16027114216866,-3.81000496542323,
26.3175215244917));
#51603=CARTESIAN_POINT('Ctrl Pts',(-1.90233119357243,-4.85254131044005,
26.3704417785737));
#51604=CARTESIAN_POINT('Ctrl Pts',(-0.071770729429417,-5.21289273822024,
26.4233620326557));
#51605=CARTESIAN_POINT('Ctrl Pts',(1.48894305049924,-4.72167819128264,26.4762822867377));
#51606=CARTESIAN_POINT('Ctrl Pts',(3.0496568304279,-4.23046364434503,26.5292025408196));
#51607=CARTESIAN_POINT('Ctrl Pts',(4.34052392614221,-2.88768312268964,26.5821227949016));
#51608=CARTESIAN_POINT('Ctrl Pts',(4.77319109373772,-1.30997581823277,26.6350430489835));
#51609=CARTESIAN_POINT('Ctrl Pts',(5.20585826133323,0.267731486224089,26.6879633030655));
#51610=CARTESIAN_POINT('Ctrl Pts',(4.78032550080995,2.08036557348242,26.7408835571475));
#51611=CARTESIAN_POINT('Ctrl Pts',(3.69010138443177,3.29954694578963,26.7938038112294));
#51612=CARTESIAN_POINT('Ctrl Pts',(2.59987726805358,4.51872831809683,26.8467240653114));
#51613=CARTESIAN_POINT('Ctrl Pts',(0.844961795820489,5.14445697545292,26.8996443193934));
#51614=CARTESIAN_POINT('Ctrl Pts',(-0.770932625263734,4.88981277963295,
26.9525645734753));
#51615=CARTESIAN_POINT('Ctrl Pts',(-2.38682704634796,4.63516858381299,27.0054848275573));
#51616=CARTESIAN_POINT('Ctrl Pts',(-3.86370041628332,3.50015153481698,27.0584050816393));
#51617=CARTESIAN_POINT('Ctrl Pts',(-4.52604495623161,2.00446386165791,27.1113253357212));
#51618=CARTESIAN_POINT('Ctrl Pts',(-4.80287247849846,1.37933979454018,27.1334434055952));
#51619=CARTESIAN_POINT('Ctrl Pts',(-4.93741567156095,0.691212705388757,
27.1555614754692));
#51620=CARTESIAN_POINT('Ctrl Pts',(-4.93474635697119,0.00209204260276723,
27.1776795453432));
#51621=CARTESIAN_POINT('Origin',(0.,0.,16.));
#51622=CARTESIAN_POINT('',(-4.93883733219525,-0.00423015144557837,28.3223204546569));
#51623=CARTESIAN_POINT('',(-4.93956784471338,-0.00436622746695347,28.1776795453432));
#51624=CARTESIAN_POINT('',(-4.942,-6.05220448138622E-16,16.));
#51625=CARTESIAN_POINT('Ctrl Pts',(-4.93883733219525,-0.00423015144557837,
28.3223204546569));
#51626=CARTESIAN_POINT('Ctrl Pts',(-4.92943499320705,1.14867573667121,28.2852411506033));
#51627=CARTESIAN_POINT('Ctrl Pts',(-4.52687920768094,2.30749865084404,28.2481618465497));
#51628=CARTESIAN_POINT('Ctrl Pts',(-3.78946858460819,3.18489002165513,28.2110825424962));
#51629=CARTESIAN_POINT('Ctrl Pts',(-2.73702279222337,4.43711887162355,28.1581622884142));
#51630=CARTESIAN_POINT('Ctrl Pts',(-1.00249392936347,5.11608531143494,28.1052420343322));
#51631=CARTESIAN_POINT('Ctrl Pts',(0.62037219239006,4.91108322945104,28.0523217802503));
#51632=CARTESIAN_POINT('Ctrl Pts',(2.2432383141436,4.70608114746714,27.9994015261683));
#51633=CARTESIAN_POINT('Ctrl Pts',(3.75444169479077,3.61711054368793,27.9464812720863));
#51634=CARTESIAN_POINT('Ctrl Pts',(4.46243050532182,2.1425023369291,27.8935610180044));
#51635=CARTESIAN_POINT('Ctrl Pts',(5.17041931585287,0.667894130170271,27.8406407639224));
#51636=CARTESIAN_POINT('Ctrl Pts',(5.07519355626782,-1.19235167956817,27.7877205098404));
#51637=CARTESIAN_POINT('Ctrl Pts',(4.22033397580047,-2.58696076330049,27.7348002557585));
#51638=CARTESIAN_POINT('Ctrl Pts',(3.36547439533311,-3.98156984703282,27.6818800016765));
#51639=CARTESIAN_POINT('Ctrl Pts',(1.75098099398345,-4.91054220475902,27.6289597475946));
#51640=CARTESIAN_POINT('Ctrl Pts',(0.115662973237938,-4.94876098597613,
27.5760394935126));
#51641=CARTESIAN_POINT('Ctrl Pts',(-1.51965504750756,-4.98697976719323,
27.5231192394306));
#51642=CARTESIAN_POINT('Ctrl Pts',(-3.17579768764892,-4.13444497190124,
27.4701989853487));
#51643=CARTESIAN_POINT('Ctrl Pts',(-4.09487415524911,-2.78129895002674,
27.4172787312667));
#51644=CARTESIAN_POINT('Ctrl Pts',(-4.6445938479574,-1.97195278400361,27.3856259723968));
#51645=CARTESIAN_POINT('Ctrl Pts',(-4.9306283269799,-0.98351309398954,27.3539732135268));
#51646=CARTESIAN_POINT('Ctrl Pts',(-4.93516121822955,0.00250487983550263,
27.3223204546569));
#51647=CARTESIAN_POINT('Ctrl Pts',(-4.93474635697119,0.00209204260276723,
27.1776795453432));
#51648=CARTESIAN_POINT('Ctrl Pts',(-4.93102900187776,-0.957594843168012,
27.2084817295512));
#51649=CARTESIAN_POINT('Ctrl Pts',(-4.66120098345796,-1.91920867090262,
27.2392839137591));
#51650=CARTESIAN_POINT('Ctrl Pts',(-4.13896060662357,-2.7152702966968,27.2700860979671));
#51651=CARTESIAN_POINT('Ctrl Pts',(-3.24171600710599,-4.08295848457032,
27.3230063520491));
#51652=CARTESIAN_POINT('Ctrl Pts',(-1.59941109810958,-4.96197656299522,
27.375926606131));
#51653=CARTESIAN_POINT('Ctrl Pts',(0.0363198151755977,-4.94999037586593,
27.428846860213));
#51654=CARTESIAN_POINT('Ctrl Pts',(1.67205072846078,-4.93800418873663,27.481767114295));
#51655=CARTESIAN_POINT('Ctrl Pts',(3.30120764603473,-4.03501373605313,27.5346873683769));
#51656=CARTESIAN_POINT('Ctrl Pts',(4.17831072893992,-2.65428408264511,27.5876076224589));
#51657=CARTESIAN_POINT('Ctrl Pts',(5.0554138118451,-1.27355442923711,27.6405278765408));
#51658=CARTESIAN_POINT('Ctrl Pts',(5.18046306008153,0.584914424895401,27.6934481306228));
#51659=CARTESIAN_POINT('Ctrl Pts',(4.49620935947501,2.07068111644173,27.7463683847048));
#51660=CARTESIAN_POINT('Ctrl Pts',(3.81195565886849,3.55644780798807,27.7992886387867));
#51661=CARTESIAN_POINT('Ctrl Pts',(2.318399009419,4.66951233694822,27.8522088928687));
#51662=CARTESIAN_POINT('Ctrl Pts',(0.69902662395141,4.900507696898,27.9051291469507));
#51663=CARTESIAN_POINT('Ctrl Pts',(-0.920345761516168,5.13150305684779,
27.9580494010326));
#51664=CARTESIAN_POINT('Ctrl Pts',(-2.66553388300184,4.48042924778721,28.0109696551146));
#51665=CARTESIAN_POINT('Ctrl Pts',(-3.73791972674343,3.24523368575399,28.0638899091965));
#51666=CARTESIAN_POINT('Ctrl Pts',(-4.5065378238221,2.35992391786528,28.1018197879121));
#51667=CARTESIAN_POINT('Ctrl Pts',(-4.92952982972571,1.17454424098757,28.1397496666277));
#51668=CARTESIAN_POINT('Ctrl Pts',(-4.93956784471338,-0.00436622746695347,
28.1776795453432));
#51669=CARTESIAN_POINT('Origin',(0.,0.,16.));
#51670=CARTESIAN_POINT('',(-4.95011095070931,-1.6828919353247E-5,29.3223204546569));
#51671=CARTESIAN_POINT('',(-4.9500545842803,0.000473333830474247,29.1776795453432));
#51672=CARTESIAN_POINT('',(-4.942,-6.05220448138622E-16,16.));
#51673=CARTESIAN_POINT('Ctrl Pts',(-4.95011089075521,-1.68287949581236E-5,
29.3223204546569));
#51674=CARTESIAN_POINT('Ctrl Pts',(-4.95002830796364,1.63484509113909,29.2694293417618));
#51675=CARTESIAN_POINT('Ctrl Pts',(-4.06015814856933,3.2697840224184,29.2165382288666));
#51676=CARTESIAN_POINT('Ctrl Pts',(-2.68714856385847,4.15726245203154,29.1636471159715));
#51677=CARTESIAN_POINT('Ctrl Pts',(-1.31338249801809,5.04522985178176,29.1107268618895));
#51678=CARTESIAN_POINT('Ctrl Pts',(0.544055526265072,5.1849128728298,29.0578066078076));
#51679=CARTESIAN_POINT('Ctrl Pts',(2.03517352301083,4.51239041724249,29.0048863537256));
#51680=CARTESIAN_POINT('Ctrl Pts',(3.52629151975661,3.83986796165517,28.9519660996436));
#51681=CARTESIAN_POINT('Ctrl Pts',(4.65108948896497,2.3551400294325,28.8990458455617));
#51682=CARTESIAN_POINT('Ctrl Pts',(4.89484265904535,0.737640825291349,28.8461255914797));
#51683=CARTESIAN_POINT('Ctrl Pts',(5.13859582912572,-0.879858378849781,
28.7932053373978));
#51684=CARTESIAN_POINT('Ctrl Pts',(4.50130420007813,-2.63012885490939,28.7402850833158));
#51685=CARTESIAN_POINT('Ctrl Pts',(3.27460223530322,-3.71222015364772,28.6873648292338));
#51686=CARTESIAN_POINT('Ctrl Pts',(2.04790027052829,-4.79431145238607,28.6344445751519));
#51687=CARTESIAN_POINT('Ctrl Pts',(0.231787970026049,-5.20822357380314,
28.5815243210699));
#51688=CARTESIAN_POINT('Ctrl Pts',(-1.34265409528112,-4.76454391006902,
28.5286040669879));
#51689=CARTESIAN_POINT('Ctrl Pts',(-2.91709616058829,-4.3208642463349,28.475683812906));
#51690=CARTESIAN_POINT('Ctrl Pts',(-4.24986799070038,-3.01959279744957,
28.422763558824));
#51691=CARTESIAN_POINT('Ctrl Pts',(-4.73107254480156,-1.45621144294418,
28.369843304742));
#51692=CARTESIAN_POINT('Ctrl Pts',(-4.87511450807598,-0.988234742120547,
28.3540023547137));
#51693=CARTESIAN_POINT('Ctrl Pts',(-4.94285418164439,-0.496772420704347,
28.3381614046853));
#51694=CARTESIAN_POINT('Ctrl Pts',(-4.93883733219525,-0.00423015144557837,
28.3223204546569));
#51695=CARTESIAN_POINT('Ctrl Pts',(-4.93956784471338,-0.00436622746695347,
28.1776795453432));
#51696=CARTESIAN_POINT('Ctrl Pts',(-4.9435349971983,-0.470286790462875,
28.1926699207096));
#51697=CARTESIAN_POINT('Ctrl Pts',(-4.88300154657712,-0.935196907127989,
28.207660296076));
#51698=CARTESIAN_POINT('Ctrl Pts',(-4.75381137141076,-1.38017405347592,
28.2226506714425));
#51699=CARTESIAN_POINT('Ctrl Pts',(-4.29773360633903,-2.95106891566672,
28.2755709255244));
#51700=CARTESIAN_POINT('Ctrl Pts',(-2.98599451019808,-4.27354132504245,
28.3284911796064));
#51701=CARTESIAN_POINT('Ctrl Pts',(-1.41886776017779,-4.74240604726615,
28.3814114336883));
#51702=CARTESIAN_POINT('Ctrl Pts',(0.148258989842506,-5.21127076948986,
28.4343316877703));
#51703=CARTESIAN_POINT('Ctrl Pts',(1.97077339374215,-4.82652780456152,28.4872519418523));
#51704=CARTESIAN_POINT('Ctrl Pts',(3.21466598259635,-3.76424227707361,28.5401721959342));
#51705=CARTESIAN_POINT('Ctrl Pts',(4.45855857145055,-2.7019567495857,28.5930924500162));
#51706=CARTESIAN_POINT('Ctrl Pts',(5.1238293452593,-0.962128659538206,28.6460127040981));
#51707=CARTESIAN_POINT('Ctrl Pts',(4.90603973778863,0.659070540261458,28.6989329581801));
#51708=CARTESIAN_POINT('Ctrl Pts',(4.68825013031796,2.28026974006111,28.7518532122621));
#51709=CARTESIAN_POINT('Ctrl Pts',(3.58740014156788,3.78284004961294,28.8047734663441));
#51710=CARTESIAN_POINT('Ctrl Pts',(2.10725580021387,4.47918211041389,28.857693720426));
#51711=CARTESIAN_POINT('Ctrl Pts',(0.627111458859856,5.17552417121484,28.910613974508));
#51712=CARTESIAN_POINT('Ctrl Pts',(-1.23232723509808,5.0656379832649,28.9635342285899));
#51713=CARTESIAN_POINT('Ctrl Pts',(-2.62015287286002,4.19980926793105,29.0164544826719));
#51714=CARTESIAN_POINT('Ctrl Pts',(-4.00797851062198,3.33398055259719,29.0693747367538));
#51715=CARTESIAN_POINT('Ctrl Pts',(-4.92419109218792,1.71220930987939,29.1222949908358));
#51716=CARTESIAN_POINT('Ctrl Pts',(-4.94951767608282,0.0766427647882502,
29.1752152449178));
#51717=CARTESIAN_POINT('Ctrl Pts',(-4.94991079785034,0.0512553373413882,
29.1760366783929));
#51718=CARTESIAN_POINT('Ctrl Pts',(-4.95008927347619,0.0258645861152391,
29.1768581118681));
#51719=CARTESIAN_POINT('Ctrl Pts',(-4.9500545842803,0.000473333830474247,
29.1776795453432));
#51720=CARTESIAN_POINT('Origin',(0.,0.,16.));
#51721=CARTESIAN_POINT('',(-4.93888642291793,0.00424076360118208,30.3223204546569));
#51722=CARTESIAN_POINT('',(-4.93818673588435,0.0040670116119004,30.1776795453432));
#51723=CARTESIAN_POINT('',(-4.942,-6.05220448138622E-16,16.));
#51724=CARTESIAN_POINT('Ctrl Pts',(-4.93888642291793,0.00424076360118208,
30.3223204546569));
#51725=CARTESIAN_POINT('Ctrl Pts',(-4.94290141421135,0.49495855667818,30.3065377870022));
#51726=CARTESIAN_POINT('Ctrl Pts',(-4.87566910369714,0.984600773625852,
30.2907551193474));
#51727=CARTESIAN_POINT('Ctrl Pts',(-4.7326693925228,1.45101307944963,30.2749724516927));
#51728=CARTESIAN_POINT('Ctrl Pts',(-4.25318257733109,3.01492218981842,30.2220521976108));
#51729=CARTESIAN_POINT('Ctrl Pts',(-2.92184129195003,4.31765692360063,30.1691319435288));
#51730=CARTESIAN_POINT('Ctrl Pts',(-1.3478876419775,4.76306597049205,30.1162116894468));
#51731=CARTESIAN_POINT('Ctrl Pts',(0.226066007995039,5.20847501738348,30.0632914353649));
#51732=CARTESIAN_POINT('Ctrl Pts',(2.04263202255905,4.79655837738413,30.0103711812829));
#51733=CARTESIAN_POINT('Ctrl Pts',(3.27052205003055,3.71581539574951,29.9574509272009));
#51734=CARTESIAN_POINT('Ctrl Pts',(4.49841207750204,2.6350724141149,29.904530673119));
#51735=CARTESIAN_POINT('Ctrl Pts',(5.13762611788102,0.885503090845023,29.851610419037));
#51736=CARTESIAN_POINT('Ctrl Pts',(4.89565006291192,-0.732262930536752,
29.798690164955));
#51737=CARTESIAN_POINT('Ctrl Pts',(4.65367400794282,-2.35002895191851,29.7457699108731));
#51738=CARTESIAN_POINT('Ctrl Pts',(3.53050785762567,-3.83599167141216,29.6928496567911));
#51739=CARTESIAN_POINT('Ctrl Pts',(2.04012959776072,-4.51015185496902,29.6399294027091));
#51740=CARTESIAN_POINT('Ctrl Pts',(0.549751337895761,-5.18431203852589,
29.5870091486272));
#51741=CARTESIAN_POINT('Ctrl Pts',(-1.307839031517,-5.04666968614595,29.5340888945452));
#51742=CARTESIAN_POINT('Ctrl Pts',(-2.68257979015076,-4.16021203843222,
29.4811686404633));
#51743=CARTESIAN_POINT('Ctrl Pts',(-4.05807756664059,-3.27326625194488,
29.4282192451945));
#51744=CARTESIAN_POINT('Ctrl Pts',(-4.95019356454733,-1.6366802542765,29.3752698499257));
#51745=CARTESIAN_POINT('Ctrl Pts',(-4.95011089075521,-1.68287949581236E-5,
29.3223204546569));
#51746=CARTESIAN_POINT('Ctrl Pts',(-4.9500545842803,0.000473333830474247,
29.1776795453432));
#51747=CARTESIAN_POINT('Ctrl Pts',(-4.94785444726563,-1.60994837137546,
29.2297783659501));
#51748=CARTESIAN_POINT('Ctrl Pts',(-4.08816932384676,-3.22238565418073,
29.2818771865568));
#51749=CARTESIAN_POINT('Ctrl Pts',(-2.74893267905414,-4.11666957233305,
29.3339760071636));
#51750=CARTESIAN_POINT('Ctrl Pts',(-1.38858051190673,-5.0250535168987,29.3868962612456));
#51751=CARTESIAN_POINT('Ctrl Pts',(0.466564408611941,-5.19245955856552,
29.4398165153276));
#51752=CARTESIAN_POINT('Ctrl Pts',(1.96755945318719,-4.54228015350161,29.4927367694096));
#51753=CARTESIAN_POINT('Ctrl Pts',(3.46855449776245,-3.8921007484377,29.5456570234915));
#51754=CARTESIAN_POINT('Ctrl Pts',(4.61539966639428,-2.42433589664307,29.5985772775735));
#51755=CARTESIAN_POINT('Ctrl Pts',(4.88328108437524,-0.810657201852559,
29.6514975316554));
#51756=CARTESIAN_POINT('Ctrl Pts',(5.15116250235621,0.803021492937955,29.7044177857374));
#51757=CARTESIAN_POINT('Ctrl Pts',(4.54008016968629,2.56261403072434,29.7573380398194));
#51758=CARTESIAN_POINT('Ctrl Pts',(3.3296746999557,3.66290398769728,29.8102582939013));
#51759=CARTESIAN_POINT('Ctrl Pts',(2.11926923022511,4.76319394467022,29.8631785479833));
#51760=CARTESIAN_POINT('Ctrl Pts',(0.309540623433855,5.20418132082974,29.9160988020653));
#51761=CARTESIAN_POINT('Ctrl Pts',(-1.27135167326916,4.78406356027939,29.9690190561472));
#51762=CARTESIAN_POINT('Ctrl Pts',(-2.85224396997218,4.36394579972904,30.0219393102292));
#51763=CARTESIAN_POINT('Ctrl Pts',(-4.20429995658695,3.0827229024688,30.0748595643112));
#51764=CARTESIAN_POINT('Ctrl Pts',(-4.70879816265426,1.5267020327104,30.1277798183931));
#51765=CARTESIAN_POINT('Ctrl Pts',(-4.86736582366476,1.03763272218799,30.1444130607098));
#51766=CARTESIAN_POINT('Ctrl Pts',(-4.94220382950374,0.521416307353422,
30.1610463030265));
#51767=CARTESIAN_POINT('Ctrl Pts',(-4.93818673588435,0.0040670116119004,
30.1776795453432));
#51768=CARTESIAN_POINT('Origin',(0.,0.,16.));
#51769=CARTESIAN_POINT('',(-4.9351415428321,-0.00248504100164359,31.3223204546569));
#51770=CARTESIAN_POINT('',(-4.93557330743154,-0.0028385321285674,31.1776795453432));
#51771=CARTESIAN_POINT('',(-4.942,-6.05220448138622E-16,16.));
#51772=CARTESIAN_POINT('Ctrl Pts',(-4.9351415428321,-0.00248504100164359,
31.3223204546569));
#51773=CARTESIAN_POINT('Ctrl Pts',(-4.93066017409234,0.981733357670619,
31.2907259781606));
#51774=CARTESIAN_POINT('Ctrl Pts',(-4.6457448695693,1.96834170751759,31.2591315016643));
#51775=CARTESIAN_POINT('Ctrl Pts',(-4.09792294976925,2.77680140323666,31.227537025168));
#51776=CARTESIAN_POINT('Ctrl Pts',(-3.18032980050788,4.13095875151604,31.1746167710861));
#51777=CARTESIAN_POINT('Ctrl Pts',(-1.52513305096331,4.98530711426681,31.1216965170041));
#51778=CARTESIAN_POINT('Ctrl Pts',(0.110223986946674,4.94888363249201,31.0687762629222));
#51779=CARTESIAN_POINT('Ctrl Pts',(1.74558102485669,4.91246015071721,31.0158560088402));
#51780=CARTESIAN_POINT('Ctrl Pts',(3.36109835113211,3.98526482441679,30.9629357547582));
#51781=CARTESIAN_POINT('Ctrl Pts',(4.2174905639687,2.59159639567501,30.9100155006763));
#51782=CARTESIAN_POINT('Ctrl Pts',(5.0738827768053,1.19792796693324,30.8570952465943));
#51783=CARTESIAN_POINT('Ctrl Pts',(5.17114987620307,-0.662213564249888,
30.8041749925123));
#51784=CARTESIAN_POINT('Ctrl Pts',(4.46478095192916,-2.13759902381238,30.7512547384304));
#51785=CARTESIAN_POINT('Ctrl Pts',(3.75841202765526,-3.61298448337487,30.6983344843484));
#51786=CARTESIAN_POINT('Ctrl Pts',(2.2484070797097,-4.70361387131672,30.6454142302665));
#51787=CARTESIAN_POINT('Ctrl Pts',(0.625767434156371,-4.91039852288288,
30.5924939761845));
#51788=CARTESIAN_POINT('Ctrl Pts',(-0.996872211396971,-5.11718317444904,
30.5395737221025));
#51789=CARTESIAN_POINT('Ctrl Pts',(-2.73214655455809,-4.44012308963949,
30.4866534680206));
#51790=CARTESIAN_POINT('Ctrl Pts',(-3.78596755363747,-3.18905130375701,
30.4337332139386));
#51791=CARTESIAN_POINT('Ctrl Pts',(-4.52550233311024,-2.31109280977609,
30.3965956275114));
#51792=CARTESIAN_POINT('Ctrl Pts',(-4.92943890178742,-1.1504483453926,30.3594580410841));
#51793=CARTESIAN_POINT('Ctrl Pts',(-4.93888642291793,0.00424076360118208,
30.3223204546569));
#51794=CARTESIAN_POINT('Ctrl Pts',(-4.93818673588435,0.0040670116119004,
30.1776795453432));
#51795=CARTESIAN_POINT('Ctrl Pts',(-4.92942306127099,-1.12458004491972,
30.2139665571085));
#51796=CARTESIAN_POINT('Ctrl Pts',(-4.54535955813864,-2.25861888984588,
30.2502535688737));
#51797=CARTESIAN_POINT('Ctrl Pts',(-3.83660874069347,-3.12794382961597,
30.286540580639));
#51798=CARTESIAN_POINT('Ctrl Pts',(-2.80298068714555,-4.39574997992736,
30.339460834721));
#51799=CARTESIAN_POINT('Ctrl Pts',(-1.0787841545299,-5.10054343829356,30.3923810888029));
#51800=CARTESIAN_POINT('Ctrl Pts',(0.546962191086786,-4.91979995442398,
30.4453013428849));
#51801=CARTESIAN_POINT('Ctrl Pts',(2.17270853670347,-4.73905647055441,30.4982215969669));
#51802=CARTESIAN_POINT('Ctrl Pts',(3.7000046953212,-3.67277604444905,30.5511418510488));
#51803=CARTESIAN_POINT('Ctrl Pts',(4.4299366186172,-2.20890488388769,30.6040621051308));
#51804=CARTESIAN_POINT('Ctrl Pts',(5.1598685419132,-0.745033723326325,30.6569823592128));
#51805=CARTESIAN_POINT('Ctrl Pts',(5.09243622988746,1.11642817169105,30.7099026132947));
#51806=CARTESIAN_POINT('Ctrl Pts',(4.25849773850338,2.52364740836047,30.7628228673767));
#51807=CARTESIAN_POINT('Ctrl Pts',(3.42455924711931,3.93086664502988,30.8157431214587));
#51808=CARTESIAN_POINT('Ctrl Pts',(1.8241145763769,4.88384322335134,30.8686633755406));
#51809=CARTESIAN_POINT('Ctrl Pts',(0.189551650661496,4.9464805066113,30.9215836296226));
#51810=CARTESIAN_POINT('Ctrl Pts',(-1.44501127505389,5.00911778987126,30.9745038837045));
#51811=CARTESIAN_POINT('Ctrl Pts',(-3.11369245574226,4.18141577806974,31.0274241377865));
#51812=CARTESIAN_POINT('Ctrl Pts',(-4.05287789782628,2.84214355302423,31.0803443918685));
#51813=CARTESIAN_POINT('Ctrl Pts',(-4.62868616337827,2.0210447769463,31.1127894430267));
#51814=CARTESIAN_POINT('Ctrl Pts',(-4.93028912913986,1.0076552769297,31.145234494185));
#51815=CARTESIAN_POINT('Ctrl Pts',(-4.93557330743154,-0.0028385321285674,
31.1776795453432));
#51816=CARTESIAN_POINT('Origin',(0.,0.,16.));
#51817=CARTESIAN_POINT('',(-4.94795422753399,-0.0028972882267797,32.3223204546569));
#51818=CARTESIAN_POINT('',(-4.94851874366221,-0.00251525819571033,32.1776795453432));
#51819=CARTESIAN_POINT('',(-4.942,-6.05220448138622E-16,16.));
#51820=CARTESIAN_POINT('Ctrl Pts',(-4.94795422753399,-0.0028972882267797,
32.3223204546569));
#51821=CARTESIAN_POINT('Ctrl Pts',(-4.93774012235113,1.46412544671205,32.2749141693191));
#51822=CARTESIAN_POINT('Ctrl Pts',(-4.24380482164535,2.93954073272814,32.2275078839812));
#51823=CARTESIAN_POINT('Ctrl Pts',(-3.10183998936669,3.85774379859783,32.1801015986434));
#51824=CARTESIAN_POINT('Ctrl Pts',(-1.82704976595674,4.88274584628794,32.1271813445614));
#51825=CARTESIAN_POINT('Ctrl Pts',(0.00605460139836145,5.21337522038518,
32.0742610904795));
#51826=CARTESIAN_POINT('Ctrl Pts',(1.55861655774584,4.69833086969986,32.0213408363975));
#51827=CARTESIAN_POINT('Ctrl Pts',(3.11117851409333,4.18328651901453,31.9684205823155));
#51828=CARTESIAN_POINT('Ctrl Pts',(4.38319805943319,2.82256844354664,31.9155003282335));
#51829=CARTESIAN_POINT('Ctrl Pts',(4.79257962264663,1.23886201646757,31.8625800741516));
#51830=CARTESIAN_POINT('Ctrl Pts',(5.20196118586006,-0.344844410611489,
31.8096598200696));
#51831=CARTESIAN_POINT('Ctrl Pts',(4.74870476694708,-2.15153918930172,31.7567395659877));
#51832=CARTESIAN_POINT('Ctrl Pts',(3.64022742565071,-3.35445119576896,31.7038193119057));
#51833=CARTESIAN_POINT('Ctrl Pts',(2.53175008435434,-4.5573632022362,31.6508990578238));
#51834=CARTESIAN_POINT('Ctrl Pts',(0.768051820674579,-5.15649243648045,
31.5979788037418));
#51835=CARTESIAN_POINT('Ctrl Pts',(-0.843772103495588,-4.87766821059161,
31.5450585496598));
#51836=CARTESIAN_POINT('Ctrl Pts',(-2.45559602766576,-4.59884398470276,
31.4921382955779));
#51837=CARTESIAN_POINT('Ctrl Pts',(-3.91554561232635,-3.44206629868081,
31.4392180414959));
#51838=CARTESIAN_POINT('Ctrl Pts',(-4.55552563016757,-1.93669428876581,
31.386297787414));
#51839=CARTESIAN_POINT('Ctrl Pts',(-4.81342445844275,-1.33006022730727,
31.3649720098283));
#51840=CARTESIAN_POINT('Ctrl Pts',(-4.93816639665535,-0.66681706968053,
31.3436462322426));
#51841=CARTESIAN_POINT('Ctrl Pts',(-4.9351415428321,-0.00248504100164359,
31.3223204546569));
#51842=CARTESIAN_POINT('Ctrl Pts',(-4.93557330743154,-0.0028385321285674,
31.1776795453432));
#51843=CARTESIAN_POINT('Ctrl Pts',(-4.93890801084376,-0.640534114505631,
31.1981547482669));
#51844=CARTESIAN_POINT('Ctrl Pts',(-4.82423274680824,-1.27707647808528,
31.2186299511906));
#51845=CARTESIAN_POINT('Ctrl Pts',(-4.58598979744053,-1.86340999470999,
31.2391051541143));
#51846=CARTESIAN_POINT('Ctrl Pts',(-3.97022655149108,-3.3788488791092,31.2920254081963));
#51847=CARTESIAN_POINT('Ctrl Pts',(-2.5290103561125,-4.55888420961813,31.3449456622783));
#51848=CARTESIAN_POINT('Ctrl Pts',(-0.921863753563045,-4.86351379667883,
31.3978659163602));
#51849=CARTESIAN_POINT('Ctrl Pts',(0.685282848986421,-5.16814338373953,
31.4507861704422));
#51850=CARTESIAN_POINT('Ctrl Pts',(2.45835985870677,-4.59736722735202,31.5037064245242));
#51851=CARTESIAN_POINT('Ctrl Pts',(3.5859801562746,-3.4123812139678,31.5566266786061));
#51852=CARTESIAN_POINT('Ctrl Pts',(4.71360045384243,-2.22739520058358,31.6095469326881));
#51853=CARTESIAN_POINT('Ctrl Pts',(5.19576403925773,-0.428199330202661,
31.6624671867701));
#51854=CARTESIAN_POINT('Ctrl Pts',(4.81182549189739,1.16186688830996,31.715387440852));
#51855=CARTESIAN_POINT('Ctrl Pts',(4.42788694453706,2.75193310682255,31.768307694934));
#51856=CARTESIAN_POINT('Ctrl Pts',(3.17784626440109,4.13286967346687,31.8212279490159));
#51857=CARTESIAN_POINT('Ctrl Pts',(1.63374115821347,4.67273892471915,31.8741482030979));
#51858=CARTESIAN_POINT('Ctrl Pts',(0.0896360520258116,5.21260817597145,
31.9270684571799));
#51859=CARTESIAN_POINT('Ctrl Pts',(-1.74853348021352,4.91141011183171,31.9799887112618));
#51860=CARTESIAN_POINT('Ctrl Pts',(-3.0395929867415,3.90697756655707,32.0329089653438));
#51861=CARTESIAN_POINT('Ctrl Pts',(-4.21688283424399,2.99105678050979,32.0811658253436));
#51862=CARTESIAN_POINT('Ctrl Pts',(-4.93923809973741,1.49038033345358,32.1294226853434));
#51863=CARTESIAN_POINT('Ctrl Pts',(-4.94851874366221,-0.00251525819571033,
32.1776795453432));
#51864=CARTESIAN_POINT('Origin',(0.,0.,16.));
#51865=CARTESIAN_POINT('',(-4.94391378591308,0.00432614989180041,33.3223204546569));
#51866=CARTESIAN_POINT('',(-4.943114998001,0.00443591996608837,33.1776795453432));
#51867=CARTESIAN_POINT('',(-4.942,-6.05220448138622E-16,16.));
#51868=CARTESIAN_POINT('Ctrl Pts',(-4.94391378591308,0.00432614989180041,
33.3223204546569));
#51869=CARTESIAN_POINT('Ctrl Pts',(-4.94684012248784,0.323678273041629,
33.3120226145595));
#51870=CARTESIAN_POINT('Ctrl Pts',(-4.91854579890533,0.642514059921896,
33.3017247744621));
#51871=CARTESIAN_POINT('Ctrl Pts',(-4.8571468315969,0.954841972036427,33.2914269343646));
#51872=CARTESIAN_POINT('Ctrl Pts',(-4.54161960262542,2.55988461298029,33.2385066802827));
#51873=CARTESIAN_POINT('Ctrl Pts',(-3.3518326489115,3.99306094874791,33.1855864262007));
#51874=CARTESIAN_POINT('Ctrl Pts',(-1.83225065173251,4.59852759962142,33.1326661721187));
#51875=CARTESIAN_POINT('Ctrl Pts',(-0.312668654553525,5.20399425049493,
33.0797459180367));
#51876=CARTESIAN_POINT('Ctrl Pts',(1.53670838609054,4.98175121647435,33.0268256639548));
#51877=CARTESIAN_POINT('Ctrl Pts',(2.86957729142234,4.03350030417842,32.9739054098728));
#51878=CARTESIAN_POINT('Ctrl Pts',(4.20244619675414,3.0852493918825,32.9209851557909));
#51879=CARTESIAN_POINT('Ctrl Pts',(5.01880696677368,1.41099060131123,32.8680649017089));
#51880=CARTESIAN_POINT('Ctrl Pts',(4.94508044508782,-0.223109674519649,
32.8151446476269));
#51881=CARTESIAN_POINT('Ctrl Pts',(4.87135392340196,-1.85720995035054,32.762224393545));
#51882=CARTESIAN_POINT('Ctrl Pts',(3.90754011001068,-3.45115171144104,32.709304139463));
#51883=CARTESIAN_POINT('Ctrl Pts',(2.49469492595997,-4.27552286412362,32.6563838853811));
#51884=CARTESIAN_POINT('Ctrl Pts',(1.08184974190924,-5.0998940168062,32.6034636312991));
#51885=CARTESIAN_POINT('Ctrl Pts',(-0.780026812800927,-5.15469456108083,
32.5505433772171));
#51886=CARTESIAN_POINT('Ctrl Pts',(-2.2389115908552,-4.41484693093525,32.4976231231352));
#51887=CARTESIAN_POINT('Ctrl Pts',(-3.69779636890945,-3.67499930078968,
32.4447028690532));
#51888=CARTESIAN_POINT('Ctrl Pts',(-4.75368937030783,-2.14050349622394,
32.3917826149712));
#51889=CARTESIAN_POINT('Ctrl Pts',(-4.92339783127462,-0.513568233299591,
32.3388623608893));
#51890=CARTESIAN_POINT('Ctrl Pts',(-4.94108042115667,-0.344051469933491,
32.3333483921451));
#51891=CARTESIAN_POINT('Ctrl Pts',(-4.94914226106849,-0.173531149322059,
32.327834423401));
#51892=CARTESIAN_POINT('Ctrl Pts',(-4.94795422753399,-0.0028972882267797,
32.3223204546569));
#51893=CARTESIAN_POINT('Ctrl Pts',(-4.94851874366221,-0.00251525819571033,
32.1776795453432));
#51894=CARTESIAN_POINT('Ctrl Pts',(-4.94941559646112,-0.146784082719192,
32.1823429394254));
#51895=CARTESIAN_POINT('Ctrl Pts',(-4.9436532640282,-0.290980244219974,
32.1870063335075));
#51896=CARTESIAN_POINT('Ctrl Pts',(-4.93099878465363,-0.434569000702025,
32.1916697275897));
#51897=CARTESIAN_POINT('Ctrl Pts',(-4.78739559522113,-2.06401599627693,
32.2445899816717));
#51898=CARTESIAN_POINT('Ctrl Pts',(-3.75623973553951,-3.61524296101718,
32.2975102357536));
#51899=CARTESIAN_POINT('Ctrl Pts',(-2.30940387553184,-4.3783847444355,32.3504304898356));
#51900=CARTESIAN_POINT('Ctrl Pts',(-0.862568015524189,-5.14152652785381,
32.4033507439175));
#51901=CARTESIAN_POINT('Ctrl Pts',(0.999947844809495,-5.11658312995021,
32.4562709979995));
#51902=CARTESIAN_POINT('Ctrl Pts',(2.4258280021366,-4.3149690305583,32.5091912520815));
#51903=CARTESIAN_POINT('Ctrl Pts',(3.85170815946372,-3.51335493116639,32.5621115061634));
#51904=CARTESIAN_POINT('Ctrl Pts',(4.84095261378425,-1.93507013028614,32.6150317602454));
#51905=CARTESIAN_POINT('Ctrl Pts',(4.9408679943685,-0.30236185746891,32.6679520143274));
#51906=CARTESIAN_POINT('Ctrl Pts',(5.04078337495275,1.33034641534833,32.7208722684093));
#51907=CARTESIAN_POINT('Ctrl Pts',(4.25136968180072,3.01747816010256,32.7737925224913));
#51908=CARTESIAN_POINT('Ctrl Pts',(2.93387467737636,3.9869761233392,32.8267127765732));
#51909=CARTESIAN_POINT('Ctrl Pts',(1.616379672952,4.95647408657584,32.8796330306552));
#51910=CARTESIAN_POINT('Ctrl Pts',(-0.229196642744684,5.20833826829488,
32.9325532847372));
#51911=CARTESIAN_POINT('Ctrl Pts',(-1.75829036071957,4.62731177229585,32.9854735388191));
#51912=CARTESIAN_POINT('Ctrl Pts',(-3.28738407869442,4.04628527629685,33.0383937929011));
#51913=CARTESIAN_POINT('Ctrl Pts',(-4.49999519894748,2.63236810257984,33.091314046983));
#51914=CARTESIAN_POINT('Ctrl Pts',(-4.8412143530065,1.03259034416892,33.144234301065));
#51915=CARTESIAN_POINT('Ctrl Pts',(-4.91309708900794,0.695574086725974,
33.1553827158244));
#51916=CARTESIAN_POINT('Ctrl Pts',(-4.94630788623483,0.350309429675576,
33.1665311305838));
#51917=CARTESIAN_POINT('Ctrl Pts',(-4.943114998001,0.00443591996608837,
33.1776795453432));
#51918=CARTESIAN_POINT('Origin',(0.,0.,16.));
#51919=CARTESIAN_POINT('',(-4.93390856647989,0.000179243442527399,34.3223204546569));
#51920=CARTESIAN_POINT('',(-4.93391474235666,-0.000255694835337854,34.1776795453433));
#51921=CARTESIAN_POINT('',(-4.942,-6.05220448138622E-16,16.));
#51922=CARTESIAN_POINT('Ctrl Pts',(-4.93390856647989,0.000179243442527399,
34.3223204546569));
#51923=CARTESIAN_POINT('Ctrl Pts',(-4.93417188922503,0.81404442559312,34.2962108057179));
#51924=CARTESIAN_POINT('Ctrl Pts',(-4.7439659144325,1.62779374632659,34.2701011567789));
#51925=CARTESIAN_POINT('Ctrl Pts',(-4.36261434797766,2.33905848282458,34.24399150784));
#51926=CARTESIAN_POINT('Ctrl Pts',(-3.58967320891792,3.780683020289,34.191071253758));
#51927=CARTESIAN_POINT('Ctrl Pts',(-2.03148547319181,4.80128989115793,34.138150999676));
#51928=CARTESIAN_POINT('Ctrl Pts',(-0.401101646399658,4.93383380390034,
34.0852307455941));
#51929=CARTESIAN_POINT('Ctrl Pts',(1.22928218039249,5.06637771664275,34.0323104915121));
#51930=CARTESIAN_POINT('Ctrl Pts',(2.93186209825069,4.31085867125863,33.9793902374301));
#51931=CARTESIAN_POINT('Ctrl Pts',(3.92751153377263,3.01301372173064,33.9264699833482));
#51932=CARTESIAN_POINT('Ctrl Pts',(4.92316096929458,1.71516877220265,33.8735497292662));
#51933=CARTESIAN_POINT('Ctrl Pts',(5.21187992248028,-0.125002081469193,
33.8206294751842));
#51934=CARTESIAN_POINT('Ctrl Pts',(4.66154619083434,-1.6654085522694,33.7677092211023));
#51935=CARTESIAN_POINT('Ctrl Pts',(4.1112124591884,-3.2058150230696,33.7147889670203));
#51936=CARTESIAN_POINT('Ctrl Pts',(2.72182604271081,-4.44645711099814,33.6618687129384));
#51937=CARTESIAN_POINT('Ctrl Pts',(1.12919138526205,-4.8195980486659,33.6089484588564));
#51938=CARTESIAN_POINT('Ctrl Pts',(-0.463443272186686,-5.19273898633366,
33.5560282047744));
#51939=CARTESIAN_POINT('Ctrl Pts',(-2.25932617060659,-4.69837877374066,
33.5031079506925));
#51940=CARTESIAN_POINT('Ctrl Pts',(-3.43663386770201,-3.56274419438412,
33.4501876966105));
#51941=CARTESIAN_POINT('Ctrl Pts',(-4.384847305511,-2.64809463314952,33.407565282626));
#51942=CARTESIAN_POINT('Ctrl Pts',(-4.93180177720373,-1.3174615522823,33.3649428686414));
#51943=CARTESIAN_POINT('Ctrl Pts',(-4.94391378591308,0.00432614989180041,
33.3223204546569));
#51944=CARTESIAN_POINT('Ctrl Pts',(-4.943114998001,0.00443591996608837,
33.1776795453432));
#51945=CARTESIAN_POINT('Ctrl Pts',(-4.93115160973848,-1.2915126956278,33.2194513846658));
#51946=CARTESIAN_POINT('Ctrl Pts',(-4.40811124636647,-2.59600908794704,
33.2612232239884));
#51947=CARTESIAN_POINT('Ctrl Pts',(-3.49331109260409,-3.50718930782419,
33.3029950633109));
#51948=CARTESIAN_POINT('Ctrl Pts',(-2.33436149027767,-4.6615528583015,33.3559153173929));
#51949=CARTESIAN_POINT('Ctrl Pts',(-0.54663509775989,-5.18464161615124,
33.4088355714748));
#51950=CARTESIAN_POINT('Ctrl Pts',(1.0517771843263,-4.83708217680429,33.4617558255568));
#51951=CARTESIAN_POINT('Ctrl Pts',(2.65018946641248,-4.48952273745735,33.5146760796387));
#51952=CARTESIAN_POINT('Ctrl Pts',(4.05928763806706,-3.27131510091373,33.5675963337207));
#51953=CARTESIAN_POINT('Ctrl Pts',(4.63424685520885,-1.73992968697417,33.6205165878027));
#51954=CARTESIAN_POINT('Ctrl Pts',(5.20920607235062,-0.208544273034641,
33.6734368418847));
#51955=CARTESIAN_POINT('Ctrl Pts',(4.95002633497964,1.63601891830083,33.7263570959666));
#51956=CARTESIAN_POINT('Ctrl Pts',(3.97531224929094,2.94965959921896,33.7792773500486));
#51957=CARTESIAN_POINT('Ctrl Pts',(3.00059816360222,4.26330028013712,33.8321976041305));
#51958=CARTESIAN_POINT('Ctrl Pts',(1.31034972959575,5.04601845063795,33.8851178582125));
#51959=CARTESIAN_POINT('Ctrl Pts',(-0.321949554671762,4.93963032168135,
33.9380381122945));
#51960=CARTESIAN_POINT('Ctrl Pts',(-1.95424883893928,4.83324219272475,33.9909583663764));
#51961=CARTESIAN_POINT('Ctrl Pts',(-3.52859897346783,3.83774776431073,34.0438786204584));
#51962=CARTESIAN_POINT('Ctrl Pts',(-4.32455329212167,2.40870049076816,34.0967988745404));
#51963=CARTESIAN_POINT('Ctrl Pts',(-4.73005222214988,1.68067235297088,34.1237590981413));
#51964=CARTESIAN_POINT('Ctrl Pts',(-4.93352684267558,0.840120210825594,
34.1507193217423));
#51965=CARTESIAN_POINT('Ctrl Pts',(-4.93391474235666,-0.000255694835337854,
34.1776795453433));
#51966=CARTESIAN_POINT('Origin',(0.,0.,16.));
#51967=CARTESIAN_POINT('',(-4.94325592752636,-0.00441992691212867,35.3223204546569));
#51968=CARTESIAN_POINT('',(-4.94405342481732,-0.00430212276008984,35.1776795453432));
#51969=CARTESIAN_POINT('',(-4.942,-6.05220448138622E-16,16.));
#51970=CARTESIAN_POINT('Ctrl Pts',(-4.94325592752636,-0.00441992691212867,
35.3223204546569));
#51971=CARTESIAN_POINT('Ctrl Pts',(-4.93125773853651,1.29607520943411,35.2803989968764));
#51972=CARTESIAN_POINT('Ctrl Pts',(-4.40405811483643,2.60517623543917,35.2384775390958));
#51973=CARTESIAN_POINT('Ctrl Pts',(-3.48340604301779,3.51702727807467,35.1965560813153));
#51974=CARTESIAN_POINT('Ctrl Pts',(-2.32120548652017,4.66811770803537,35.1436358272333));
#51975=CARTESIAN_POINT('Ctrl Pts',(-0.53201099429802,5.18616256481328,35.0907155731514));
#51976=CARTESIAN_POINT('Ctrl Pts',(1.06541470817911,4.83409661000376,35.0377953190694));
#51977=CARTESIAN_POINT('Ctrl Pts',(2.66284041065621,4.48203065519423,34.9848750649874));
#51978=CARTESIAN_POINT('Ctrl Pts',(4.0684973233883,3.25985388879729,34.9319548109055));
#51979=CARTESIAN_POINT('Ctrl Pts',(4.63913537493446,1.72685306505386,34.8790345568235));
#51980=CARTESIAN_POINT('Ctrl Pts',(5.20977342648062,0.193852241310417,34.8261143027416));
#51981=CARTESIAN_POINT('Ctrl Pts',(4.94539261684082,-1.64997263977952,34.7731940486596));
#51982=CARTESIAN_POINT('Ctrl Pts',(3.96697764231472,-2.96085915244703,34.7202737945776));
#51983=CARTESIAN_POINT('Ctrl Pts',(2.98856266778862,-4.27174566511454,34.6673535404957));
#51984=CARTESIAN_POINT('Ctrl Pts',(1.29611352837622,-5.04969380935962,34.6144332864137));
#51985=CARTESIAN_POINT('Ctrl Pts',(-0.335879201461312,-4.93870263300798,
34.5615130323317));
#51986=CARTESIAN_POINT('Ctrl Pts',(-1.96787193129885,-4.82771145665634,
34.5085927782498));
#51987=CARTESIAN_POINT('Ctrl Pts',(-3.53940825156152,-3.82778095970798,
34.4556725241678));
#51988=CARTESIAN_POINT('Ctrl Pts',(-4.33132914049615,-2.39649460920384,
34.4027522700858));
#51989=CARTESIAN_POINT('Ctrl Pts',(-4.73253428635246,-1.67137236904084,
34.3759416649429));
#51990=CARTESIAN_POINT('Ctrl Pts',(-4.93363817440523,-0.835535479848384,
34.3491310597999));
#51991=CARTESIAN_POINT('Ctrl Pts',(-4.93390856647989,0.000179243442527399,
34.3223204546569));
#51992=CARTESIAN_POINT('Ctrl Pts',(-4.93391474235666,-0.000255694835337854,
34.1776795453433));
#51993=CARTESIAN_POINT('Ctrl Pts',(-4.93428825140812,-0.80945462617062,
34.2036395758242));
#51994=CARTESIAN_POINT('Ctrl Pts',(-4.7463640914517,-1.61849015480256,34.2295996063052));
#51995=CARTESIAN_POINT('Ctrl Pts',(-4.36919376142154,-2.32674560401052,
34.2555596367863));
#51996=CARTESIAN_POINT('Ctrl Pts',(-3.60032140928848,-3.77054430657554,
34.3084798908682));
#51997=CARTESIAN_POINT('Ctrl Pts',(-2.04501820224325,-4.79554159303451,
34.3614001449502));
#51998=CARTESIAN_POINT('Ctrl Pts',(-0.415014641507274,-4.93268305062891,
34.4143203990321));
#51999=CARTESIAN_POINT('Ctrl Pts',(1.21498891922872,-5.0698245082233,34.4672406531141));
#52000=CARTESIAN_POINT('Ctrl Pts',(2.91969283365546,-4.31911013695313,34.5201609071961));
#52001=CARTESIAN_POINT('Ctrl Pts',(3.91899855510175,-3.02407829854611,34.573081161278));
#52002=CARTESIAN_POINT('Ctrl Pts',(4.91830427654803,-1.72904646013911,34.62600141536));
#52003=CARTESIAN_POINT('Ctrl Pts',(5.21221180501386,0.110302845404735,34.678921669442));
#52004=CARTESIAN_POINT('Ctrl Pts',(4.66622456671209,1.65225528404048,34.7318419235239));
#52005=CARTESIAN_POINT('Ctrl Pts',(4.12023732841032,3.19420772267622,34.7847621776059));
#52006=CARTESIAN_POINT('Ctrl Pts',(2.73435532334095,4.43876329440389,34.8376824316879));
#52007=CARTESIAN_POINT('Ctrl Pts',(1.14277932318225,4.81639436187842,34.8906026857698));
#52008=CARTESIAN_POINT('Ctrl Pts',(-0.448796676976434,5.19402542935295,
34.9435229398518));
#52009=CARTESIAN_POINT('Ctrl Pts',(-2.24606667222443,4.70473199257438,34.9964431939337));
#52010=CARTESIAN_POINT('Ctrl Pts',(-3.42657246357288,3.57242220104389,35.0493634480157));
#52011=CARTESIAN_POINT('Ctrl Pts',(-4.38069925079363,2.65724913586347,35.0921354804582));
#52012=CARTESIAN_POINT('Ctrl Pts',(-4.93192805452064,1.32202900724285,35.1349075129007));
#52013=CARTESIAN_POINT('Ctrl Pts',(-4.94405342481732,-0.00430212276008983,
35.1776795453432));
#52014=CARTESIAN_POINT('Origin',(0.,0.,16.));
#52015=CARTESIAN_POINT('',(-4.94842418382236,0.0025848059749288,36.3223204546569));
#52016=CARTESIAN_POINT('',(-4.9478484900732,0.00296101277178129,36.1776795453433));
#52017=CARTESIAN_POINT('',(-4.942,-6.05220448138622E-16,16.));
#52018=CARTESIAN_POINT('Ctrl Pts',(-4.94842418382236,0.0025848059749288,
36.3223204546569));
#52019=CARTESIAN_POINT('Ctrl Pts',(-4.94937063025513,0.151489796715591,
36.3175074421168));
#52020=CARTESIAN_POINT('Ctrl Pts',(-4.94323189211144,0.300315679824302,
36.3126944295766));
#52021=CARTESIAN_POINT('Ctrl Pts',(-4.92975351682066,0.448473855033485,
36.3078814170365));
#52022=CARTESIAN_POINT('Ctrl Pts',(-4.78155547265312,2.07750935224505,36.2549611629546));
#52023=CARTESIAN_POINT('Ctrl Pts',(-3.74602889959972,3.62582202129232,36.2020409088726));
#52024=CARTESIAN_POINT('Ctrl Pts',(-2.2970465727752,4.38488033790615,36.1491206547906));
#52025=CARTESIAN_POINT('Ctrl Pts',(-0.848064245950652,5.14393865451998,
36.0962004007087));
#52026=CARTESIAN_POINT('Ctrl Pts',(1.01437383464502,5.11374261870034,36.0432801466267));
#52027=CARTESIAN_POINT('Ctrl Pts',(2.43798755887529,4.30811039761326,35.9903598925447));
#52028=CARTESIAN_POINT('Ctrl Pts',(3.86160128310556,3.50247817652618,35.9374396384628));
#52029=CARTESIAN_POINT('Ctrl Pts',(4.84639065097043,1.92140977017166,35.8845193843808));
#52030=CARTESIAN_POINT('Ctrl Pts',(4.94170100734347,0.28842622847917,35.8315991302989));
#52031=CARTESIAN_POINT('Ctrl Pts',(5.03701136371651,-1.34455731321331,35.7786788762169));
#52032=CARTESIAN_POINT('Ctrl Pts',(4.24284270859772,-3.02945599024377,35.7257586221349));
#52033=CARTESIAN_POINT('Ctrl Pts',(2.92261874766819,-3.99523443505293,35.6728383680529));
#52034=CARTESIAN_POINT('Ctrl Pts',(1.60239478673866,-4.96101287986208,35.619918113971));
#52035=CARTESIAN_POINT('Ctrl Pts',(-0.243884480001596,-5.20767109244996,
35.566997859889));
#52036=CARTESIAN_POINT('Ctrl Pts',(-1.77133346242501,-4.62233450759977,
35.5140776058071));
#52037=CARTESIAN_POINT('Ctrl Pts',(-3.29878244484848,-4.03699792274956,
35.4611573517251));
#52038=CARTESIAN_POINT('Ctrl Pts',(-4.50740114295507,-2.61966654046123,
35.4082370976431));
#52039=CARTESIAN_POINT('Ctrl Pts',(-4.84410718162179,-1.01893284774532,
35.3553168435612));
#52040=CARTESIAN_POINT('Ctrl Pts',(-4.91408721473011,-0.686240873293583,
35.3443180472597));
#52041=CARTESIAN_POINT('Ctrl Pts',(-4.94640385328257,-0.345626598935659,
35.3333192509583));
#52042=CARTESIAN_POINT('Ctrl Pts',(-4.94325592752636,-0.00441992691212867,
35.3223204546569));
#52043=CARTESIAN_POINT('Ctrl Pts',(-4.94405342481732,-0.00430212276008983,
35.1776795453432));
#52044=CARTESIAN_POINT('Ctrl Pts',(-4.94693032680687,-0.318991453753773,
35.1878277669827));
#52045=CARTESIAN_POINT('Ctrl Pts',(-4.91945907962359,-0.633180389759553,
35.1979759886221));
#52046=CARTESIAN_POINT('Ctrl Pts',(-4.85982046564743,-0.941139879242983,
35.2081242102616));
#52047=CARTESIAN_POINT('Ctrl Pts',(-4.54882108892463,-2.5470660217169,35.2610444643436));
#52048=CARTESIAN_POINT('Ctrl Pts',(-3.36308074803015,-3.98359216038229,
35.3139647184255));
#52049=CARTESIAN_POINT('Ctrl Pts',(-1.84521233241245,-4.59334199455474,
35.3668849725075));
#52050=CARTESIAN_POINT('Ctrl Pts',(-0.327343916794751,-5.2030918287272,
35.4198052265894));
#52051=CARTESIAN_POINT('Ctrl Pts',(1.52265257354617,-4.98606535840671,35.4727254806714));
#52052=CARTESIAN_POINT('Ctrl Pts',(2.858190490191,-4.04157721099188,35.5256457347534));
#52053=CARTESIAN_POINT('Ctrl Pts',(4.19372840683581,-3.09708906357705,35.5785659888353));
#52054=CARTESIAN_POINT('Ctrl Pts',(5.01480774978454,-1.42513923906789,35.6314862429173));
#52055=CARTESIAN_POINT('Ctrl Pts',(4.94569007160633,0.20916248765404,35.6844064969993));
#52056=CARTESIAN_POINT('Ctrl Pts',(4.87657239342812,1.843464214376,35.7373267510812));
#52057=CARTESIAN_POINT('Ctrl Pts',(3.91725769412294,3.44011784331073,35.7902470051632));
#52058=CARTESIAN_POINT('Ctrl Pts',(2.50674303141734,4.26847028864764,35.8431672592451));
#52059=CARTESIAN_POINT('Ctrl Pts',(1.09622836871175,5.09682273398456,35.8960875133271));
#52060=CARTESIAN_POINT('Ctrl Pts',(-0.765486257394255,5.15687399572365,
35.9490077674091));
#52061=CARTESIAN_POINT('Ctrl Pts',(-2.2264518005877,4.42114369934827,36.001928021491));
#52062=CARTESIAN_POINT('Ctrl Pts',(-3.68741734378115,3.68541340297289,36.054848275573));
#52063=CARTESIAN_POINT('Ctrl Pts',(-4.74763380406204,2.15390154848305,36.107768529655));
#52064=CARTESIAN_POINT('Ctrl Pts',(-4.92192993683911,0.527451350812649,
36.1606887837369));
#52065=CARTESIAN_POINT('Ctrl Pts',(-4.94058331188609,0.353386757129483,
36.166352370939));
#52066=CARTESIAN_POINT('Ctrl Pts',(-4.94908977224877,0.178234784323597,
36.1720159581411));
#52067=CARTESIAN_POINT('Ctrl Pts',(-4.9478484900732,0.00296101277178129,
36.1776795453433));
#52068=CARTESIAN_POINT('Origin',(0.,0.,16.));
#52069=CARTESIAN_POINT('',(-4.93549302535697,0.00277814199197368,37.3223204546569));
#52070=CARTESIAN_POINT('',(-4.9350718820976,0.00242042316235142,37.1776795453432));
#52071=CARTESIAN_POINT('',(-4.942,-6.05220448138622E-16,16.));
#52072=CARTESIAN_POINT('Ctrl Pts',(-4.93549302535697,0.00277814199197368,
37.3223204546569));
#52073=CARTESIAN_POINT('Ctrl Pts',(-4.93877741300468,0.645159704289348,
37.3016956332752));
#52074=CARTESIAN_POINT('Ctrl Pts',(-4.82236482292357,1.2863972760676,37.2810708118936));
#52075=CARTESIAN_POINT('Ctrl Pts',(-4.5807162353096,1.87633613908203,37.2604459905119));
#52076=CARTESIAN_POINT('Ctrl Pts',(-3.96068154902433,3.39003237653315,37.2075257364299));
#52077=CARTESIAN_POINT('Ctrl Pts',(-2.51614312549289,4.56599842518147,37.1546054823479));
#52078=CARTESIAN_POINT('Ctrl Pts',(-0.908143809323614,4.86609426099016,
37.101685228266));
#52079=CARTESIAN_POINT('Ctrl Pts',(0.699855506845637,5.16619009679885,37.048764974184));
#52080=CARTESIAN_POINT('Ctrl Pts',(2.47131571565271,4.59041571976794,36.995844720102));
#52081=CARTESIAN_POINT('Ctrl Pts',(3.59558957056917,3.40225427845545,36.9429244660201));
#52082=CARTESIAN_POINT('Ctrl Pts',(4.71986342548563,2.21409283714297,36.8900042119381));
#52083=CARTESIAN_POINT('Ctrl Pts',(5.19695092651147,0.413544331548897,36.8370839578562));
#52084=CARTESIAN_POINT('Ctrl Pts',(4.80852954676355,-1.17543274293179,36.7841637037742));
#52085=CARTESIAN_POINT('Ctrl Pts',(4.42010816701563,-2.76440981741246,36.7312434496922));
#52086=CARTESIAN_POINT('Ctrl Pts',(3.16617790649396,-4.14181546077975,36.6783231956103));
#52087=CARTESIAN_POINT('Ctrl Pts',(1.6205564033125,-4.67732781392721,36.6254029415283));
#52088=CARTESIAN_POINT('Ctrl Pts',(0.0749349001310295,-5.21284016707467,
36.5724826874463));
#52089=CARTESIAN_POINT('Ctrl Pts',(-1.76237784571023,-4.90645923000227,
36.5195624333644));
#52090=CARTESIAN_POINT('Ctrl Pts',(-3.05059946099004,-3.89838959877812,
36.4666421792824));
#52091=CARTESIAN_POINT('Ctrl Pts',(-4.22165937898849,-2.98200228957926,
36.4185349377406));
#52092=CARTESIAN_POINT('Ctrl Pts',(-4.93896421945116,-1.48575712054711,
36.3704276961987));
#52093=CARTESIAN_POINT('Ctrl Pts',(-4.94842418382236,0.0025848059749288,
36.3223204546569));
#52094=CARTESIAN_POINT('Ctrl Pts',(-4.9478484900732,0.00296101277178129,
36.1776795453433));
#52095=CARTESIAN_POINT('Ctrl Pts',(-4.93749129838862,-1.4595139062905,36.2249362122231));
#52096=CARTESIAN_POINT('Ctrl Pts',(-4.24848225306339,-2.93046862920176,
36.2721928791029));
#52097=CARTESIAN_POINT('Ctrl Pts',(-3.11270745258791,-3.84898058519796,
36.3194495459828));
#52098=CARTESIAN_POINT('Ctrl Pts',(-1.84081303028634,-4.87757378268728,
36.3723698000648));
#52099=CARTESIAN_POINT('Ctrl Pts',(-0.00864838040995825,-5.21337163681495,
36.4252900541467));
#52100=CARTESIAN_POINT('Ctrl Pts',(1.54535997115889,-4.70270792099264,36.4782103082287));
#52101=CARTESIAN_POINT('Ctrl Pts',(3.09936832272773,-4.19204420517033,36.5311305623107));
#52102=CARTESIAN_POINT('Ctrl Pts',(4.37522037598902,-2.83491891939801,36.5840508163926));
#52103=CARTESIAN_POINT('Ctrl Pts',(4.78906674566614,-1.25237332141095,36.6369710704746));
#52104=CARTESIAN_POINT('Ctrl Pts',(5.20291311534324,0.330172276576089,36.6898913245566));
#52105=CARTESIAN_POINT('Ctrl Pts',(4.75475380143625,2.13813818677785,36.7428115786385));
#52106=CARTESIAN_POINT('Ctrl Pts',(3.64967335059123,3.34417159616718,36.7957318327205));
#52107=CARTESIAN_POINT('Ctrl Pts',(2.54459289974621,4.55020500555648,36.8486520868024));
#52108=CARTESIAN_POINT('Ctrl Pts',(0.782591311963154,5.15430591413334,36.9015723408844));
#52109=CARTESIAN_POINT('Ctrl Pts',(-0.830012575668756,4.88002851988171,
36.9544925949664));
#52110=CARTESIAN_POINT('Ctrl Pts',(-2.44261646330071,4.60575112563006,37.0074128490484));
#52111=CARTESIAN_POINT('Ctrl Pts',(-3.9058226507815,3.45309542854993,37.0603331031303));
#52112=CARTESIAN_POINT('Ctrl Pts',(-4.5500456396125,1.94953427978849,37.1132533572123));
#52113=CARTESIAN_POINT('Ctrl Pts',(-4.81147567364344,1.33937902438292,37.1347287532559));
#52114=CARTESIAN_POINT('Ctrl Pts',(-4.93803628002896,0.671436970049187,
37.1562041492996));
#52115=CARTESIAN_POINT('Ctrl Pts',(-4.9350718820976,0.00242042316235142,
37.1776795453432));
#52116=CARTESIAN_POINT('Origin',(0.,0.,16.));
#52117=CARTESIAN_POINT('',(-4.93830712716952,-0.00410043205665789,38.3223204546569));
#52118=CARTESIAN_POINT('',(-4.93901314208066,-0.00426717980477184,38.1776795453432));
#52119=CARTESIAN_POINT('',(-4.942,-6.05220448138622E-16,16.));
#52120=CARTESIAN_POINT('Ctrl Pts',(-4.93830712716952,-0.00410043205665789,
38.3223204546569));
#52121=CARTESIAN_POINT('Ctrl Pts',(-4.92941979674321,1.12913042651997,38.2858838244337));
#52122=CARTESIAN_POINT('Ctrl Pts',(-4.54190399082784,2.26785272885638,38.2494471942104));
#52123=CARTESIAN_POINT('Ctrl Pts',(-3.8277718834972,3.13875149433059,38.2130105639872));
#52124=CARTESIAN_POINT('Ctrl Pts',(-2.79057244061549,4.40363750783395,38.1600903099052));
#52125=CARTESIAN_POINT('Ctrl Pts',(-1.06439510407127,5.10356550944081,38.1071700558233));
#52126=CARTESIAN_POINT('Ctrl Pts',(0.560835013546147,4.91823775582626,38.0542498017413));
#52127=CARTESIAN_POINT('Ctrl Pts',(2.18606513116352,4.73291000221171,38.0013295476593));
#52128=CARTESIAN_POINT('Ctrl Pts',(3.71034802985413,3.66232649337579,37.9484092935774));
#52129=CARTESIAN_POINT('Ctrl Pts',(4.43614857526344,2.19640259366137,37.8954890394954));
#52130=CARTESIAN_POINT('Ctrl Pts',(5.16194912067276,0.730478693946923,37.8425687854135));
#52131=CARTESIAN_POINT('Ctrl Pts',(5.08926731280079,-1.13078559664599,37.7896485313315));
#52132=CARTESIAN_POINT('Ctrl Pts',(4.25136345697712,-2.53564731221314,37.7367282772495));
#52133=CARTESIAN_POINT('Ctrl Pts',(3.41345960115345,-3.94050902778028,37.6838080231676));
#52134=CARTESIAN_POINT('Ctrl Pts',(1.81033369737808,-4.88896816832161,37.6308877690856));
#52135=CARTESIAN_POINT('Ctrl Pts',(0.175600643277768,-4.9469953455946,37.5779675150036));
#52136=CARTESIAN_POINT('Ctrl Pts',(-1.45913241082256,-5.00502252286759,
37.5250472609217));
#52137=CARTESIAN_POINT('Ctrl Pts',(-3.12547261524786,-4.17261773687219,
37.4721270068397));
#52138=CARTESIAN_POINT('Ctrl Pts',(-4.06087724294093,-2.83070213074755,
37.4192067527577));
#52139=CARTESIAN_POINT('Ctrl Pts',(-4.63172289977408,-2.01177663806308,
37.3869113200575));
#52140=CARTESIAN_POINT('Ctrl Pts',(-4.93035015801884,-1.00309677586341,
37.3546158873572));
#52141=CARTESIAN_POINT('Ctrl Pts',(-4.93549302535697,0.00277814199197368,
37.3223204546569));
#52142=CARTESIAN_POINT('Ctrl Pts',(-4.9350718820976,0.00242042316235142,
37.1776795453432));
#52143=CARTESIAN_POINT('Ctrl Pts',(-4.93073133015009,-0.977171771522589,
37.2091244033815));
#52144=CARTESIAN_POINT('Ctrl Pts',(-4.64869419974499,-1.95906763650772,
37.2405692614198));
#52145=CARTESIAN_POINT('Ctrl Pts',(-4.10573795122914,-2.76523328246712,
37.2720141194581));
#52146=CARTESIAN_POINT('Ctrl Pts',(-3.19196748383364,-4.12197309551857,
37.3249343735401));
#52147=CARTESIAN_POINT('Ctrl Pts',(-1.53918675886144,-4.9809861211788,37.3778546276221));
#52148=CARTESIAN_POINT('Ctrl Pts',(0.0962665215178138,-4.94917487945839,
37.4307748817041));
#52149=CARTESIAN_POINT('Ctrl Pts',(1.73171980189707,-4.91736363773799,37.483695135786));
#52150=CARTESIAN_POINT('Ctrl Pts',(3.34984563768341,-3.99472812863699,37.536615389868));
#52151=CARTESIAN_POINT('Ctrl Pts',(4.21016493327244,-2.60348045225429,37.5895356439499));
#52152=CARTESIAN_POINT('Ctrl Pts',(5.07048422886148,-1.21223277587156,37.6424558980319));
#52153=CARTESIAN_POINT('Ctrl Pts',(5.17299698425316,0.64762706779285,37.6953761521139));
#52154=CARTESIAN_POINT('Ctrl Pts',(4.47079179693381,2.12499880919883,37.7482964061958));
#52155=CARTESIAN_POINT('Ctrl Pts',(3.76858660961448,3.60237055060479,37.8012166602778));
#52156=CARTESIAN_POINT('Ctrl Pts',(2.26166347958414,4.69725418975229,37.8541369143597));
#52157=CARTESIAN_POINT('Ctrl Pts',(0.639613445927835,4.90861425153937,37.9070571684417));
#52158=CARTESIAN_POINT('Ctrl Pts',(-0.982436587728495,5.11997431332645,
37.9599774225237));
#52159=CARTESIAN_POINT('Ctrl Pts',(-2.71961352501084,4.44781079775303,38.0128976766056));
#52160=CARTESIAN_POINT('Ctrl Pts',(-3.77695866803847,3.19971599529649,38.0658179306876));
#52161=CARTESIAN_POINT('Ctrl Pts',(-4.52195594113156,2.32031797609409,38.1031051355728));
#52162=CARTESIAN_POINT('Ctrl Pts',(-4.92945048540112,1.15499867080211,38.140392340458));
#52163=CARTESIAN_POINT('Ctrl Pts',(-4.93901314208066,-0.00426717980477184,
38.1776795453432));
#52164=CARTESIAN_POINT('Origin',(0.,0.,16.));
#52165=CARTESIAN_POINT('',(-4.95007301157197,-0.000387401246429997,39.3223204546569));
#52166=CARTESIAN_POINT('',(-4.95010830192917,0.000103228088722096,39.1776795453432));
#52167=CARTESIAN_POINT('',(-4.942,-6.05220448138622E-16,16.));
#52168=CARTESIAN_POINT('Ctrl Pts',(-4.95007301157197,-0.000387401246429997,
39.3223204546569));
#52169=CARTESIAN_POINT('Ctrl Pts',(-4.94825412650634,1.61464285750734,39.2700720155921));
#52170=CARTESIAN_POINT('Ctrl Pts',(-4.08291838964434,3.23134503628798,39.2178235765273));
#52171=CARTESIAN_POINT('Ctrl Pts',(-2.73731172677047,4.12440578092639,39.1655751374625));
#52172=CARTESIAN_POINT('Ctrl Pts',(-1.37440313527419,5.0289495790347,39.1126548833806));
#52173=CARTESIAN_POINT('Ctrl Pts',(0.481206517102607,5.19112301285789,39.0597346292986));
#52174=CARTESIAN_POINT('Ctrl Pts',(1.98036191326499,4.53671304225247,39.0068143752166));
#52175=CARTESIAN_POINT('Ctrl Pts',(3.47951730942733,3.88230307164706,38.9538941211347));
#52176=CARTESIAN_POINT('Ctrl Pts',(4.62221844937522,2.41130969661302,38.9009738670527));
#52177=CARTESIAN_POINT('Ctrl Pts',(4.88554783933805,0.796881951604831,38.8480536129708));
#52178=CARTESIAN_POINT('Ctrl Pts',(5.14887722930088,-0.817545793403355,
38.7951333588888));
#52179=CARTESIAN_POINT('Ctrl Pts',(4.53283486927871,-2.57540790838573,38.7422131048068));
#52180=CARTESIAN_POINT('Ctrl Pts',(3.31933115184711,-3.67227984222765,38.6892928507249));
#52181=CARTESIAN_POINT('Ctrl Pts',(2.10582743441549,-4.76915177606959,38.6363725966429));
#52182=CARTESIAN_POINT('Ctrl Pts',(0.294862359574459,-5.20503352877106,
38.5834523425609));
#52183=CARTESIAN_POINT('Ctrl Pts',(-1.28483879610452,-4.78045895320511,
38.530532088479));
#52184=CARTESIAN_POINT('Ctrl Pts',(-2.86453995178352,-4.35588437763916,
38.477611834397));
#52185=CARTESIAN_POINT('Ctrl Pts',(-4.21297718830044,-3.07085347380577,
38.424691580315));
#52186=CARTESIAN_POINT('Ctrl Pts',(-4.71308503194927,-1.51341600918913,
38.3717713262331));
#52187=CARTESIAN_POINT('Ctrl Pts',(-4.86885884155228,-1.02830470737132,
38.3552877023743));
#52188=CARTESIAN_POINT('Ctrl Pts',(-4.94232768041382,-0.516764503992941,
38.3388040785156));
#52189=CARTESIAN_POINT('Ctrl Pts',(-4.93830712716952,-0.00410043205665789,
38.3223204546569));
#52190=CARTESIAN_POINT('Ctrl Pts',(-4.93901314208066,-0.00426717980477184,
38.1776795453432));
#52191=CARTESIAN_POINT('Ctrl Pts',(-4.94302238554053,-0.490301467717737,
38.19331259454));
#52192=CARTESIAN_POINT('Ctrl Pts',(-4.87708344029753,-0.975271683602742,
38.2089456437367));
#52193=CARTESIAN_POINT('Ctrl Pts',(-4.7367428403112,-1.43766007643938,38.2245786929335));
#52194=CARTESIAN_POINT('Ctrl Pts',(-4.26166852078334,-3.00291525637914,
38.2774989470154));
#52195=CARTESIAN_POINT('Ctrl Pts',(-2.9340065329546,-4.30939952691902,38.3304192010974));
#52196=CARTESIAN_POINT('Ctrl Pts',(-1.36131527943717,-4.75924573231914,
38.3833394551794));
#52197=CARTESIAN_POINT('Ctrl Pts',(0.211375974080253,-5.20909193771926,
38.4362597092614));
#52198=CARTESIAN_POINT('Ctrl Pts',(2.0290964932864,-4.80230007797962,38.4891799633433));
#52199=CARTESIAN_POINT('Ctrl Pts',(3.2600296070944,-3.72502432092665,38.5421002174252));
#52200=CARTESIAN_POINT('Ctrl Pts',(4.4909627209024,-2.64774856387368,38.5950204715072));
#52201=CARTESIAN_POINT('Ctrl Pts',(5.13510842931226,-0.899988909507443,
38.6479407255892));
#52202=CARTESIAN_POINT('Ctrl Pts',(4.89769581831224,0.718453131327276,38.7008609796712));
#52203=CARTESIAN_POINT('Ctrl Pts',(4.66028320731222,2.33689517216197,38.7537812337531));
#52204=CARTESIAN_POINT('Ctrl Pts',(3.54131227690224,3.82601959946517,38.8067014878351));
#52205=CARTESIAN_POINT('Ctrl Pts',(2.05284121454405,4.50438033235388,38.859621741917));
#52206=CARTESIAN_POINT('Ctrl Pts',(0.564370152185806,5.18274106524261,38.912541995999));
#52207=CARTESIAN_POINT('Ctrl Pts',(-1.29360104212064,5.05033810371689,38.965462250081));
#52208=CARTESIAN_POINT('Ctrl Pts',(-2.67083637362622,4.16776106512145,39.0183825041629));
#52209=CARTESIAN_POINT('Ctrl Pts',(-4.04807170513178,3.28518402652602,39.0713027582449));
#52210=CARTESIAN_POINT('Ctrl Pts',(-4.94457117383642,1.65243291086087,39.1242230123269));
#52211=CARTESIAN_POINT('Ctrl Pts',(-4.95008293089447,0.0166795651704946,
39.1771432664088));
#52212=CARTESIAN_POINT('Ctrl Pts',(-4.95010154909182,0.0111541440981086,
39.1773220260536));
#52213=CARTESIAN_POINT('Ctrl Pts',(-4.95011000089745,0.00562868876953041,
39.1775007856984));
#52214=CARTESIAN_POINT('Ctrl Pts',(-4.95010830192917,0.000103228088722096,
39.1776795453432));
#52215=CARTESIAN_POINT('Origin',(0.,0.,16.));
#52216=CARTESIAN_POINT('',(-4.93943724668283,0.00434520414469897,40.3223204546569));
#52217=CARTESIAN_POINT('',(-4.9387122051873,0.0042019715207839,40.1776795453432));
#52218=CARTESIAN_POINT('',(-4.942,-6.05220448138622E-16,16.));
#52219=CARTESIAN_POINT('Ctrl Pts',(-4.93943724668283,0.00434520414469897,
40.3223204546569));
#52220=CARTESIAN_POINT('Ctrl Pts',(-4.94341650816428,0.474947915493244,
40.3071804608325));
#52221=CARTESIAN_POINT('Ctrl Pts',(-4.88164614501736,0.944527111103383,
40.2920404670082));
#52222=CARTESIAN_POINT('Ctrl Pts',(-4.74989944410437,1.39357590613184,40.2769004731838));
#52223=CARTESIAN_POINT('Ctrl Pts',(-4.28939272477215,2.96317868165193,40.2239802191018));
#52224=CARTESIAN_POINT('Ctrl Pts',(-2.97393022079225,4.28194545604953,40.1710599650198));
#52225=CARTESIAN_POINT('Ctrl Pts',(-1.40548766464857,4.74638841223249,40.1181397109379));
#52226=CARTESIAN_POINT('Ctrl Pts',(0.162954891495088,5.21083136841545,40.0652194568559));
#52227=CARTESIAN_POINT('Ctrl Pts',(1.98437749980252,4.82095050638379,40.012299202774));
#52228=CARTESIAN_POINT('Ctrl Pts',(3.22526935667327,3.75516126313619,39.959378948692));
#52229=CARTESIAN_POINT('Ctrl Pts',(4.46616121354403,2.68937201988858,39.90645869461));
#52230=CARTESIAN_POINT('Ctrl Pts',(5.1265223189781,0.947674395425016,39.8535384405281));
#52231=CARTESIAN_POINT('Ctrl Pts',(4.90416134563252,-0.672904176876648,
39.8006181864461));
#52232=CARTESIAN_POINT('Ctrl Pts',(4.68180037228695,-2.29348274917834,39.7476979323641));
#52233=CARTESIAN_POINT('Ctrl Pts',(3.57671732016171,-3.79294226931812,39.6947776782822));
#52234=CARTESIAN_POINT('Ctrl Pts',(2.09461507151,-4.4851071600863,39.6418574242002));
#52235=CARTESIAN_POINT('Ctrl Pts',(0.612512822858338,-5.17727205085446,
39.5889371701182));
#52236=CARTESIAN_POINT('Ctrl Pts',(-1.24660862231976,-5.06214231225107,
39.5360169160363));
#52237=CARTESIAN_POINT('Ctrl Pts',(-2.63198689690885,-4.19240307100288,
39.4830966619543));
#52238=CARTESIAN_POINT('Ctrl Pts',(-4.01736517149795,-3.32266382975467,
39.4301764078723));
#52239=CARTESIAN_POINT('Ctrl Pts',(-4.92900027549801,-1.69831508586162,
39.3772561537904));
#52240=CARTESIAN_POINT('Ctrl Pts',(-4.9497140621902,-0.0626836327184169,
39.3243358997084));
#52241=CARTESIAN_POINT('Ctrl Pts',(-4.94997702073422,-0.0419195265770804,
39.3236640846913));
#52242=CARTESIAN_POINT('Ctrl Pts',(-4.95009639895585,-0.0211536021213772,
39.3229922696741));
#52243=CARTESIAN_POINT('Ctrl Pts',(-4.95007301157197,-0.000387401246429997,
39.3223204546569));
#52244=CARTESIAN_POINT('Ctrl Pts',(-4.95010830192917,0.000103228088722096,
39.1776795453432));
#52245=CARTESIAN_POINT('Ctrl Pts',(-4.94960703596349,-1.6301363826534,39.2304210397804));
#52246=CARTESIAN_POINT('Ctrl Pts',(-4.06548675829959,-3.26084190194751,
39.2831625342175));
#52247=CARTESIAN_POINT('Ctrl Pts',(-2.6988623875562,-4.14966758230844,39.3359040286547));
#52248=CARTESIAN_POINT('Ctrl Pts',(-1.32760604174843,-5.04150580838138,
39.3888242827367));
#52249=CARTESIAN_POINT('Ctrl Pts',(0.529430695278565,-5.18642668481171,
39.4417445368187));
#52250=CARTESIAN_POINT('Ctrl Pts',(2.02243945069843,-4.51811220521201,39.4946647909006));
#52251=CARTESIAN_POINT('Ctrl Pts',(3.51544820611836,-3.84979772561229,39.5475850449826));
#52252=CARTESIAN_POINT('Ctrl Pts',(4.6444289799311,-2.36824788998248,39.6005052990645));
#52253=CARTESIAN_POINT('Ctrl Pts',(4.89274292745657,-0.751442530371268,
39.6534255531465));
#52254=CARTESIAN_POINT('Ctrl Pts',(5.14105687498204,0.865362829239897,39.7063458072285));
#52255=CARTESIAN_POINT('Ctrl Pts',(4.50870399622024,2.61742371283248,39.7592660613104));
#52256=CARTESIAN_POINT('Ctrl Pts',(3.2850586262277,3.70297030137619,39.8121863153924));
#52257=CARTESIAN_POINT('Ctrl Pts',(2.06141325623513,4.78851688991993,39.8651065694743));
#52258=CARTESIAN_POINT('Ctrl Pts',(0.246475395011777,5.2075491834148,39.9180268235563));
#52259=CARTESIAN_POINT('Ctrl Pts',(-1.32921167314713,4.76831160460351,39.9709470776383));
#52260=CARTESIAN_POINT('Ctrl Pts',(-2.90489874130597,4.32907402579225,40.0238673317202));
#52261=CARTESIAN_POINT('Ctrl Pts',(-4.24133501640037,3.03156657467491,40.0767875858022));
#52262=CARTESIAN_POINT('Ctrl Pts',(-4.72694684795839,1.46954847732333,40.1297078398842));
#52263=CARTESIAN_POINT('Ctrl Pts',(-4.87368101212714,0.997563642860038,
40.1456984083705));
#52264=CARTESIAN_POINT('Ctrl Pts',(-4.94273254556439,0.501428253000672,
40.1616889768569));
#52265=CARTESIAN_POINT('Ctrl Pts',(-4.9387122051873,0.0042019715207839,
40.1776795453432));
#52266=CARTESIAN_POINT('Origin',(0.,0.,16.));
#52267=CARTESIAN_POINT('',(-4.93485552516168,-0.00220275864159403,41.3223204546569));
#52268=CARTESIAN_POINT('',(-4.93524162710697,-0.00257366327817901,41.1776795453432));
#52269=CARTESIAN_POINT('',(-4.942,-6.05220448138622E-16,16.));
#52270=CARTESIAN_POINT('Ctrl Pts',(-4.93485552516168,-0.00220275864159403,
41.3223204546569));
#52271=CARTESIAN_POINT('Ctrl Pts',(-4.93097721826847,0.962135133190097,
41.291368651991));
#52272=CARTESIAN_POINT('Ctrl Pts',(-4.65830472720369,1.92849849558568,41.2604168493251));
#52273=CARTESIAN_POINT('Ctrl Pts',(-4.13125993704044,2.72695615437044,41.2294650466591));
#52274=CARTESIAN_POINT('Ctrl Pts',(-3.23013813457067,4.09212969959618,41.1765447925771));
#52275=CARTESIAN_POINT('Ctrl Pts',(-1.58541225739997,4.96646613003761,41.1236245384952));
#52276=CARTESIAN_POINT('Ctrl Pts',(0.0502660136753988,4.94985574164777,
41.0707042844132));
#52277=CARTESIAN_POINT('Ctrl Pts',(1.68594428475072,4.93324535325794,41.0177840303312));
#52278=CARTESIAN_POINT('Ctrl Pts',(3.31257494973071,4.0256881460368,40.9648637762493));
#52279=CARTESIAN_POINT('Ctrl Pts',(4.18578697328013,2.64249615885673,40.9119435221673));
#52280=CARTESIAN_POINT('Ctrl Pts',(5.05899899682956,1.25930417167664,40.8590232680854));
#52281=CARTESIAN_POINT('Ctrl Pts',(5.17879237894847,-0.599522595462416,
40.8061030140034));
#52282=CARTESIAN_POINT('Ctrl Pts',(4.49034783841098,-2.08335662461616,40.7531827599214));
#52283=CARTESIAN_POINT('Ctrl Pts',(3.8019032978735,-3.56719065376989,40.7002625058395));
#52284=CARTESIAN_POINT('Ctrl Pts',(2.30522083467963,-4.67603194493831,40.6473422517575));
#52285=CARTESIAN_POINT('Ctrl Pts',(0.685205202367444,-4.90245778828362,
40.5944219976755));
#52286=CARTESIAN_POINT('Ctrl Pts',(-0.93481042994472,-5.12888363162893,
40.5415017435936));
#52287=CARTESIAN_POINT('Ctrl Pts',(-2.6781592313752,-4.47289402715115,40.4885814895116));
#52288=CARTESIAN_POINT('Ctrl Pts',(-3.74705816474816,-3.23467983659099,
40.4356612354296));
#52289=CARTESIAN_POINT('Ctrl Pts',(-4.51015502798955,-2.35070724073872,
40.397880975172));
#52290=CARTESIAN_POINT('Ctrl Pts',(-4.92950741869571,-1.16999430476845,
40.3601007149145));
#52291=CARTESIAN_POINT('Ctrl Pts',(-4.93943724668283,0.00434520414469897,
40.3223204546569));
#52292=CARTESIAN_POINT('Ctrl Pts',(-4.9387122051873,0.0042019715207839,
40.1776795453432));
#52293=CARTESIAN_POINT('Ctrl Pts',(-4.92942736292292,-1.14412557296836,
40.2146092309388));
#52294=CARTESIAN_POINT('Ctrl Pts',(-4.53040370843391,-2.2982715368062,40.2515389165345));
#52295=CARTESIAN_POINT('Ctrl Pts',(-3.79843588104676,-3.17419030434592,
40.2884686021301));
#52296=CARTESIAN_POINT('Ctrl Pts',(-2.74952569455548,-4.42938224507769,
40.341388856212));
#52297=CARTESIAN_POINT('Ctrl Pts',(-1.01691793355136,-5.11323738295533,
40.394309110294));
#52298=CARTESIAN_POINT('Ctrl Pts',(0.606519628933596,-4.91281316257247,
40.4472293643759));
#52299=CARTESIAN_POINT('Ctrl Pts',(2.22995719141853,-4.71238894218962,40.5001496184579));
#52300=CARTESIAN_POINT('Ctrl Pts',(3.74422455538428,-3.62768536354625,40.5530698725399));
#52301=CARTESIAN_POINT('Ctrl Pts',(4.45636984813063,-2.15507935058069,40.6059901266218));
#52302=CARTESIAN_POINT('Ctrl Pts',(5.16851514087698,-0.682473337615157,
40.6589103807038));
#52303=CARTESIAN_POINT('Ctrl Pts',(5.07853836240398,1.17803510967258,40.7118306347858));
#52304=CARTESIAN_POINT('Ctrl Pts',(4.22761426072911,2.57504891081838,40.7647508888677));
#52305=CARTESIAN_POINT('Ctrl Pts',(3.37669015905424,3.97206271196421,40.8176711429497));
#52306=CARTESIAN_POINT('Ctrl Pts',(1.76481873417747,4.90558186696812,40.8705913970317));
#52307=CARTESIAN_POINT('Ctrl Pts',(0.12961696774931,4.94841375314338,40.9235116511136));
#52308=CARTESIAN_POINT('Ctrl Pts',(-1.50558479867887,4.99124563931864,40.9764319051956));
#52309=CARTESIAN_POINT('Ctrl Pts',(-3.16411690665841,4.14339025666527,41.0293521592775));
#52310=CARTESIAN_POINT('Ctrl Pts',(-4.0870097333165,2.79283917732535,41.0822724133595));
#52311=CARTESIAN_POINT('Ctrl Pts',(-4.6416213166461,1.98122676595515,41.1140747906874));
#52312=CARTESIAN_POINT('Ctrl Pts',(-4.93056429073029,0.988070940573039,
41.1458771680153));
#52313=CARTESIAN_POINT('Ctrl Pts',(-4.93524162710697,-0.00257366327817901,
41.1776795453432));
#52314=CARTESIAN_POINT('Origin',(0.,0.,16.));
#52315=CARTESIAN_POINT('',(-4.94748713622925,-0.00316321289392352,42.3223204546569));
#52316=CARTESIAN_POINT('',(-4.94809820533655,-0.00280696805152256,42.1776795453432));
#52317=CARTESIAN_POINT('',(-4.942,-6.05220448138622E-16,16.));
#52318=CARTESIAN_POINT('Ctrl Pts',(-4.94748713622925,-0.00316321289392352,
42.3223204546569));
#52319=CARTESIAN_POINT('Ctrl Pts',(-4.93670139323051,1.44433029491444,42.2755568431494));
#52320=CARTESIAN_POINT('Ctrl Pts',(-4.26377312667576,2.9005508041267,42.2287932316419));
#52321=CARTESIAN_POINT('Ctrl Pts',(-3.14834440585587,3.81988560527279,42.1820296201344));
#52322=CARTESIAN_POINT('Ctrl Pts',(-1.88606441050834,4.8602550227471,42.1291093660525));
#52323=CARTESIAN_POINT('Ctrl Pts',(-0.0570997319322858,5.21306603328002,
42.0761891119705));
#52324=CARTESIAN_POINT('Ctrl Pts',(1.50158745972911,4.71686693007535,42.0232688578886));
#52325=CARTESIAN_POINT('Ctrl Pts',(3.06027465139055,4.22066782687068,41.9703486038066));
#52326=CARTESIAN_POINT('Ctrl Pts',(4.34868435613734,2.87545860992836,41.9174283497246));
#52327=CARTESIAN_POINT('Ctrl Pts',(4.77722061558389,1.29682756189652,41.8645080956427));
#52328=CARTESIAN_POINT('Ctrl Pts',(5.20575687503042,-0.281803486135251,
41.8115878415607));
#52329=CARTESIAN_POINT('Ctrl Pts',(4.77441968917683,-2.09385636525649,41.7586675874787));
#52330=CARTESIAN_POINT('Ctrl Pts',(3.68059554195264,-3.31010800304349,41.7057473333968));
#52331=CARTESIAN_POINT('Ctrl Pts',(2.58677139472839,-4.52635964083055,41.6528270793148));
#52332=CARTESIAN_POINT('Ctrl Pts',(0.830460286133465,-5.14681003728328,
41.5999068252328));
#52333=CARTESIAN_POINT('Ctrl Pts',(-0.78462299692839,-4.88753161503282,
41.5469865711509));
#52334=CARTESIAN_POINT('Ctrl Pts',(-2.39970627999022,-4.62825319278237,
41.4940663170689));
#52335=CARTESIAN_POINT('Ctrl Pts',(-3.87356173751901,-3.48924595182876,
41.4411460629869));
#52336=CARTESIAN_POINT('Ctrl Pts',(-4.531730602399,-1.99173700134697,41.388225808905));
#52337=CARTESIAN_POINT('Ctrl Pts',(-4.80495209353668,-1.37008555249385,
41.366257357489));
#52338=CARTESIAN_POINT('Ctrl Pts',(-4.93760820478682,-0.686654334984092,
41.3442889060729));
#52339=CARTESIAN_POINT('Ctrl Pts',(-4.93485552516168,-0.00220275864159403,
41.3223204546569));
#52340=CARTESIAN_POINT('Ctrl Pts',(-4.93524162710697,-0.00257366327817901,
41.1776795453432));
#52341=CARTESIAN_POINT('Ctrl Pts',(-4.93834753998013,-0.660395889443513,
41.1987974220973));
#52342=CARTESIAN_POINT('Ctrl Pts',(-4.81610883381463,-1.31711081291602,
41.2199152988513));
#52343=CARTESIAN_POINT('Ctrl Pts',(-4.56308028711322,-1.91882712196431,
41.2410331756054));
#52344=CARTESIAN_POINT('Ctrl Pts',(-3.92900446891528,-3.42669556588764,
41.2939534296874));
#52345=CARTESIAN_POINT('Ctrl Pts',(-2.47359928718284,-4.58918567770784,
41.3468736837693));
#52346=CARTESIAN_POINT('Ctrl Pts',(-0.862880381041693,-4.87432422789462,
41.3997939378513));
#52347=CARTESIAN_POINT('Ctrl Pts',(0.74783852509941,-5.15946277808138,41.4527141919333));
#52348=CARTESIAN_POINT('Ctrl Pts',(2.51387115564923,-4.56724976663472,41.5056344460152));
#52349=CARTESIAN_POINT('Ctrl Pts',(3.62705400678358,-3.36869091228363,41.5585547000972));
#52350=CARTESIAN_POINT('Ctrl Pts',(4.74023685791794,-2.17013205793252,41.6114749541791));
#52351=CARTESIAN_POINT('Ctrl Pts',(5.20056992963686,-0.36522736067698,41.6643952082611));
#52352=CARTESIAN_POINT('Ctrl Pts',(4.79739777779339,1.22007122425299,41.7173154623431));
#52353=CARTESIAN_POINT('Ctrl Pts',(4.3942256259499,2.80536980918301,41.770235716425));
#52354=CARTESIAN_POINT('Ctrl Pts',(3.12754825054399,4.17106228178741,41.823155970507));
#52355=CARTESIAN_POINT('Ctrl Pts',(1.57701656414349,4.69218690879255,41.8760762245889));
#52356=CARTESIAN_POINT('Ctrl Pts',(0.0264848777430365,5.21331153579767,
41.9289964786709));
#52357=CARTESIAN_POINT('Ctrl Pts',(-1.80790111965202,4.88986831720356,41.9819167327529));
#52358=CARTESIAN_POINT('Ctrl Pts',(-3.08669837960869,3.86986980968975,42.0348369868349));
#52359=CARTESIAN_POINT('Ctrl Pts',(-4.2372765819408,2.95214181174547,42.0824511730043));
#52360=CARTESIAN_POINT('Ctrl Pts',(-4.93809323584742,1.47053667915491,42.1300653591738));
#52361=CARTESIAN_POINT('Ctrl Pts',(-4.94809820533655,-0.00280696805152256,
42.1776795453432));
#52362=CARTESIAN_POINT('Origin',(0.,0.,16.));
#52363=CARTESIAN_POINT('',(-4.94451025515232,0.00421302333877771,43.3223204546569));
#52364=CARTESIAN_POINT('',(-4.94371934458518,0.00435719887056521,43.1776795453432));
#52365=CARTESIAN_POINT('',(-4.942,-6.05220448138622E-16,16.));
#52366=CARTESIAN_POINT('Ctrl Pts',(-4.94451025515232,0.00421302333877771,
43.3223204546569));
#52367=CARTESIAN_POINT('Ctrl Pts',(-4.94721961825891,0.30354166338666,43.3126652883898));
#52368=CARTESIAN_POINT('Ctrl Pts',(-4.9223727794906,0.602421473877891,43.3030101221227));
#52369=CARTESIAN_POINT('Ctrl Pts',(-4.8683572221906,0.895933308008362,43.2933549558557));
#52370=CARTESIAN_POINT('Ctrl Pts',(-4.57229634269635,2.50468041899365,43.2404347017737));
#52371=CARTESIAN_POINT('Ctrl Pts',(-3.39995792978838,3.95216446044364,43.1875144476917));
#52372=CARTESIAN_POINT('Ctrl Pts',(-1.88782194598489,4.57599462800297,43.1345941936098));
#52373=CARTESIAN_POINT('Ctrl Pts',(-0.375685962181428,5.19982479556229,
43.0816739395278));
#52374=CARTESIAN_POINT('Ctrl Pts',(1.47624759251752,5.00000108923096,43.0287536854458));
#52375=CARTESIAN_POINT('Ctrl Pts',(2.82050563945827,4.06796588887349,42.9758334313639));
#52376=CARTESIAN_POINT('Ctrl Pts',(4.16476368639908,3.13593068851599,42.9229131772819));
#52377=CARTESIAN_POINT('Ctrl Pts',(5.00134622558163,1.47168399413228,42.8699929231999));
#52378=CARTESIAN_POINT('Ctrl Pts',(4.9474203102028,-0.163189489389038,42.817072669118));
#52379=CARTESIAN_POINT('Ctrl Pts',(4.89349439482397,-1.79806297291028,42.764152415036));
#52380=CARTESIAN_POINT('Ctrl Pts',(3.94906002488378,-3.40356324556919,42.7112321609541));
#52381=CARTESIAN_POINT('Ctrl Pts',(2.54630479212863,-4.24498886227479,42.6583119068721));
#52382=CARTESIAN_POINT('Ctrl Pts',(1.14354955937346,-5.0864144789804,42.6053916527901));
#52383=CARTESIAN_POINT('Ctrl Pts',(-0.717526536196703,-5.16376543973274,
42.5524713987082));
#52384=CARTESIAN_POINT('Ctrl Pts',(-2.18526664959422,-4.44164476353361,
42.4995511446262));
#52385=CARTESIAN_POINT('Ctrl Pts',(-3.65300676299177,-3.71952408733446,
42.4466308905442));
#52386=CARTESIAN_POINT('Ctrl Pts',(-4.72741089421663,-2.19793177418379,
42.3937106364623));
#52387=CARTESIAN_POINT('Ctrl Pts',(-4.91681530376954,-0.573171705400564,
42.3407903823803));
#52388=CARTESIAN_POINT('Ctrl Pts',(-4.93885025563959,-0.38415018261489,
42.3346337398059));
#52389=CARTESIAN_POINT('Ctrl Pts',(-4.94890712844976,-0.19373232997381,
42.3284770972314));
#52390=CARTESIAN_POINT('Ctrl Pts',(-4.94748713622925,-0.00316321289392352,
42.3223204546569));
#52391=CARTESIAN_POINT('Ctrl Pts',(-4.94809820533655,-0.00280696805152256,
42.1776795453432));
#52392=CARTESIAN_POINT('Ctrl Pts',(-4.94921314716046,-0.166994620502292,
42.1829856132557));
#52393=CARTESIAN_POINT('Ctrl Pts',(-4.94174917029318,-0.331079676814377,
42.1882916811682));
#52394=CARTESIAN_POINT('Ctrl Pts',(-4.92537268191333,-0.494270345953525,
42.1935977490807));
#52395=CARTESIAN_POINT('Ctrl Pts',(-4.76204120174297,-2.12185819764955,
42.2465180031627));
#52396=CARTESIAN_POINT('Ctrl Pts',(-3.71216971888389,-3.6604801046081,42.2994382572447));
#52397=CARTESIAN_POINT('Ctrl Pts',(-2.25619545826342,-4.40603918329588,
42.3523585113266));
#52398=CARTESIAN_POINT('Ctrl Pts',(-0.800221197642949,-5.15159826198366,
42.4052787654086));
#52399=CARTESIAN_POINT('Ctrl Pts',(1.06185584073894,-5.10409451240069,42.4581990194906));
#52400=CARTESIAN_POINT('Ctrl Pts',(2.4779207651768,-4.28526637586659,42.5111192735725));
#52401=CARTESIAN_POINT('Ctrl Pts',(3.89398568961467,-3.46643823933247,42.5640395276545));
#52402=CARTESIAN_POINT('Ctrl Pts',(4.8640385001085,-1.87628571584728,42.6169597817364));
#52403=CARTESIAN_POINT('Ctrl Pts',(4.9441682152519,-0.242486886078373,42.6698800358184));
#52404=CARTESIAN_POINT('Ctrl Pts',(5.02429793039529,1.39131194369048,42.7228002899004));
#52405=CARTESIAN_POINT('Ctrl Pts',(4.21450455018825,3.06875707974299,42.7757205439823));
#52406=CARTESIAN_POINT('Ctrl Pts',(2.88536189314395,4.02222400870711,42.8286407980643));
#52407=CARTESIAN_POINT('Ctrl Pts',(1.55621923609964,4.97569093767124,42.8815610521463));
#52408=CARTESIAN_POINT('Ctrl Pts',(-0.292272697781964,5.20517965954696,
42.9344813062282));
#52409=CARTESIAN_POINT('Ctrl Pts',(-1.81421576809595,4.60567263029181,42.9874015603102));
#52410=CARTESIAN_POINT('Ctrl Pts',(-3.33615883840994,4.00616560103666,43.0403218143921));
#52411=CARTESIAN_POINT('Ctrl Pts',(-4.53155304515633,2.57766282065063,43.0932420684741));
#52412=CARTESIAN_POINT('Ctrl Pts',(-4.85336774243223,0.97386897853116,43.1461623225561));
#52413=CARTESIAN_POINT('Ctrl Pts',(-4.91725446964838,0.655483458634976,
43.1566680634851));
#52414=CARTESIAN_POINT('Ctrl Pts',(-4.94671318283581,0.330189668722103,
43.1671738044142));
#52415=CARTESIAN_POINT('Ctrl Pts',(-4.94371934458518,0.00435719887056521,
43.1776795453432));
#52416=CARTESIAN_POINT('Origin',(0.,0.,16.));
#52417=CARTESIAN_POINT('',(-4.93394997286128,0.000507016503537849,44.3223204546569));
#52418=CARTESIAN_POINT('',(-4.93390371744476,7.29331094537614E-5,44.1776795453432));
#52419=CARTESIAN_POINT('',(-4.942,-6.05220448138622E-16,16.));
#52420=CARTESIAN_POINT('Ctrl Pts',(-4.93394997286128,0.000507016503537849,
44.3223204546569));
#52421=CARTESIAN_POINT('Ctrl Pts',(-4.93467682586532,0.794322762801275,
44.2968534795483));
#52422=CARTESIAN_POINT('Ctrl Pts',(-4.75416264908751,1.58782655048687,44.2713865044396));
#52423=CARTESIAN_POINT('Ctrl Pts',(-4.39062917456631,2.28603892939324,44.245919529331));
#52424=CARTESIAN_POINT('Ctrl Pts',(-3.63520833024163,3.73692095748179,44.192999275249));
#52425=CARTESIAN_POINT('Ctrl Pts',(-2.08949837449215,4.77632854708712,44.1400790211671));
#52426=CARTESIAN_POINT('Ctrl Pts',(-0.460839790231528,4.92861291064672,
44.0871587670851));
#52427=CARTESIAN_POINT('Ctrl Pts',(1.16781879402907,5.08089727420631,44.0342385130031));
#52428=CARTESIAN_POINT('Ctrl Pts',(2.8794260068008,4.3460584117202,43.9813182589212));
#52429=CARTESIAN_POINT('Ctrl Pts',(3.8907242466578,3.06036980963467,43.9283980048392));
#52430=CARTESIAN_POINT('Ctrl Pts',(4.90202248651478,1.77468120754915,43.8754777507573));
#52431=CARTESIAN_POINT('Ctrl Pts',(5.21301175345704,-0.0618571341358118,
43.8225574966753));
#52432=CARTESIAN_POINT('Ctrl Pts',(4.68137860928635,-1.60881722136807,43.7696372425933));
#52433=CARTESIAN_POINT('Ctrl Pts',(4.14974546511566,-3.15577730860032,43.7167169885114));
#52434=CARTESIAN_POINT('Ctrl Pts',(2.77548990983206,-4.41315914137991,43.6637967344294));
#52435=CARTESIAN_POINT('Ctrl Pts',(1.18749227412456,-4.80556558941283,43.6108764803475));
#52436=CARTESIAN_POINT('Ctrl Pts',(-0.400505361582988,-5.19797203744577,
43.5579562262655));
#52437=CARTESIAN_POINT('Ctrl Pts',(-2.20224507771443,-4.72540310073197,
43.5050359721835));
#52438=CARTESIAN_POINT('Ctrl Pts',(-3.3932232627399,-3.60411354211475,43.4521157181016));
#52439=CARTESIAN_POINT('Ctrl Pts',(-4.36691049562677,-2.68740042232609,
43.4088506302867));
#52440=CARTESIAN_POINT('Ctrl Pts',(-4.93236951831919,-1.33708753420181,
43.3655855424718));
#52441=CARTESIAN_POINT('Ctrl Pts',(-4.94451025515232,0.00421302333877771,
43.3223204546569));
#52442=CARTESIAN_POINT('Ctrl Pts',(-4.94371934458518,0.00435719887056521,
43.1776795453432));
#52443=CARTESIAN_POINT('Ctrl Pts',(-4.93163241109647,-1.31111647133373,
43.2200940584961));
#52444=CARTESIAN_POINT('Ctrl Pts',(-4.39058351177215,-2.63537038181765,
43.262508571649));
#52445=CARTESIAN_POINT('Ctrl Pts',(-3.45056931084653,-3.5492493095965,43.3049230848019));
#52446=CARTESIAN_POINT('Ctrl Pts',(-2.27772099417954,-4.68948885175174,
43.3578433388839));
#52447=CARTESIAN_POINT('Ctrl Pts',(-0.483789173040172,-5.19088303220938,
43.4107635929659));
#52448=CARTESIAN_POINT('Ctrl Pts',(1.11029555303778,-4.82398621634968,43.4636838470478));
#52449=CARTESIAN_POINT('Ctrl Pts',(2.70438027911579,-4.45708940048996,43.5166041011298));
#52450=CARTESIAN_POINT('Ctrl Pts',(4.09861791013234,-3.22190158831284,43.5695243552118));
#52451=CARTESIAN_POINT('Ctrl Pts',(4.65498401236277,-1.68366358732205,43.6224446092938));
#52452=CARTESIAN_POINT('Ctrl Pts',(5.21135011459319,-0.145425586331283,
43.6753648633757));
#52453=CARTESIAN_POINT('Ctrl Pts',(4.92984468803749,1.69586260347318,43.7282851174576));
#52454=CARTESIAN_POINT('Ctrl Pts',(3.93928891523517,2.99759938499667,43.7812053715396));
#52455=CARTESIAN_POINT('Ctrl Pts',(2.94873314243287,4.29933616652015,43.8341256256216));
#52456=CARTESIAN_POINT('Ctrl Pts',(1.24912702338399,5.06152153976273,43.8870458797035));
#52457=CARTESIAN_POINT('Ctrl Pts',(-0.381763724262289,4.93536783730094,
43.9399661337855));
#52458=CARTESIAN_POINT('Ctrl Pts',(-2.01265447190855,4.80921413483915,43.9928863878675));
#52459=CARTESIAN_POINT('Ctrl Pts',(-3.57482984815219,3.79472135667302,44.0458066419495));
#52460=CARTESIAN_POINT('Ctrl Pts',(-4.35341454219008,2.35613689213404,44.0987268960314));
#52461=CARTESIAN_POINT('Ctrl Pts',(-4.74060923336151,1.6407204811301,44.125044445802));
#52462=CARTESIAN_POINT('Ctrl Pts',(-4.93401170909488,0.820420654182907,
44.1513619955726));
#52463=CARTESIAN_POINT('Ctrl Pts',(-4.93390371744476,7.29331094537614E-5,
44.1776795453432));
#52464=CARTESIAN_POINT('Origin',(0.,0.,16.));
#52465=CARTESIAN_POINT('',(-4.94264971735337,-0.00447858357024544,45.3223204546569));
#52466=CARTESIAN_POINT('',(-4.94345166054126,-0.00439535110808767,45.1776795453432));
#52467=CARTESIAN_POINT('',(-4.942,-6.05220448138622E-16,16.));
#52468=CARTESIAN_POINT('Ctrl Pts',(-4.94264971735337,-0.00447858357024544,
45.3223204546569));
#52469=CARTESIAN_POINT('Ctrl Pts',(-4.93082575729553,1.27648252745284,45.2810416707067));
#52470=CARTESIAN_POINT('Ctrl Pts',(-4.42134998955586,2.56578412734584,45.2397628867565));
#52471=CARTESIAN_POINT('Ctrl Pts',(-3.52575508348954,3.47457186233093,45.1984841028063));
#52472=CARTESIAN_POINT('Ctrl Pts',(-2.37758390575486,4.63965651937944,45.1455638487244));
#52473=CARTESIAN_POINT('Ctrl Pts',(-0.594796197848898,5.17933734465609,
45.0926435946425));
#52474=CARTESIAN_POINT('Ctrl Pts',(1.00677715711088,4.84664815013159,45.0397233405605));
#52475=CARTESIAN_POINT('Ctrl Pts',(2.60835051207067,4.51395895560708,44.9868030864785));
#52476=CARTESIAN_POINT('Ctrl Pts',(4.02870951408424,3.30889974128137,44.9338828323965));
#52477=CARTESIAN_POINT('Ctrl Pts',(4.61787619111481,1.78292400813641,44.8809625783145));
#52478=CARTESIAN_POINT('Ctrl Pts',(5.20704286814536,0.25694827499149,44.8280423242326));
#52479=CARTESIAN_POINT('Ctrl Pts',(4.96501722019298,-1.58994397697268,44.7751220701506));
#52480=CARTESIAN_POINT('Ctrl Pts',(4.00255388014552,-2.91258664622809,44.7222018160687));
#52481=CARTESIAN_POINT('Ctrl Pts',(3.04009054009802,-4.23522931548356,44.6692815619867));
#52482=CARTESIAN_POINT('Ctrl Pts',(1.35718950795542,-5.03362240203022,44.6163613079047));
#52483=CARTESIAN_POINT('Ctrl Pts',(-0.276028001533181,-4.94240903584718,
44.5634410538228));
#52484=CARTESIAN_POINT('Ctrl Pts',(-1.90924551102172,-4.85119566966413,
44.5105207997408));
#52485=CARTESIAN_POINT('Ctrl Pts',(-3.49277949785625,-3.8703758507514,44.4576005456588));
#52486=CARTESIAN_POINT('Ctrl Pts',(-4.30198062482356,-2.4487877080092,44.4046802915769));
#52487=CARTESIAN_POINT('Ctrl Pts',(-4.72176742799645,-1.71131475847591,
44.3772270126036));
#52488=CARTESIAN_POINT('Ctrl Pts',(-4.93316642875337,-0.85522261151742,
44.3497737336302));
#52489=CARTESIAN_POINT('Ctrl Pts',(-4.93394997286128,0.000507016503537849,
44.3223204546569));
#52490=CARTESIAN_POINT('Ctrl Pts',(-4.93390371744476,7.29331094537614E-5,
44.1776795453432));
#52491=CARTESIAN_POINT('Ctrl Pts',(-4.93379455568915,-0.829163376745596,
44.2042822496546));
#52492=CARTESIAN_POINT('Ctrl Pts',(-4.73595877931974,-1.65844862422957,
44.2308849539659));
#52493=CARTESIAN_POINT('Ctrl Pts',(-4.34068739432695,-2.37950250585247,
44.2574876582773));
#52494=CARTESIAN_POINT('Ctrl Pts',(-3.55438154059382,-3.813881288388,44.3104079123592));
#52495=CARTESIAN_POINT('Ctrl Pts',(-1.98677582129545,-4.81996270254719,
44.3633281664412));
#52496=CARTESIAN_POINT('Ctrl Pts',(-0.355230555152893,-4.9373485276323,
44.4162484205232));
#52497=CARTESIAN_POINT('Ctrl Pts',(1.27631471098969,-5.05473435271742,44.4691686746052));
#52498=CARTESIAN_POINT('Ctrl Pts',(2.97179952397649,-4.28342458872844,44.5220889286871));
#52499=CARTESIAN_POINT('Ctrl Pts',(3.95534413875573,-2.9763823636485,44.5750091827691));
#52500=CARTESIAN_POINT('Ctrl Pts',(4.93888875353493,-1.66934013856861,44.627929436851));
#52501=CARTESIAN_POINT('Ctrl Pts',(5.21049317010665,0.173434547602146,44.680849690933));
#52502=CARTESIAN_POINT('Ctrl Pts',(4.64586705931524,1.70865985432931,44.733769945015));
#52503=CARTESIAN_POINT('Ctrl Pts',(4.08124094852381,3.24388516105654,44.7866901990969));
#52504=CARTESIAN_POINT('Ctrl Pts',(2.68038431036912,4.47156108834011,44.8396104531789));
#52505=CARTESIAN_POINT('Ctrl Pts',(1.08435053733238,4.82988438193028,44.8925307072609));
#52506=CARTESIAN_POINT('Ctrl Pts',(-0.511683235704347,5.18820767552046,
44.9454509613428));
#52507=CARTESIAN_POINT('Ctrl Pts',(-2.30289414362315,4.67717833541725,44.9983712154248));
#52508=CARTESIAN_POINT('Ctrl Pts',(-3.46959671833554,3.53065119244912,45.0512914695067));
#52509=CARTESIAN_POINT('Ctrl Pts',(-4.39839859233384,2.61791080594467,45.0934208281189));
#52510=CARTESIAN_POINT('Ctrl Pts',(-4.93141112790613,1.30241637823199,45.1355501867311));
#52511=CARTESIAN_POINT('Ctrl Pts',(-4.94345166054126,-0.00439535110808767,
45.1776795453432));
#52512=CARTESIAN_POINT('Origin',(0.,0.,16.));
#52513=CARTESIAN_POINT('',(-4.94881445934699,0.00227942523971326,46.3223204546569));
#52514=CARTESIAN_POINT('',(-4.94828946219151,0.00267981890309541,46.1776795453432));
#52515=CARTESIAN_POINT('',(-4.942,-6.05220448138622E-16,16.));
#52516=CARTESIAN_POINT('Ctrl Pts',(-4.94881445934699,0.00227942523971326,
46.3223204546569));
#52517=CARTESIAN_POINT('Ctrl Pts',(-4.94955378308614,0.131274482234953,
46.3181501159471));
#52518=CARTESIAN_POINT('Ctrl Pts',(-4.94494719039334,0.260215895992481,
46.3139797772374));
#52519=CARTESIAN_POINT('Ctrl Pts',(-4.93482452766902,0.388722801454193,
46.3098094385276));
#52520=CARTESIAN_POINT('Ctrl Pts',(-4.80637120034064,2.01943401260374,46.2568891844456));
#52521=CARTESIAN_POINT('Ctrl Pts',(-3.78967659005442,3.58017725671765,46.2039689303636));
#52522=CARTESIAN_POINT('Ctrl Pts',(-2.34999567814797,4.35673258852779,46.1510486762817));
#52523=CARTESIAN_POINT('Ctrl Pts',(-0.910314766241556,5.13328792033792,
46.0981284221997));
#52524=CARTESIAN_POINT('Ctrl Pts',(0.952352447285067,5.12565533984434,46.0452081681177));
#52525=CARTESIAN_POINT('Ctrl Pts',(2.38562099756669,4.33732763245101,45.9922879140358));
#52526=CARTESIAN_POINT('Ctrl Pts',(3.81888954784836,3.54899992505766,45.9393676599538));
#52527=CARTESIAN_POINT('Ctrl Pts',(4.82275943488501,1.97997709076453,45.8864474058719));
#52528=CARTESIAN_POINT('Ctrl Pts',(4.93784446656618,0.348267941757418,45.8335271517899));
#52529=CARTESIAN_POINT('Ctrl Pts',(5.05292949824735,-1.28344120724965,45.7806068977079));
#52530=CARTESIAN_POINT('Ctrl Pts',(4.27922967457309,-2.97783667097068,45.727686643626));
#52531=CARTESIAN_POINT('Ctrl Pts',(2.97080185134115,-3.95953720721528,45.674766389544));
#52532=CARTESIAN_POINT('Ctrl Pts',(1.66237402810921,-4.94123774345989,45.621846135462));
#52533=CARTESIAN_POINT('Ctrl Pts',(-0.18078179468041,-5.21024335222807,
45.5689258813801));
#52534=CARTESIAN_POINT('Ctrl Pts',(-1.71520936255536,-4.64345295850584,
45.5160056272981));
#52535=CARTESIAN_POINT('Ctrl Pts',(-3.24963693043034,-4.0766625647836,45.4630853732162));
#52536=CARTESIAN_POINT('Ctrl Pts',(-4.47533624339064,-2.67407616857091,
45.4101651191342));
#52537=CARTESIAN_POINT('Ctrl Pts',(-4.8314085760891,-1.07753872605438,45.3572448650522));
#52538=CARTESIAN_POINT('Ctrl Pts',(-4.90973785658425,-0.726330228027688,
45.3456033949204));
#52539=CARTESIAN_POINT('Ctrl Pts',(-4.94598431844091,-0.365736088925451,
45.3339619247887));
#52540=CARTESIAN_POINT('Ctrl Pts',(-4.94264971735337,-0.00447858357024544,
45.3223204546569));
#52541=CARTESIAN_POINT('Ctrl Pts',(-4.94345166054126,-0.00439535110808767,
45.1776795453432));
#52542=CARTESIAN_POINT('Ctrl Pts',(-4.94653568871891,-0.339118433408757,
45.188470440813));
#52543=CARTESIAN_POINT('Ctrl Pts',(-4.91544069255685,-0.673271876348126,
45.1992613362828));
#52544=CARTESIAN_POINT('Ctrl Pts',(-4.848063077171,-0.999941813506336,45.2100522317526));
#52545=CARTESIAN_POINT('Ctrl Pts',(-4.51763261978812,-2.60198273066066,
45.2629724858346));
#52546=CARTESIAN_POINT('Ctrl Pts',(-3.31457746351644,-4.02403961913634,
45.3158927399166));
#52547=CARTESIAN_POINT('Ctrl Pts',(-1.78943402176491,-4.61535752812037,
45.3688129939985));
#52548=CARTESIAN_POINT('Ctrl Pts',(-0.264290580013278,-5.20667543710444,
45.4217332480805));
#52549=CARTESIAN_POINT('Ctrl Pts',(1.58294114721826,-4.96725436659668,45.4746535021624));
#52550=CARTESIAN_POINT('Ctrl Pts',(2.90693970933454,-4.00665705506737,45.5275737562444));
#52551=CARTESIAN_POINT('Ctrl Pts',(4.23093827145077,-3.0460597435381,45.5804940103263));
#52552=CARTESIAN_POINT('Ctrl Pts',(5.0317036684518,-1.36428619098739,45.6334142644083));
#52553=CARTESIAN_POINT('Ctrl Pts',(4.94279342482124,0.2690583397166,45.6863345184903));
#52554=CARTESIAN_POINT('Ctrl Pts',(4.85388318119067,1.90240287042061,45.7392547725723));
#52555=CARTESIAN_POINT('Ctrl Pts',(3.87529729692844,3.4873183792779,45.7921750266543));
#52556=CARTESIAN_POINT('Ctrl Pts',(2.45485161832049,4.29852332349801,45.8450952807362));
#52557=CARTESIAN_POINT('Ctrl Pts',(1.03440593971258,5.1097282677181,45.8980155348182));
#52558=CARTESIAN_POINT('Ctrl Pts',(-0.827899533241065,5.1472226473011,45.9509357889001));
#52559=CARTESIAN_POINT('Ctrl Pts',(-2.27984537368615,4.39384846150945,46.0038560429821));
#52560=CARTESIAN_POINT('Ctrl Pts',(-3.73179121413126,3.64047427571779,46.056776297064));
#52561=CARTESIAN_POINT('Ctrl Pts',(-4.77337742206781,2.0962315245515,46.109696551146));
#52562=CARTESIAN_POINT('Ctrl Pts',(-4.92795824091158,0.46778927569873,46.162616805228));
#52563=CARTESIAN_POINT('Ctrl Pts',(-4.94262440066108,0.31328760891278,46.1676377185997));
#52564=CARTESIAN_POINT('Ctrl Pts',(-4.94930605767903,0.158028008604056,
46.1726586319715));
#52565=CARTESIAN_POINT('Ctrl Pts',(-4.94828946219151,0.00267981890309541,
46.1776795453432));
#52566=CARTESIAN_POINT('Origin',(0.,0.,16.));
#52567=CARTESIAN_POINT('',(-4.9358501160701,0.00303175399314515,47.3223204546569));
#52568=CARTESIAN_POINT('',(-4.93538463697233,0.00269292579073279,47.1776795453432));
#52569=CARTESIAN_POINT('',(-4.942,-6.05220448138622E-16,16.));
#52570=CARTESIAN_POINT('Ctrl Pts',(-4.9358501160701,0.00303175399314515,
47.3223204546569));
#52571=CARTESIAN_POINT('Ctrl Pts',(-4.93933793021421,0.625283723714611,
47.3023383071056));
#52572=CARTESIAN_POINT('Ctrl Pts',(-4.83028758168748,1.24635811395051,47.2823561595543));
#52573=CARTESIAN_POINT('Ctrl Pts',(-4.60310972348256,1.82070849089976,47.2623740120029));
#52574=CARTESIAN_POINT('Ctrl Pts',(-4.00145717602152,3.34180464946569,47.2094537579209));
#52575=CARTESIAN_POINT('Ctrl Pts',(-2.57127018656423,4.53518329005682,47.156533503839));
#52576=CARTESIAN_POINT('Ctrl Pts',(-0.967024164301558,4.85473612062603,
47.103613249757));
#52577=CARTESIAN_POINT('Ctrl Pts',(0.637221857961163,5.17428895119525,47.050692995675));
#52578=CARTESIAN_POINT('Ctrl Pts',(2.41552691302929,4.62001597174252,46.9977727415931));
#52579=CARTESIAN_POINT('Ctrl Pts',(3.55411144818602,3.44556096290971,46.9448524875111));
#52580=CARTESIAN_POINT('Ctrl Pts',(4.69269598334273,2.27110595407693,46.8919322334292));
#52581=CARTESIAN_POINT('Ctrl Pts',(5.19155999858808,0.476468915864107,46.8390119793472));
#52582=CARTESIAN_POINT('Ctrl Pts',(4.82241570154595,-1.11709683409153,46.7860917252652));
#52583=CARTESIAN_POINT('Ctrl Pts',(4.45327140450381,-2.71066258404717,46.7331714711833));
#52584=CARTESIAN_POINT('Ctrl Pts',(3.21611879517418,-4.10315704574563,46.6802512171013));
#52585=CARTESIAN_POINT('Ctrl Pts',(1.67709780224552,-4.65735348636513,46.6273309630194));
#52586=CARTESIAN_POINT('Ctrl Pts',(0.138076809316829,-5.21154992698464,
46.5744107089374));
#52587=CARTESIAN_POINT('Ctrl Pts',(-1.7028125672109,-4.92744834652514,46.5214904548554));
#52588=CARTESIAN_POINT('Ctrl Pts',(-3.00315123328947,-3.93505796720279,
46.4685702007734));
#52589=CARTESIAN_POINT('Ctrl Pts',(-4.2010177406636,-3.02087212574391,46.4198202854013));
#52590=CARTESIAN_POINT('Ctrl Pts',(-4.94017200312835,-1.50563121453851,
46.3710703700291));
#52591=CARTESIAN_POINT('Ctrl Pts',(-4.94881445934699,0.00227942523971326,
46.3223204546569));
#52592=CARTESIAN_POINT('Ctrl Pts',(-4.94828946219151,0.00267981890309541,
46.1776795453432));
#52593=CARTESIAN_POINT('Ctrl Pts',(-4.93859117623925,-1.47933656262951,
46.2255788860534));
#52594=CARTESIAN_POINT('Ctrl Pts',(-4.22826766932132,-2.96941554830109,
46.2734782267636));
#52595=CARTESIAN_POINT('Ctrl Pts',(-3.06585319961028,-3.88640494404102,
46.3213775674738));
#52596=CARTESIAN_POINT('Ctrl Pts',(-1.78159190971431,-4.89951516838867,
46.3742978215558));
#52597=CARTESIAN_POINT('Ctrl Pts',(0.0545060998286173,-5.21309387054478,
46.4272180756378));
#52598=CARTESIAN_POINT('Ctrl Pts',(1.60221433767964,-4.68364264720964,46.4801383297198));
#52599=CARTESIAN_POINT('Ctrl Pts',(3.14992257553069,-4.15419142387448,46.5330585838017));
#52600=CARTESIAN_POINT('Ctrl Pts',(4.40924104168984,-2.78171027504809,46.5859788378836));
#52601=CARTESIAN_POINT('Ctrl Pts',(4.80388637285101,-1.19426753592463,46.6388990919656));
#52602=CARTESIAN_POINT('Ctrl Pts',(5.19853170401218,0.393175203198827,46.6918193460476));
#52603=CARTESIAN_POINT('Ctrl Pts',(4.72850390017529,2.19557953261941,46.7447396001296));
#52604=CARTESIAN_POINT('Ctrl Pts',(3.60889486296925,3.38813770361555,46.7976598542115));
#52605=CARTESIAN_POINT('Ctrl Pts',(2.48928582576321,4.58069587461169,46.8505801082935));
#52606=CARTESIAN_POINT('Ctrl Pts',(0.720095555188062,5.16340788718348,46.9035003623755));
#52607=CARTESIAN_POINT('Ctrl Pts',(-0.889067460630859,4.86961582479301,
46.9564206164574));
#52608=CARTESIAN_POINT('Ctrl Pts',(-2.49823047644978,4.57582376240254,47.0093408705394));
#52609=CARTESIAN_POINT('Ctrl Pts',(-3.9473662375124,3.40552762504981,47.0622611246213));
#52610=CARTESIAN_POINT('Ctrl Pts',(-4.57332808734244,1.89427279876787,47.1151813787033));
#52611=CARTESIAN_POINT('Ctrl Pts',(-4.81974582587867,1.29934836887573,47.1360141009166));
#52612=CARTESIAN_POINT('Ctrl Pts',(-4.93859613551441,0.651585501425685,
47.1568468231299));
#52613=CARTESIAN_POINT('Ctrl Pts',(-4.93538463697233,0.00269292579073279,
47.1776795453432));
#52614=CARTESIAN_POINT('Origin',(0.,0.,16.));
#52615=CARTESIAN_POINT('',(-4.93779824682792,-0.00394849367342132,48.3223204546569));
#52616=CARTESIAN_POINT('',(-4.93847649956811,-0.00414486738929824,48.1776795453433));
#52617=CARTESIAN_POINT('',(-4.942,-6.05220448138622E-16,16.));
#52618=CARTESIAN_POINT('Ctrl Pts',(-4.93779824682792,-0.00394849367342132,
48.3223204546569));
#52619=CARTESIAN_POINT('Ctrl Pts',(-4.92945107906705,1.10958389040538,48.286526498264));
#52620=CARTESIAN_POINT('Ctrl Pts',(-4.55663414200584,2.22817899674935,48.2507325418711));
#52621=CARTESIAN_POINT('Ctrl Pts',(-3.86551329136296,3.09215224876629,48.2149385854782));
#52622=CARTESIAN_POINT('Ctrl Pts',(-2.8437125545035,4.36950989861378,48.1620183313963));
#52623=CARTESIAN_POINT('Ctrl Pts',(-1.12614067807074,5.09029714456033,48.1090980773143));
#52624=CARTESIAN_POINT('Ctrl Pts',(0.50121521532169,4.92467073449426,48.0561778232323));
#52625=CARTESIAN_POINT('Ctrl Pts',(2.12857110871417,4.75904432442819,48.0032575691504));
#52626=CARTESIAN_POINT('Ctrl Pts',(3.66571101906626,3.70700425834946,47.9503373150684));
#52627=CARTESIAN_POINT('Ctrl Pts',(4.40921624712591,2.2499801379868,47.8974170609865));
#52628=CARTESIAN_POINT('Ctrl Pts',(5.15272147518552,0.792956017624232,47.8444968069045));
#52629=CARTESIAN_POINT('Ctrl Pts',(5.10259202095273,-1.06905215702231,47.7915765528226));
#52630=CARTESIAN_POINT('Ctrl Pts',(4.28176788829653,-2.4839610073443,47.7386562987406));
#52631=CARTESIAN_POINT('Ctrl Pts',(3.46094375564028,-3.89886985766637,47.6857360446586));
#52632=CARTESIAN_POINT('Ctrl Pts',(1.86942494456057,-4.86667938366393,47.6328157905766));
#52633=CARTESIAN_POINT('Ctrl Pts',(0.235514769794999,-4.94450516517706,
47.5798955364947));
#52634=CARTESIAN_POINT('Ctrl Pts',(-1.39839540497048,-5.02233094669018,
47.5269752824127));
#52635=CARTESIAN_POINT('Ctrl Pts',(-3.07469694342178,-4.21017298371899,
47.4740550283308));
#52636=CARTESIAN_POINT('Ctrl Pts',(-4.02628865991507,-2.87968716396305,
47.4211347742488));
#52637=CARTESIAN_POINT('Ctrl Pts',(-4.61856906134665,-2.05157920362054,
47.3881966677182));
#52638=CARTESIAN_POINT('Ctrl Pts',(-4.93010088448512,-1.0226738972605,47.3552585611876));
#52639=CARTESIAN_POINT('Ctrl Pts',(-4.9358501160701,0.00303175399314515,
47.3223204546569));
#52640=CARTESIAN_POINT('Ctrl Pts',(-4.93538463697233,0.00269292579073279,
47.1776795453432));
#52641=CARTESIAN_POINT('Ctrl Pts',(-4.93043813690577,-0.996761729574154,
47.2097670772119));
#52642=CARTESIAN_POINT('Ctrl Pts',(-4.63591709407219,-1.99889645937005,
47.2418546090805));
#52643=CARTESIAN_POINT('Ctrl Pts',(-4.07193915439288,-2.81476655400573,
47.2739421409492));
#52644=CARTESIAN_POINT('Ctrl Pts',(-3.1418004330159,-4.16033756528617,47.3268623950311));
#52645=CARTESIAN_POINT('Ctrl Pts',(-1.47873505166457,-4.99926607263594,
47.3797826491131));
#52646=CARTESIAN_POINT('Ctrl Pts',(0.156212871657996,-4.94764557838933,
47.4327029031951));
#52647=CARTESIAN_POINT('Ctrl Pts',(1.79116079498061,-4.89602508414272,47.4856231572771));
#52648=CARTESIAN_POINT('Ctrl Pts',(3.39799126027446,-3.95385558829969,47.538543411359));
#52649=CARTESIAN_POINT('Ctrl Pts',(4.24139410598325,-2.552288241629,47.591463665441));
#52650=CARTESIAN_POINT('Ctrl Pts',(5.08479695169201,-1.15072089495835,47.6443839195229));
#52651=CARTESIAN_POINT('Ctrl Pts',(5.16477217781576,0.710244302539926,47.6973041736049));
#52652=CARTESIAN_POINT('Ctrl Pts',(4.44472189944271,2.17900125452958,47.7502244276869));
#52653=CARTESIAN_POINT('Ctrl Pts',(3.72467162106964,3.64775820651928,47.8031446817689));
#52654=CARTESIAN_POINT('Ctrl Pts',(2.20459583819974,4.72430691300034,47.8560649358508));
#52655=CARTESIAN_POINT('Ctrl Pts',(0.580104444733958,4.91600224408279,47.9089851899327));
#52656=CARTESIAN_POINT('Ctrl Pts',(-1.04438694873177,5.10769757516524,47.9619054440147));
#52657=CARTESIAN_POINT('Ctrl Pts',(-2.77329395279337,4.41453953084916,48.0148256980967));
#52658=CARTESIAN_POINT('Ctrl Pts',(-3.81544231731622,3.15372781860764,48.0677459521787));
#52659=CARTESIAN_POINT('Ctrl Pts',(-4.53707600502276,2.28068110435693,48.1043904832335));
#52660=CARTESIAN_POINT('Ctrl Pts',(-4.92941962837742,1.13545330336185,48.1410350142884));
#52661=CARTESIAN_POINT('Ctrl Pts',(-4.93847649956811,-0.00414486738929824,
48.1776795453433));
#52662=CARTESIAN_POINT('Origin',(0.,0.,16.));
#52663=CARTESIAN_POINT('',(-4.94996872029631,-0.000754789231165454,49.3223204546569));
#52664=CARTESIAN_POINT('',(-4.95009281286112,-0.000267728824007536,49.1776795453432));
#52665=CARTESIAN_POINT('',(-4.942,-6.05220448138622E-16,16.));
#52666=CARTESIAN_POINT('Ctrl Pts',(-4.94996872029631,-0.000754789231165454,
49.3223204546569));
#52667=CARTESIAN_POINT('Ctrl Pts',(-4.94657205241788,1.59450047399929,49.2707146894224));
#52668=CARTESIAN_POINT('Ctrl Pts',(-4.10534559557285,3.19283284813315,49.219108924188));
#52669=CARTESIAN_POINT('Ctrl Pts',(-2.78707318578254,4.09094385103807,49.1675031589536));
#52670=CARTESIAN_POINT('Ctrl Pts',(-1.4352220784804,5.01193130760659,49.1145829048716));
#52671=CARTESIAN_POINT('Ctrl Pts',(0.418286878732396,5.19657136329379,49.0616626507896));
#52672=CARTESIAN_POINT('Ctrl Pts',(1.92525967895112,4.56036990866522,49.0087423967077));
#52673=CARTESIAN_POINT('Ctrl Pts',(3.4322324791698,3.92416845403667,48.9558221426257));
#52674=CARTESIAN_POINT('Ctrl Pts',(4.59266912239443,2.4671254890924,48.9029018885438));
#52675=CARTESIAN_POINT('Ctrl Pts',(4.87553607768602,0.856006127569342,48.8499816344618));
#52676=CARTESIAN_POINT('Ctrl Pts',(5.15840303297761,-0.755113233953766,
48.7970613803799));
#52677=CARTESIAN_POINT('Ctrl Pts',(4.56370030033613,-2.52030899205568,48.7441411262979));
#52678=CARTESIAN_POINT('Ctrl Pts',(3.36357293293406,-3.63180060852569,48.6912208722159));
#52679=CARTESIAN_POINT('Ctrl Pts',(2.16344556553202,-4.74329222499568,48.6383006181339));
#52680=CARTESIAN_POINT('Ctrl Pts',(0.357893563369426,-5.20107969983381,
48.585380364052));
#52681=CARTESIAN_POINT('Ctrl Pts',(-1.22683490171212,-4.79567249290391,
48.53246010997));
#52682=CARTESIAN_POINT('Ctrl Pts',(-2.81156336679367,-4.39026528597401,
48.4795398558881));
#52683=CARTESIAN_POINT('Ctrl Pts',(-4.17546829479417,-3.12166339727609,
48.4266196018061));
#52684=CARTESIAN_POINT('Ctrl Pts',(-4.69440596015137,-1.57039842605291,
48.3736993477241));
#52685=CARTESIAN_POINT('Ctrl Pts',(-4.86234697051046,-1.0683708724689,48.356573050035));
#52686=CARTESIAN_POINT('Ctrl Pts',(-4.94179210764521,-0.536739194059861,
48.339446752346));
#52687=CARTESIAN_POINT('Ctrl Pts',(-4.93779824682792,-0.00394849367342132,
48.3223204546569));
#52688=CARTESIAN_POINT('Ctrl Pts',(-4.93847649956811,-0.00414486738929824,
48.1776795453433));
#52689=CARTESIAN_POINT('Ctrl Pts',(-4.942499122392,-0.510299091646249,48.1939552683704));
#52690=CARTESIAN_POINT('Ctrl Pts',(-4.87091055869885,-1.01534275567644,
48.2102309913974));
#52691=CARTESIAN_POINT('Ctrl Pts',(-4.7189797263556,-1.49493463832769,48.2265067144245));
#52692=CARTESIAN_POINT('Ctrl Pts',(-4.224979045888,-3.05432000285457,48.2794269685065));
#52693=CARTESIAN_POINT('Ctrl Pts',(-2.88158795996869,-4.34462535174135,
48.3323472225885));
#52694=CARTESIAN_POINT('Ctrl Pts',(-1.30356274672183,-4.77538725089245,
48.3852674766704));
#52695=CARTESIAN_POINT('Ctrl Pts',(0.274462466525034,-5.20614915004355,
48.4381877307524));
#52696=CARTESIAN_POINT('Ctrl Pts',(2.08712180709941,-4.77736759945896,48.4911079848343));
#52697=CARTESIAN_POINT('Ctrl Pts',(3.30491467655429,-3.68525958533767,48.5440282389163));
#52698=CARTESIAN_POINT('Ctrl Pts',(4.5227075460092,-2.59315157121635,48.5969484929983));
#52699=CARTESIAN_POINT('Ctrl Pts',(5.14563394434455,-0.837717093558183,
48.6498687470803));
#52700=CARTESIAN_POINT('Ctrl Pts',(4.88863323791471,0.7777302204381,48.7027890011622));
#52701=CARTESIAN_POINT('Ctrl Pts',(4.63163253148487,2.39317753443434,48.7557092552442));
#52702=CARTESIAN_POINT('Ctrl Pts',(3.49470472029,3.86863768476876,48.8086295093261));
#52703=CARTESIAN_POINT('Ctrl Pts',(1.99812533468889,4.52891757238984,48.8615497634081));
#52704=CARTESIAN_POINT('Ctrl Pts',(0.501545949087793,5.18919746001092,48.91447001749));
#52705=CARTESIAN_POINT('Ctrl Pts',(-1.35468501091949,5.03429708491863,48.967390271572));
#52706=CARTESIAN_POINT('Ctrl Pts',(-2.7211279083772,4.13510122450199,49.020310525654));
#52707=CARTESIAN_POINT('Ctrl Pts',(-4.07559217393182,3.24378797391906,49.0727668655504));
#52708=CARTESIAN_POINT('Ctrl Pts',(-4.94881798417885,1.62117145762289,49.1252232054468));
#52709=CARTESIAN_POINT('Ctrl Pts',(-4.95009281286112,-0.000267728824007536,
49.1776795453432));
#52710=CARTESIAN_POINT('Origin',(0.,0.,16.));
#52711=CARTESIAN_POINT('',(-4.94000433004934,0.00442567287284368,50.3223204546569));
#52712=CARTESIAN_POINT('',(-4.93925722597112,0.00431400617654748,50.1776795453432));
#52713=CARTESIAN_POINT('',(-4.942,-6.05220448138622E-16,16.));
#52714=CARTESIAN_POINT('Ctrl Pts',(-4.94000433004934,0.00442567287284368,
50.3223204546569));
#52715=CARTESIAN_POINT('Ctrl Pts',(-4.94391985550658,0.454920647205931,
50.3078231346629));
#52716=CARTESIAN_POINT('Ctrl Pts',(-4.88736862134446,0.904450331901516,
50.2933258146688));
#52717=CARTESIAN_POINT('Ctrl Pts',(-4.76643244788693,1.33593422554585,50.2788284946748));
#52718=CARTESIAN_POINT('Ctrl Pts',(-4.3249734037525,2.91100032695947,50.2259082405929));
#52719=CARTESIAN_POINT('Ctrl Pts',(-3.02558272518919,4.24560561283798,50.1729879865109));
#52720=CARTESIAN_POINT('Ctrl Pts',(-1.46288143191014,4.72901432133872,50.120067732429));
#52721=CARTESIAN_POINT('Ctrl Pts',(0.0998198613689605,5.21242302983948,
50.067147478347));
#52722=CARTESIAN_POINT('Ctrl Pts',(1.92583176936386,4.84463516096244,50.014227224265));
#52723=CARTESIAN_POINT('Ctrl Pts',(3.17954335484605,3.79395606061911,49.961306970183));
#52724=CARTESIAN_POINT('Ctrl Pts',(4.43325494032821,2.74327696027582,49.9083867161011));
#52725=CARTESIAN_POINT('Ctrl Pts',(5.11466620329769,1.00970662846638,49.8554664620191));
#52726=CARTESIAN_POINT('Ctrl Pts',(4.91195294283073,-0.613446674675755,
49.8025462079371));
#52727=CARTESIAN_POINT('Ctrl Pts',(4.70923968236377,-2.23659997781789,49.7496259538552));
#52728=CARTESIAN_POINT('Ctrl Pts',(3.62240189846027,-3.74933625229266,49.6967056997732));
#52729=CARTESIAN_POINT('Ctrl Pts',(2.14879315998069,-4.45940427533482,49.6437854456913));
#52730=CARTESIAN_POINT('Ctrl Pts',(0.675184421501018,-5.16947229837701,
49.5908651916093));
#52731=CARTESIAN_POINT('Ctrl Pts',(-1.18519527155483,-5.0768720699865,49.5379449375273));
#52732=CARTESIAN_POINT('Ctrl Pts',(-2.58100775862557,-4.22397886893019,
49.4850246834454));
#52733=CARTESIAN_POINT('Ctrl Pts',(-3.97682024569624,-3.37108566787394,
49.4321044293634));
#52734=CARTESIAN_POINT('Ctrl Pts',(-4.9080655267819,-1.75789949415196,49.3791841752814));
#52735=CARTESIAN_POINT('Ctrl Pts',(-4.94859153862899,-0.12263897856609,
49.3262639211994));
#52736=CARTESIAN_POINT('Ctrl Pts',(-4.94959816627151,-0.0820206605359307,
49.3249494323519));
#52737=CARTESIAN_POINT('Ctrl Pts',(-4.9500552393514,-0.0413887231133244,
49.3236349435044));
#52738=CARTESIAN_POINT('Ctrl Pts',(-4.94996872029631,-0.000754789231165454,
49.3223204546569));
#52739=CARTESIAN_POINT('Ctrl Pts',(-4.95009281286112,-0.000267728824007536,
49.1776795453432));
#52740=CARTESIAN_POINT('Ctrl Pts',(-4.95010408721063,-0.0146074376385199,
49.1781434595288));
#52741=CARTESIAN_POINT('Ctrl Pts',(-4.95004716359657,-0.02894705437045,
49.1786073737143));
#52742=CARTESIAN_POINT('Ctrl Pts',(-4.94992177176232,-0.0432860723615371,
49.1790712878999));
#52743=CARTESIAN_POINT('Ctrl Pts',(-4.93561790278161,-1.6789861630675,49.2319915419818));
#52744=CARTESIAN_POINT('Ctrl Pts',(-4.03035532991194,-3.30689499873837,
49.2849117960638));
#52745=CARTESIAN_POINT('Ctrl Pts',(-2.6483960323012,-4.18205663360964,49.3378320501458));
#52746=CARTESIAN_POINT('Ctrl Pts',(-1.26643673469055,-5.05721826848085,
49.3907523042277));
#52747=CARTESIAN_POINT('Ctrl Pts',(0.592219287661027,-5.17963270255261,
49.4436725583097));
#52748=CARTESIAN_POINT('Ctrl Pts',(2.07702265223193,-4.49328122119488,49.4965928123917));
#52749=CARTESIAN_POINT('Ctrl Pts',(3.56182601680279,-3.80692973983718,49.5495130664736));
#52750=CARTESIAN_POINT('Ctrl Pts',(4.67277672359291,-2.31181234304998,49.6024333205556));
#52751=CARTESIAN_POINT('Ctrl Pts',(4.90148676195955,-0.692117586080884,
49.6553535746375));
#52752=CARTESIAN_POINT('Ctrl Pts',(5.13019680032621,0.927577170888348,49.7082738287195));
#52753=CARTESIAN_POINT('Ctrl Pts',(4.47666617026921,2.67184928803957,49.7611940828015));
#52754=CARTESIAN_POINT('Ctrl Pts',(3.23996046927922,3.7424932048215,49.8141143368834));
#52755=CARTESIAN_POINT('Ctrl Pts',(2.00325476828929,4.81313712160337,49.8670345909654));
#52756=CARTESIAN_POINT('Ctrl Pts',(0.183373996366374,5.21015283801606,49.9199548450474));
#52757=CARTESIAN_POINT('Ctrl Pts',(-1.38687661076657,4.75185989872763,49.9728750991293));
#52758=CARTESIAN_POINT('Ctrl Pts',(-2.95712721789961,4.29356695943917,50.0257953532113));
#52759=CARTESIAN_POINT('Ctrl Pts',(-4.27774766024261,2.97996536444961,50.0787156072932));
#52760=CARTESIAN_POINT('Ctrl Pts',(-4.74440185394119,1.41217926586765,50.1316358613752));
#52761=CARTESIAN_POINT('Ctrl Pts',(-4.87974057311241,0.957491050521679,
50.1469837560312));
#52762=CARTESIAN_POINT('Ctrl Pts',(-4.94325117479429,0.481423074070403,
50.1623316506872));
#52763=CARTESIAN_POINT('Ctrl Pts',(-4.93925722597112,0.00431400617654748,
50.1776795453432));
#52764=CARTESIAN_POINT('Origin',(0.,0.,16.));
#52765=CARTESIAN_POINT('',(-4.9346053643787,-0.00190906406864477,51.3223204546569));
#52766=CARTESIAN_POINT('',(-4.93494424898874,-0.00229539766483815,51.1776795453432));
#52767=CARTESIAN_POINT('',(-4.942,-6.05220448138622E-16,16.));
#52768=CARTESIAN_POINT('Ctrl Pts',(-4.9346053643787,-0.00190906406864477,
51.3223204546569));
#52769=CARTESIAN_POINT('Ctrl Pts',(-4.93132359046474,0.942525285964724,
51.2920113258213));
#52770=CARTESIAN_POINT('Ctrl Pts',(-4.67058264693544,1.88863740917005,51.2617021969857));
#52771=CARTESIAN_POINT('Ctrl Pts',(-4.16399066183724,2.67671072463696,51.2313930681501));
#52772=CARTESIAN_POINT('Ctrl Pts',(-3.27947244580022,4.05270012756452,51.1784728140682));
#52773=CARTESIAN_POINT('Ctrl Pts',(-1.64545880455478,4.94689631680689,51.1255525599862));
#52774=CARTESIAN_POINT('Ctrl Pts',(-0.00969933613304136,4.95010145937766,
51.0726323059043));
#52775=CARTESIAN_POINT('Ctrl Pts',(1.62606013228874,4.95330660194842,51.0197120518223));
#52776=CARTESIAN_POINT('Ctrl Pts',(3.26356542788682,4.06552069784751,50.9667917977403));
#52777=CARTESIAN_POINT('Ctrl Pts',(4.15346911827026,2.69300813567829,50.9138715436584));
#52778=CARTESIAN_POINT('Ctrl Pts',(5.04337280865373,1.32049557350902,50.8609512895764));
#52779=CARTESIAN_POINT('Ctrl Pts',(5.18567489382252,-0.536743646728604,
50.8080310354945));
#52780=CARTESIAN_POINT('Ctrl Pts',(4.5152557662665,-2.0288084927985,50.7551107814125));
#52781=CARTESIAN_POINT('Ctrl Pts',(3.8448366387105,-3.52087333886836,50.7021905273305));
#52782=CARTESIAN_POINT('Ctrl Pts',(2.36169629842972,-4.64776381077051,50.6492702732485));
#52783=CARTESIAN_POINT('Ctrl Pts',(0.74454241669244,-4.89379761790371,50.5963500191666));
#52784=CARTESIAN_POINT('Ctrl Pts',(-0.872611465044887,-5.13983142503691,
50.5434297650846));
#52785=CARTESIAN_POINT('Ctrl Pts',(-2.62377888823873,-4.50500856740112,
50.4905095110027));
#52786=CARTESIAN_POINT('Ctrl Pts',(-3.70759889498285,-3.27983368010881,
50.4375892569207));
#52787=CARTESIAN_POINT('Ctrl Pts',(-4.49451017129344,-2.39029120233235,
50.3991663228328));
#52788=CARTESIAN_POINT('Ctrl Pts',(-4.92962682740573,-1.18954250282331,
50.3607433887448));
#52789=CARTESIAN_POINT('Ctrl Pts',(-4.94000433004934,0.00442567287284368,
50.3223204546569));
#52790=CARTESIAN_POINT('Ctrl Pts',(-4.93925722597112,0.00431400617654748,
50.1776795453432));
#52791=CARTESIAN_POINT('Ctrl Pts',(-4.92947985362941,-1.16367116612706,
50.2152519047692));
#52792=CARTESIAN_POINT('Ctrl Pts',(-4.51515233090316,-2.33789552818176,
50.2528242641951));
#52793=CARTESIAN_POINT('Ctrl Pts',(-3.75970560074729,-3.21997096669155,
50.2903966236211));
#52794=CARTESIAN_POINT('Ctrl Pts',(-2.69566720880064,-4.46236449849485,
50.3433168777031));
#52795=CARTESIAN_POINT('Ctrl Pts',(-0.95490247985317,-5.12518095992721,
50.396237131785));
#52796=CARTESIAN_POINT('Ctrl Pts',(0.665988059953313,-4.90510541524102,
50.449157385867));
#52797=CARTESIAN_POINT('Ctrl Pts',(2.28687859975984,-4.68502987055481,50.5020776399489));
#52798=CARTESIAN_POINT('Ctrl Pts',(3.78789495042532,-3.58206231974999,50.5549978940309));
#52799=CARTESIAN_POINT('Ctrl Pts',(4.48214910531455,-2.10093755936608,50.6079181481129));
#52800=CARTESIAN_POINT('Ctrl Pts',(5.17640326020376,-0.619812798982218,
50.6608384021949));
#52801=CARTESIAN_POINT('Ctrl Pts',(5.06389521931669,1.2394691709808,50.7137586562768));
#52802=CARTESIAN_POINT('Ctrl Pts',(4.19611038046471,2.62607252481409,50.7666789103588));
#52803=CARTESIAN_POINT('Ctrl Pts',(3.32832554161272,4.01267587864738,50.8195991644407));
#52804=CARTESIAN_POINT('Ctrl Pts',(1.70526390479588,4.92660061635104,50.8725194185227));
#52805=CARTESIAN_POINT('Ctrl Pts',(0.0696632635531223,4.94962081985461,
50.9254396726047));
#52806=CARTESIAN_POINT('Ctrl Pts',(-1.56593737768968,4.97264102335818,50.9783599266866));
#52807=CARTESIAN_POINT('Ctrl Pts',(-3.21407702335836,4.1047566926616,51.0312801807686));
#52808=CARTESIAN_POINT('Ctrl Pts',(-4.12054180005445,2.74312495242765,51.0842004348505));
#52809=CARTESIAN_POINT('Ctrl Pts',(-4.65427267801061,1.94138954819395,51.1153601383481));
#52810=CARTESIAN_POINT('Ctrl Pts',(-4.93087142137606,0.968476272531438,
51.1465198418457));
#52811=CARTESIAN_POINT('Ctrl Pts',(-4.93494424898874,-0.00229539766483815,
51.1776795453432));
#52812=CARTESIAN_POINT('Origin',(0.,0.,16.));
#52813=CARTESIAN_POINT('',(-4.94698954266231,-0.00340802453188072,52.3223204546568));
#52814=CARTESIAN_POINT('',(-4.94764183754834,-0.00307943510729547,52.1776795453432));
#52815=CARTESIAN_POINT('',(-4.942,-6.05220448138622E-16,16.));
#52816=CARTESIAN_POINT('Ctrl Pts',(-4.94698954266231,-0.00340802453188072,
52.3223204546568));
#52817=CARTESIAN_POINT('Ctrl Pts',(-4.93574079437759,1.42456851634609,52.2761995169797));
#52818=CARTESIAN_POINT('Ctrl Pts',(-4.28342182577614,2.86150661417242,52.2300785793026));
#52819=CARTESIAN_POINT('Ctrl Pts',(-3.19438680274345,3.78146684366169,52.1839576416255));
#52820=CARTESIAN_POINT('Ctrl Pts',(-1.94480227507184,4.83705095668842,52.1310373875436));
#52821=CARTESIAN_POINT('Ctrl Pts',(-0.120245685876333,5.21199182863453,
52.0781171334615));
#52822=CARTESIAN_POINT('Ctrl Pts',(1.44433800372382,4.73471079013843,52.0251968793796));
#52823=CARTESIAN_POINT('Ctrl Pts',(3.00892169332389,4.25742975164236,51.9722766252976));
#52824=CARTESIAN_POINT('Ctrl Pts',(4.31353248332859,2.92792680270421,51.9193563712157));
#52825=CARTESIAN_POINT('Ctrl Pts',(4.7611605513041,1.3546027978562,51.8664361171337));
#52826=CARTESIAN_POINT('Ctrl Pts',(5.20878861927959,-0.218721206991761,
51.8135158630518));
#52827=CARTESIAN_POINT('Ctrl Pts',(4.79943396522586,-2.03586626774964,51.7605956089698));
#52828=CARTESIAN_POINT('Ctrl Pts',(3.72042353078829,-3.26527905190521,51.7076753548878));
#52829=CARTESIAN_POINT('Ctrl Pts',(2.64141309635066,-4.49469183606084,51.6547551008059));
#52830=CARTESIAN_POINT('Ctrl Pts',(0.892746881529132,-5.1363723436142,51.6018348467239));
#52831=CARTESIAN_POINT('Ctrl Pts',(-0.725358746921474,-4.8966777741157,
51.5489145926419));
#52832=CARTESIAN_POINT('Ctrl Pts',(-2.34346437537199,-4.65698320461722,
51.49599433856));
#52833=CARTESIAN_POINT('Ctrl Pts',(-3.83100941745154,-3.535913558067,51.443074084478));
#52834=CARTESIAN_POINT('Ctrl Pts',(-4.50727054307715,-2.04648742648548,
51.3901538303961));
#52835=CARTESIAN_POINT('Ctrl Pts',(-4.79621520662888,-1.41010346743882,
51.3675427051497));
#52836=CARTESIAN_POINT('Ctrl Pts',(-4.93705362349566,-0.70647314083382,
51.3449315799033));
#52837=CARTESIAN_POINT('Ctrl Pts',(-4.9346053643787,-0.00190906406864477,
51.3223204546569));
#52838=CARTESIAN_POINT('Ctrl Pts',(-4.93494424898874,-0.00229539766483815,
51.1776795453432));
#52839=CARTESIAN_POINT('Ctrl Pts',(-4.9377885305877,-0.680239141156077,
51.1994400959276));
#52840=CARTESIAN_POINT('Ctrl Pts',(-4.80772180958983,-1.35713842276963,
51.221200646512));
#52841=CARTESIAN_POINT('Ctrl Pts',(-4.53950114466406,-1.9739626613036,51.2429611970964));
#52842=CARTESIAN_POINT('Ctrl Pts',(-3.88720580485411,-3.47403938502989,
51.2958814511784));
#52843=CARTESIAN_POINT('Ctrl Pts',(-2.41782521751062,-4.61881368271118,
51.3488017052603));
#52844=CARTESIAN_POINT('Ctrl Pts',(-0.803770380809228,-4.88441935193539,
51.4017219593423));
#52845=CARTESIAN_POINT('Ctrl Pts',(0.810284455892164,-5.1500250211596,51.4546422134243));
#52846=CARTESIAN_POINT('Ctrl Pts',(2.56901354195146,-4.53646206192671,51.5075624675063));
#52847=CARTESIAN_POINT('Ctrl Pts',(3.6675955870482,-3.32450625514402,51.5604827215882));
#52848=CARTESIAN_POINT('Ctrl Pts',(4.7661776321449,-2.11255044836137,51.6134029756702));
#52849=CARTESIAN_POINT('Ctrl Pts',(5.20461263627908,-0.302201794028944,
51.6663232297521));
#52850=CARTESIAN_POINT('Ctrl Pts',(4.78226604547315,1.27809651472091,51.7192434838341));
#52851=CARTESIAN_POINT('Ctrl Pts',(4.3599194546672,2.85839482347081,51.7721637379161));
#52852=CARTESIAN_POINT('Ctrl Pts',(3.07679126892111,4.20864278663813,51.825083991998));
#52853=CARTESIAN_POINT('Ctrl Pts',(1.52006054286266,4.71094631434696,51.87800424608));
#52854=CARTESIAN_POINT('Ctrl Pts',(-0.0366701831957017,5.21324984205576,
51.930924500162));
#52855=CARTESIAN_POINT('Ctrl Pts',(-1.86700344956638,4.86760893430616,51.9838447542439));
#52856=CARTESIAN_POINT('Ctrl Pts',(-3.13335079942941,3.83219414935389,52.0367650083259));
#52857=CARTESIAN_POINT('Ctrl Pts',(-4.25734861844162,2.9131698704424,52.083736520665));
#52858=CARTESIAN_POINT('Ctrl Pts',(-4.93702884968978,1.45073013335928,52.1307080330041));
#52859=CARTESIAN_POINT('Ctrl Pts',(-4.94764183754834,-0.00307943510729547,
52.1776795453432));
#52860=CARTESIAN_POINT('Origin',(0.,0.,16.));
#52861=CARTESIAN_POINT('',(-4.94509673752737,0.0040742516207555,53.3223204546569));
#52862=CARTESIAN_POINT('',(-4.94431829400652,0.00425244366110885,53.1776795453432));
#52863=CARTESIAN_POINT('',(-4.942,-6.05220448138622E-16,16.));
#52864=CARTESIAN_POINT('Ctrl Pts',(-4.94509673752737,0.0040742516207555,
53.3223204546569));
#52865=CARTESIAN_POINT('Ctrl Pts',(-4.94757864022345,0.283393084706415,
53.3133079622201));
#52866=CARTESIAN_POINT('Ctrl Pts',(-4.92595073565188,0.562327591030859,
53.3042954697834));
#52867=CARTESIAN_POINT('Ctrl Pts',(-4.87885318126865,0.836893165749963,
53.2952829773467));
#52868=CARTESIAN_POINT('Ctrl Pts',(-4.60230209819144,2.44910866310731,53.2423627232647));
#52869=CARTESIAN_POINT('Ctrl Pts',(-3.44758426677398,3.91068799192893,53.1894424691828));
#52870=CARTESIAN_POINT('Ctrl Pts',(-1.94311620233063,4.55279012908506,53.1365222151008));
#52871=CARTESIAN_POINT('Ctrl Pts',(-0.438648137887247,5.19489226624121,
53.0836019610189));
#52872=CARTESIAN_POINT('Ctrl Pts',(1.4155701595821,5.01751721173186,53.0306817069369));
#52873=CARTESIAN_POINT('Ctrl Pts',(2.77102007823768,4.10183449949628,52.9777614528549));
#52874=CARTESIAN_POINT('Ctrl Pts',(4.12646999689325,3.1861517872607,52.924841198773));
#52875=CARTESIAN_POINT('Ctrl Pts',(4.98315153673507,1.53216141729899,52.871920944691));
#52876=CARTESIAN_POINT('Ctrl Pts',(4.9490341412924,-0.10324535619766,52.8190006906091));
#52877=CARTESIAN_POINT('Ctrl Pts',(4.91491674584974,-1.73865212969422,52.7660804365271));
#52878=CARTESIAN_POINT('Ctrl Pts',(3.99000041512261,-3.35547530672568,52.7131601824451));
#52879=CARTESIAN_POINT('Ctrl Pts',(2.59754098802034,-4.21383190822896,52.6602399283632));
#52880=CARTESIAN_POINT('Ctrl Pts',(1.205081560918,-5.07218850973229,52.6073196742812));
#52881=CARTESIAN_POINT('Ctrl Pts',(-0.654920962559591,-5.17207853570735,
52.5543994201993));
#52882=CARTESIAN_POINT('Ctrl Pts',(-2.13130102041059,-4.4677907846777,52.5014791661173));
#52883=CARTESIAN_POINT('Ctrl Pts',(-3.6076810782616,-3.76350303364805,52.4485589120353));
#52884=CARTESIAN_POINT('Ctrl Pts',(-4.70043867048604,-2.25503750561363,
52.3956386579533));
#52885=CARTESIAN_POINT('Ctrl Pts',(-4.90951123352436,-0.632691064542821,
52.3427184038713));
#52886=CARTESIAN_POINT('Ctrl Pts',(-4.93637335904372,-0.424248248792036,
52.3359190874665));
#52887=CARTESIAN_POINT('Ctrl Pts',(-4.94864787405361,-0.213925520686765,
52.3291197710617));
#52888=CARTESIAN_POINT('Ctrl Pts',(-4.94698954266231,-0.00340802453188072,
52.3223204546568));
#52889=CARTESIAN_POINT('Ctrl Pts',(-4.94764183754834,-0.00307943510729547,
52.1776795453432));
#52890=CARTESIAN_POINT('Ctrl Pts',(-4.94898592720496,-0.187198217650565,
52.1836282870861));
#52891=CARTESIAN_POINT('Ctrl Pts',(-4.93959875206843,-0.371178579690442,
52.1895770288289));
#52892=CARTESIAN_POINT('Ctrl Pts',(-4.91902378063747,-0.553899157022463,
52.1955257705718));
#52893=CARTESIAN_POINT('Ctrl Pts',(-4.73598797862701,-2.17938901629118,
52.2484460246538));
#52894=CARTESIAN_POINT('Ctrl Pts',(-3.66755494125079,-3.70518007267354,
52.3013662787357));
#52895=CARTESIAN_POINT('Ctrl Pts',(-2.2026559442682,-4.43304703582165,52.3542865328177));
#52896=CARTESIAN_POINT('Ctrl Pts',(-0.737756947285612,-5.16091399896976,
52.4072067868996));
#52897=CARTESIAN_POINT('Ctrl Pts',(1.12360800930335,-5.09085686888362,52.4601270409816));
#52898=CARTESIAN_POINT('Ctrl Pts',(2.52964989329714,-4.2549348582521,52.5130472950635));
#52899=CARTESIAN_POINT('Ctrl Pts',(3.93569177729098,-3.41901284762056,52.5659675491455));
#52900=CARTESIAN_POINT('Ctrl Pts',(4.88641058868961,-1.81722595644361,52.6188878032275));
#52901=CARTESIAN_POINT('Ctrl Pts',(4.94674287935491,-0.182576329732651,
52.6718080573094));
#52902=CARTESIAN_POINT('Ctrl Pts',(5.0070751700202,1.45207329697826,52.7247283113914));
#52903=CARTESIAN_POINT('Ctrl Pts',(4.17702093995222,3.11958565922317,52.7776485654734));
#52904=CARTESIAN_POINT('Ctrl Pts',(2.83642568199835,4.05688163262466,52.8305688195553));
#52905=CARTESIAN_POINT('Ctrl Pts',(1.49583042404448,4.99417760602615,52.8834890736373));
#52906=CARTESIAN_POINT('Ctrl Pts',(-0.355305861795278,5.20125719058422,
52.9364093277193));
#52907=CARTESIAN_POINT('Ctrl Pts',(-1.86987493927361,4.58335760574097,52.9893295818012));
#52908=CARTESIAN_POINT('Ctrl Pts',(-3.384444016752,3.9654580208977,53.0422498358832));
#52909=CARTESIAN_POINT('Ctrl Pts',(-4.56244588586893,2.52257926665306,53.0951700899651));
#52910=CARTESIAN_POINT('Ctrl Pts',(-4.86480890004871,0.915004697602124,
53.1480903440471));
#52911=CARTESIAN_POINT('Ctrl Pts',(-4.92116211960056,0.615391324314909,
53.1579534111458));
#52912=CARTESIAN_POINT('Ctrl Pts',(-4.94709912492537,0.310057072885753,
53.1678164782445));
#52913=CARTESIAN_POINT('Ctrl Pts',(-4.94431829400652,0.00425244366110885,
53.1776795453432));
#52914=CARTESIAN_POINT('Origin',(0.,0.,16.));
#52915=CARTESIAN_POINT('',(-4.93403082595878,0.000832190755156725,54.3223204546569));
#52916=CARTESIAN_POINT('',(-4.93393232083006,0.000401187422265207,54.1776795453432));
#52917=CARTESIAN_POINT('',(-4.942,-6.05220448138622E-16,16.));
#52918=CARTESIAN_POINT('Ctrl Pts',(-4.93403082595878,0.000832190755156725,
54.3223204546569));
#52919=CARTESIAN_POINT('Ctrl Pts',(-4.93519480376781,0.77458390453562,54.2974961533786));
#52920=CARTESIAN_POINT('Ctrl Pts',(-4.76408859627892,1.54784860488958,54.2726718521003));
#52921=CARTESIAN_POINT('Ctrl Pts',(-4.41799967623941,2.23268389970517,54.2478475508221));
#52922=CARTESIAN_POINT('Ctrl Pts',(-3.6802099846732,3.69261050145239,54.1949272967401));
#52923=CARTESIAN_POINT('Ctrl Pts',(-2.14720464186602,4.75066627671043,54.1420070426582));
#52924=CARTESIAN_POINT('Ctrl Pts',(-0.52051030581542,4.92266874335397,54.0890867885762));
#52925=CARTESIAN_POINT('Ctrl Pts',(1.10618403023518,5.0946712099975,54.0361665344942));
#52926=CARTESIAN_POINT('Ctrl Pts',(2.82656735952921,4.38062036802653,53.9832462804122));
#52927=CARTESIAN_POINT('Ctrl Pts',(3.85336599568517,3.10727678821045,53.9303260263302));
#52928=CARTESIAN_POINT('Ctrl Pts',(4.8801646318411,1.83393320839441,53.8774057722483));
#52929=CARTESIAN_POINT('Ctrl Pts',(5.21337857485901,0.00129689073330608,
53.8244855181664));
#52930=CARTESIAN_POINT('Ctrl Pts',(4.70052403533771,-1.55198979650856,53.7715652640844));
#52931=CARTESIAN_POINT('Ctrl Pts',(4.18766949581641,-3.10527648375042,53.7186450100024));
#52932=CARTESIAN_POINT('Ctrl Pts',(2.82874647375599,-4.37921354057296,53.6657247559204));
#52933=CARTESIAN_POINT('Ctrl Pts',(1.24561889847324,-4.79082791331733,53.6128045018385));
#52934=CARTESIAN_POINT('Ctrl Pts',(-0.337508676809509,-5.2024422860617,
53.5598842477565));
#52935=CARTESIAN_POINT('Ctrl Pts',(-2.14484080531469,-4.75173397472772,
53.5069639936746));
#52936=CARTESIAN_POINT('Ctrl Pts',(-3.34931470219873,-3.64495398611418,
53.4540437395926));
#52937=CARTESIAN_POINT('Ctrl Pts',(-4.34866275314335,-2.72666225118592,
53.4101359779474));
#52938=CARTESIAN_POINT('Ctrl Pts',(-4.93300521093011,-1.35673296483636,
53.3662282163021));
#52939=CARTESIAN_POINT('Ctrl Pts',(-4.94509673752737,0.0040742516207555,
53.3223204546569));
#52940=CARTESIAN_POINT('Ctrl Pts',(-4.94431829400652,0.00425244366110885,
53.1776795453432));
#52941=CARTESIAN_POINT('Ctrl Pts',(-4.93217858577541,-1.33073665953657,
53.2207367323265));
#52942=CARTESIAN_POINT('Ctrl Pts',(-4.37274694612505,-2.67469001651735,
53.2637939193098));
#52943=CARTESIAN_POINT('Ctrl Pts',(-3.4073211579765,-3.59078845896452,53.306851106293));
#52944=CARTESIAN_POINT('Ctrl Pts',(-2.22074624248181,-4.71673666262315,
53.359771360375));
#52945=CARTESIAN_POINT('Ctrl Pts',(-0.42087225224974,-5.19636268608309,
53.4126916144569));
#52946=CARTESIAN_POINT('Ctrl Pts',(1.16865098585596,-4.81018233582522,53.4656118685389));
#52947=CARTESIAN_POINT('Ctrl Pts',(2.75817422396157,-4.42400198556738,53.5185321226208));
#52948=CARTESIAN_POINT('Ctrl Pts',(4.13734670994089,-3.17201526159183,53.5714523767028));
#52949=CARTESIAN_POINT('Ctrl Pts',(4.6750380505237,-1.62715041000601,53.6243726307848));
#52950=CARTESIAN_POINT('Ctrl Pts',(5.2127293911065,-0.0822855584201898,
53.6772928848668));
#52951=CARTESIAN_POINT('Ctrl Pts',(4.90893958629287,1.75545742077581,53.7302131389487));
#52952=CARTESIAN_POINT('Ctrl Pts',(3.9026874904557,3.045099273007,53.7831333930307));
#52953=CARTESIAN_POINT('Ctrl Pts',(2.89643539461849,4.33474112523822,53.8360536471126));
#52954=CARTESIAN_POINT('Ctrl Pts',(1.18772100775765,5.0762818505045,53.8889739011946));
#52955=CARTESIAN_POINT('Ctrl Pts',(-0.441521870018959,4.93038108759577,
53.9418941552766));
#52956=CARTESIAN_POINT('Ctrl Pts',(-2.07076474779552,4.78448032468705,53.9948144093585));
#52957=CARTESIAN_POINT('Ctrl Pts',(-3.62053611648792,3.75113807360336,54.0477346634405));
#52958=CARTESIAN_POINT('Ctrl Pts',(-4.38163692859106,2.30322753036564,54.1006549175225));
#52959=CARTESIAN_POINT('Ctrl Pts',(-4.75089382782116,1.60075691273335,54.1263297934627));
#52960=CARTESIAN_POINT('Ctrl Pts',(-4.9345120375631,0.800704467282281,54.152004669403));
#52961=CARTESIAN_POINT('Ctrl Pts',(-4.93393232083006,0.000401187422265207,
54.1776795453432));
#52962=CARTESIAN_POINT('Origin',(0.,0.,16.));
#52963=CARTESIAN_POINT('',(-4.94204396072975,-0.00451108372972908,55.3223204546568));
#52964=CARTESIAN_POINT('',(-4.94284599866247,-0.00446247280752122,55.1776795453432));
#52965=CARTESIAN_POINT('',(-4.942,-6.05220448138622E-16,16.));
#52966=CARTESIAN_POINT('Ctrl Pts',(-4.94204396072975,-0.00451108372972908,
55.3223204546568));
#52967=CARTESIAN_POINT('Ctrl Pts',(-4.93045565886636,1.25690241555476,55.281684344537));
#52968=CARTESIAN_POINT('Ctrl Pts',(-4.43833582829864,2.52635331123123,55.2410482344173));
#52969=CARTESIAN_POINT('Ctrl Pts',(-3.56758671933519,3.43160655309978,55.2004121242975));
#52970=CARTESIAN_POINT('Ctrl Pts',(-2.43361341450575,4.61051446104039,55.1474918702155));
#52971=CARTESIAN_POINT('Ctrl Pts',(-0.65749411504605,5.17175205664432,55.0945716161334));
#52972=CARTESIAN_POINT('Ctrl Pts',(0.947991861475882,4.85848844455039,55.0416513620514));
#52973=CARTESIAN_POINT('Ctrl Pts',(2.55347783799768,4.54522483245649,54.9887311079695));
#52974=CARTESIAN_POINT('Ctrl Pts',(3.98833049158174,3.35746001266491,54.9358108538876));
#52975=CARTESIAN_POINT('Ctrl Pts',(4.59593933387555,1.83873330708663,54.8828905998056));
#52976=CARTESIAN_POINT('Ctrl Pts',(5.2035481761694,0.320006601508274,54.8299703457237));
#52977=CARTESIAN_POINT('Ctrl Pts',(4.98391320717291,-1.52968198985681,54.7770500916417));
#52978=CARTESIAN_POINT('Ctrl Pts',(4.0375427431176,-2.86388671786309,54.7241298375597));
#52979=CARTESIAN_POINT('Ctrl Pts',(3.09117227906232,-4.19809144586933,54.6712095834777));
#52980=CARTESIAN_POINT('Ctrl Pts',(1.41806631994828,-5.0168123105168,54.6182893293958));
#52981=CARTESIAN_POINT('Ctrl Pts',(-0.216136294490469,-4.94539014006561,
54.5653690753138));
#52982=CARTESIAN_POINT('Ctrl Pts',(-1.85033890892918,-4.87396796961441,
54.5124488212319));
#52983=CARTESIAN_POINT('Ctrl Pts',(-3.4456381786926,-3.91240276406461,54.4595285671499));
#52984=CARTESIAN_POINT('Ctrl Pts',(-4.27200079341172,-2.50072144717157,
54.4066083130679));
#52985=CARTESIAN_POINT('Ctrl Pts',(-4.7107259171786,-1.75124409976784,54.3785123602642));
#52986=CARTESIAN_POINT('Ctrl Pts',(-4.93271344484821,-0.874894033659396,
54.3504164074605));
#52987=CARTESIAN_POINT('Ctrl Pts',(-4.93403082595878,0.000832190755156725,
54.3223204546569));
#52988=CARTESIAN_POINT('Ctrl Pts',(-4.93393232083006,0.000401187422265207,
54.1776795453432));
#52989=CARTESIAN_POINT('Ctrl Pts',(-4.93331714350093,-0.848855710199169,
54.2049249234849));
#52990=CARTESIAN_POINT('Ctrl Pts',(-4.72528049547278,-1.69839506725433,
54.2321703016266));
#52991=CARTESIAN_POINT('Ctrl Pts',(-4.31154403127411,-2.43191021565593,
54.2594156797684));
#52992=CARTESIAN_POINT('Ctrl Pts',(-3.50792006634005,-3.85665858304818,
54.3123359338503));
#52993=CARTESIAN_POINT('Ctrl Pts',(-1.92824188095795,-4.8436764824408,54.3652561879323));
#52994=CARTESIAN_POINT('Ctrl Pts',(-0.295394338707872,-4.9412894486446,
54.4181764420142));
#52995=CARTESIAN_POINT('Ctrl Pts',(1.33745320354216,-5.0389024148484,54.4710966960962));
#52996=CARTESIAN_POINT('Ctrl Pts',(3.02347010266025,-4.24711044786332,54.5240169501782));
#52997=CARTESIAN_POINT('Ctrl Pts',(3.99110927558139,-2.92824964458212,54.5769372042601));
#52998=CARTESIAN_POINT('Ctrl Pts',(4.95874844850256,-1.60938884130088,54.6298574583421));
#52999=CARTESIAN_POINT('Ctrl Pts',(5.20800989522687,0.236540798276539,54.6827777124241));
#53000=CARTESIAN_POINT('Ctrl Pts',(4.62482777083827,1.76481367875202,54.735697966506));
#53001=CARTESIAN_POINT('Ctrl Pts',(4.04164564644968,3.29308655922746,54.788618220588));
#53002=CARTESIAN_POINT('Ctrl Pts',(2.62601995094824,4.50370268060093,54.8415384746699));
#53003=CARTESIAN_POINT('Ctrl Pts',(1.02576262302031,4.84266561635652,54.8944587287519));
#53004=CARTESIAN_POINT('Ctrl Pts',(-0.574494704907621,5.1816285521121,54.9473789828339));
#53005=CARTESIAN_POINT('Ctrl Pts',(-2.35938366526199,4.64893830224978,55.0002992369159));
#53006=CARTESIAN_POINT('Ctrl Pts',(-3.51211180971311,3.48836206072432,55.0532194909978));
#53007=CARTESIAN_POINT('Ctrl Pts',(-4.4157898059278,2.57853157081683,55.0947061757796));
#53008=CARTESIAN_POINT('Ctrl Pts',(-4.93095870305679,1.2828191742603,55.1361928605614));
#53009=CARTESIAN_POINT('Ctrl Pts',(-4.94284599866247,-0.00446247280752122,
55.1776795453432));
#53010=CARTESIAN_POINT('Origin',(0.,0.,16.));
#53011=CARTESIAN_POINT('',(-4.94916162572937,0.00195780085970945,56.3223204546569));
#53012=CARTESIAN_POINT('',(-4.9486927940556,0.00238008058365034,56.1776795453432));
#53013=CARTESIAN_POINT('',(-4.942,-6.05220448138622E-16,16.));
#53014=CARTESIAN_POINT('Ctrl Pts',(-4.94916162572937,0.00195780085970945,
56.3223204546569));
#53015=CARTESIAN_POINT('Ctrl Pts',(-4.94971144692239,0.111053665337975,
56.3187927897774));
#53016=CARTESIAN_POINT('Ctrl Pts',(-4.94641661384693,0.220115719674017,
56.315265124898));
#53017=CARTESIAN_POINT('Ctrl Pts',(-4.93917135292333,0.328914702796541,
56.3117374600186));
#53018=CARTESIAN_POINT('Ctrl Pts',(-4.83048159296228,1.96106232098248,56.2588172059367));
#53019=CARTESIAN_POINT('Ctrl Pts',(-3.83276814539685,3.53400710106189,56.2058969518547));
#53020=CARTESIAN_POINT('Ctrl Pts',(-2.40259992160997,4.32794548855851,56.1529766977728));
#53021=CARTESIAN_POINT('Ctrl Pts',(-0.972431697823093,5.12188387605513,
56.1000564436908));
#53022=CARTESIAN_POINT('Ctrl Pts',(0.890191302185183,5.13681587096895,56.0471361896088));
#53023=CARTESIAN_POINT('Ctrl Pts',(2.33290434633096,4.36590836437554,55.9942159355269));
#53024=CARTESIAN_POINT('Ctrl Pts',(3.77561739047674,3.59500085778213,55.9412956814449));
#53025=CARTESIAN_POINT('Ctrl Pts',(4.79842047875997,2.03825384968152,55.8883754273629));
#53026=CARTESIAN_POINT('Ctrl Pts',(4.93326329701873,0.408058546708748,55.8354551732809));
#53027=CARTESIAN_POINT('Ctrl Pts',(5.0681061152775,-1.22213675626403,55.782534919199));
#53028=CARTESIAN_POINT('Ctrl Pts',(4.31498866351168,-2.92578035410902,55.729614665117));
#53029=CARTESIAN_POINT('Ctrl Pts',(3.01854898978546,-3.92325891721657,55.6766944110351));
#53030=CARTESIAN_POINT('Ctrl Pts',(1.72210931605921,-4.92073748032415,55.6237741569531));
#53031=CARTESIAN_POINT('Ctrl Pts',(-0.117652579627481,-5.21205100869435,
55.5708539028712));
#53032=CARTESIAN_POINT('Ctrl Pts',(-1.65883355567899,-4.66388998260118,
55.5179336487892));
#53033=CARTESIAN_POINT('Ctrl Pts',(-3.20001453173045,-4.11572895650802,
55.4650133947072));
#53034=CARTESIAN_POINT('Ctrl Pts',(-4.4426145881467,-2.72809337595155,55.4120931406252));
#53035=CARTESIAN_POINT('Ctrl Pts',(-4.81800096125524,-1.13598647553473,
55.3591728865432));
#53036=CARTESIAN_POINT('Ctrl Pts',(-4.90513773579808,-0.766417759225417,
55.3468887425811));
#53037=CARTESIAN_POINT('Ctrl Pts',(-4.94554706100059,-0.385831662281748,
55.334604598619));
#53038=CARTESIAN_POINT('Ctrl Pts',(-4.94204396072975,-0.00451108372972908,
55.3223204546568));
#53039=CARTESIAN_POINT('Ctrl Pts',(-4.94284599866247,-0.00446247280752122,
55.1776795453432));
#53040=CARTESIAN_POINT('Ctrl Pts',(-4.94612209119225,-0.359232298306442,
55.1891131146434));
#53041=CARTESIAN_POINT('Ctrl Pts',(-4.91117232521921,-0.713361781229651,
55.2005466839435));
#53042=CARTESIAN_POINT('Ctrl Pts',(-4.83559423534505,-1.05859700628939,
55.2119802532437));
#53043=CARTESIAN_POINT('Ctrl Pts',(-4.48578118797803,-2.6565175985889,55.2649005073256));
#53044=CARTESIAN_POINT('Ctrl Pts',(-3.26558776469621,-4.06389654999934,
55.3178207614076));
#53045=CARTESIAN_POINT('Ctrl Pts',(-1.73339311164005,-4.63669575788038,
55.3707410154896));
#53046=CARTESIAN_POINT('Ctrl Pts',(-0.201198458583838,-5.20949496576144,
55.4236612695715));
#53047=CARTESIAN_POINT('Ctrl Pts',(1.64299742424673,-4.94771443011306,55.4765815236535));
#53048=CARTESIAN_POINT('Ctrl Pts',(2.95526233502001,-3.97114892214321,55.5295017777355));
#53049=CARTESIAN_POINT('Ctrl Pts',(4.26752724579325,-2.9945834141734,55.5824220318174));
#53050=CARTESIAN_POINT('Ctrl Pts',(5.04786118450924,-1.30323293388218,55.6353422858994));
#53051=CARTESIAN_POINT('Ctrl Pts',(4.93917142300628,0.328914707462642,55.6882625399813));
#53052=CARTESIAN_POINT('Ctrl Pts',(4.83048166150332,1.96106234880747,55.7411827940633));
#53053=CARTESIAN_POINT('Ctrl Pts',(3.83276819978142,3.5340071512059,55.7941030481453));
#53054=CARTESIAN_POINT('Ctrl Pts',(2.40259995570176,4.32794554996814,55.8470233022272));
#53055=CARTESIAN_POINT('Ctrl Pts',(0.972431711622098,5.12188394873038,55.8999435563092));
#53056=CARTESIAN_POINT('Ctrl Pts',(-0.890191314815322,5.13681594385641,
55.9528638103912));
#53057=CARTESIAN_POINT('Ctrl Pts',(-2.33290437943218,4.36590842632473,56.0057840644731));
#53058=CARTESIAN_POINT('Ctrl Pts',(-3.77561744404904,3.59500090879304,56.0587043185551));
#53059=CARTESIAN_POINT('Ctrl Pts',(-4.79842054684533,2.03825387860361,56.1116245726371));
#53060=CARTESIAN_POINT('Ctrl Pts',(-4.93326336701772,0.408058552499706,
56.164544826719));
#53061=CARTESIAN_POINT('Ctrl Pts',(-4.94441928789138,0.273187967299986,
56.1689230662604));
#53062=CARTESIAN_POINT('Ctrl Pts',(-4.94949737612309,0.137814649647994,
56.1733013058018));
#53063=CARTESIAN_POINT('Ctrl Pts',(-4.9486927940556,0.00238008058365034,
56.1776795453432));
#53064=CARTESIAN_POINT('Origin',(0.,0.,16.));
#53065=CARTESIAN_POINT('',(-4.93623902664834,0.00326946414225537,57.3223204546569));
#53066=CARTESIAN_POINT('',(-4.93573111423024,0.00295138605979709,57.1776795453432));
#53067=CARTESIAN_POINT('',(-4.942,-6.05220448138622E-16,16.));
#53068=CARTESIAN_POINT('Ctrl Pts',(-4.93623902664834,0.00326946414225537,
57.3223204546569));
#53069=CARTESIAN_POINT('Ctrl Pts',(-4.93989713650663,0.605389273547052,
57.3029809809359));
#53070=CARTESIAN_POINT('Ctrl Pts',(-4.83794904041642,1.20631307007342,57.2836415072149));
#53071=CARTESIAN_POINT('Ctrl Pts',(-4.62482770521538,1.76481365371148,57.2643020334939));
#53072=CARTESIAN_POINT('Ctrl Pts',(-4.04164558910142,3.29308651250188,57.211381779412));
#53073=CARTESIAN_POINT('Ctrl Pts',(-2.6260199136863,4.50370261669748,57.15846152533));
#53074=CARTESIAN_POINT('Ctrl Pts',(-1.02576260846464,4.84266554764316,57.1055412712481));
#53075=CARTESIAN_POINT('Ctrl Pts',(0.574494696756969,5.18162847858883,57.0526210171661));
#53076=CARTESIAN_POINT('Ctrl Pts',(2.35938363178511,4.64893823628462,56.9997007630841));
#53077=CARTESIAN_POINT('Ctrl Pts',(3.51211175987971,3.48836201122659,56.9467805090022));
#53078=CARTESIAN_POINT('Ctrl Pts',(4.66483988797431,2.32778578616857,56.8938602549202));
#53079=CARTESIAN_POINT('Ctrl Pts',(5.18540720913538,0.539323578356728,56.8409400008383));
#53080=CARTESIAN_POINT('Ctrl Pts',(4.83559416673167,-1.05859699126952,56.7880197467563));
#53081=CARTESIAN_POINT('Ctrl Pts',(4.48578112432795,-2.65651756089581,56.7350994926743));
#53082=CARTESIAN_POINT('Ctrl Pts',(3.26558771835941,-4.0638964923365,56.6821792385924));
#53083=CARTESIAN_POINT('Ctrl Pts',(1.73339308704371,-4.63669569208971,56.6292589845104));
#53084=CARTESIAN_POINT('Ctrl Pts',(0.201198455728012,-5.20949489184292,
56.5763387304284));
#53085=CARTESIAN_POINT('Ctrl Pts',(-1.64299740093485,-4.94771435990864,
56.5234184763465));
#53086=CARTESIAN_POINT('Ctrl Pts',(-2.95526229308795,-3.97114886579523,
56.4704982222645));
#53087=CARTESIAN_POINT('Ctrl Pts',(-4.18005158912286,-3.0596812412178,56.4211056330619));
#53088=CARTESIAN_POINT('Ctrl Pts',(-4.94146330594845,-1.52554761761349,
56.3717130438594));
#53089=CARTESIAN_POINT('Ctrl Pts',(-4.94916162572937,0.00195780085970945,
56.3223204546569));
#53090=CARTESIAN_POINT('Ctrl Pts',(-4.9486927940556,0.00238008058365034,
56.1776795453432));
#53091=CARTESIAN_POINT('Ctrl Pts',(-4.93977230579782,-1.49919761032442,
56.2262215598838));
#53092=CARTESIAN_POINT('Ctrl Pts',(-4.20773066973569,-3.00830456759471,
56.2747635744243));
#53093=CARTESIAN_POINT('Ctrl Pts',(-3.018549032617,-3.92325897288391,56.3233055889649));
#53094=CARTESIAN_POINT('Ctrl Pts',(-1.72210934049551,-4.92073755014514,
56.3762258430469));
#53095=CARTESIAN_POINT('Ctrl Pts',(0.117652581295909,-5.2120510826492,56.4291460971289));
#53096=CARTESIAN_POINT('Ctrl Pts',(1.65883357921563,-4.66389004877836,56.4820663512108));
#53097=CARTESIAN_POINT('Ctrl Pts',(3.2000145771353,-4.11572901490753,56.5349866052928));
#53098=CARTESIAN_POINT('Ctrl Pts',(4.44261465118334,-2.72809341466183,56.5879068593747));
#53099=CARTESIAN_POINT('Ctrl Pts',(4.8180010296186,-1.13598649165438,56.6408271134567));
#53100=CARTESIAN_POINT('Ctrl Pts',(5.19338740805387,0.456120431353115,56.6937473675386));
#53101=CARTESIAN_POINT('Ctrl Pts',(4.70156009087639,2.25269867712231,56.7466676216206));
#53102=CARTESIAN_POINT('Ctrl Pts',(3.56758676995704,3.43160660179086,56.7995878757026));
#53103=CARTESIAN_POINT('Ctrl Pts',(2.43361344903769,4.61051452645941,56.8525081297845));
#53104=CARTESIAN_POINT('Ctrl Pts',(0.65749412437644,5.17175213002719,56.9054283838665));
#53105=CARTESIAN_POINT('Ctrl Pts',(-0.94799187492607,4.85848851348866,56.9583486379485));
#53106=CARTESIAN_POINT('Ctrl Pts',(-2.55347787422853,4.54522489695015,57.0112688920304));
#53107=CARTESIAN_POINT('Ctrl Pts',(-3.98833054817231,3.35746006030537,57.0641891461124));
#53108=CARTESIAN_POINT('Ctrl Pts',(-4.59593939908791,1.83873333317766,57.1171094001944));
#53109=CARTESIAN_POINT('Ctrl Pts',(-4.82775332951413,1.25931120769625,57.1372994485773));
#53110=CARTESIAN_POINT('Ctrl Pts',(-4.93915674573565,0.631715508347176,
57.1574894969603));
#53111=CARTESIAN_POINT('Ctrl Pts',(-4.93573111423024,0.00295138605979709,
57.1776795453432));
#53112=CARTESIAN_POINT('Origin',(0.,0.,16.));
#53113=CARTESIAN_POINT('',(-4.9373129524182,-0.00377529733612325,58.3223204546568));
#53114=CARTESIAN_POINT('',(-4.93796046055574,-0.00400002009900308,58.1776795453432));
#53115=CARTESIAN_POINT('',(-4.942,-6.05220448138622E-16,16.));
#53116=CARTESIAN_POINT('Ctrl Pts',(-4.9373129524182,-0.00377529733612325,
58.3223204546568));
#53117=CARTESIAN_POINT('Ctrl Pts',(-4.92952693668152,1.09003472006405,58.2871691720943));
#53118=CARTESIAN_POINT('Ctrl Pts',(-4.57107143779465,2.18847891881712,58.2520178895318));
#53119=CARTESIAN_POINT('Ctrl Pts',(-3.90268743507911,3.04509922980021,58.2168666069693));
#53120=CARTESIAN_POINT('Ctrl Pts',(-2.89643535351957,4.33474106373227,58.1639463528874));
#53121=CARTESIAN_POINT('Ctrl Pts',(-1.18772099090388,5.07628177847635,58.1110260988054));
#53122=CARTESIAN_POINT('Ctrl Pts',(0.441521863755048,4.93038101763753,58.0581058447234));
#53123=CARTESIAN_POINT('Ctrl Pts',(2.07076471841393,4.78448025679871,58.0051855906414));
#53124=CARTESIAN_POINT('Ctrl Pts',(3.62053606511612,3.75113802037702,57.9522653365595));
#53125=CARTESIAN_POINT('Ctrl Pts',(4.38163686641958,2.30322749768385,57.8993450824775));
#53126=CARTESIAN_POINT('Ctrl Pts',(5.14273766772306,0.855316974990642,57.8464248283956));
#53127=CARTESIAN_POINT('Ctrl Pts',(5.11516792362781,-1.00716183397399,57.7935045743136));
#53128=CARTESIAN_POINT('Ctrl Pts',(4.31154397009623,-2.43191018115001,57.7405843202316));
#53129=CARTESIAN_POINT('Ctrl Pts',(3.50792001656464,-3.85665852832602,57.6876640661497));
#53130=CARTESIAN_POINT('Ctrl Pts',(1.92824185359667,-4.84367641371333,57.6347438120677));
#53131=CARTESIAN_POINT('Ctrl Pts',(0.295394334515388,-4.94128937853172,
57.5818235579858));
#53132=CARTESIAN_POINT('Ctrl Pts',(-1.33745318456585,-5.03890234335011,
57.5289033039038));
#53133=CARTESIAN_POINT('Ctrl Pts',(-3.02347005976055,-4.24711038759957,
57.4759830498218));
#53134=CARTESIAN_POINT('Ctrl Pts',(-3.99110921895138,-2.92824960303174,
57.4230627957398));
#53135=CARTESIAN_POINT('Ctrl Pts',(-4.60512891022411,-2.09136068211493,
57.3894820153788));
#53136=CARTESIAN_POINT('Ctrl Pts',(-4.9298871379951,-1.04224259902719,57.3559012350179));
#53137=CARTESIAN_POINT('Ctrl Pts',(-4.93623902664834,0.00326946414225537,
57.3223204546569));
#53138=CARTESIAN_POINT('Ctrl Pts',(-4.93573111423024,0.00295138605979709,
57.1776795453432));
#53139=CARTESIAN_POINT('Ctrl Pts',(-4.93017780293081,-1.01634181563486,
57.2104097510422));
#53140=CARTESIAN_POINT('Ctrl Pts',(-4.62285556832308,-2.03870561435216,
57.2431399567412));
#53141=CARTESIAN_POINT('Ctrl Pts',(-4.03754280040764,-2.86388675849859,
57.2758701624402));
#53142=CARTESIAN_POINT('Ctrl Pts',(-3.09117232292437,-4.19809150543631,
57.3287904165222));
#53143=CARTESIAN_POINT('Ctrl Pts',(-1.41806634007047,-5.01681238170109,
57.3817106706042));
#53144=CARTESIAN_POINT('Ctrl Pts',(0.216136297556334,-4.94539021023678,
57.4346309246861));
#53145=CARTESIAN_POINT('Ctrl Pts',(1.85033893518309,-4.87396803877247,57.4875511787681));
#53146=CARTESIAN_POINT('Ctrl Pts',(3.4456382275827,-3.91240281957913,57.5404714328501));
#53147=CARTESIAN_POINT('Ctrl Pts',(4.27200085402752,-2.50072148265561,57.593391686932));
#53148=CARTESIAN_POINT('Ctrl Pts',(5.0983634804724,-1.08904014573198,57.646311941014));
#53149=CARTESIAN_POINT('Ctrl Pts',(5.15578944096228,0.772757308922017,57.699232195096));
#53150=CARTESIAN_POINT('Ctrl Pts',(4.41799973892759,2.23268393138458,57.7521524491779));
#53151=CARTESIAN_POINT('Ctrl Pts',(3.68021003689295,3.69261055384702,57.8050727032599));
#53152=CARTESIAN_POINT('Ctrl Pts',(2.14720467233395,4.75066634411819,57.8579929573418));
#53153=CARTESIAN_POINT('Ctrl Pts',(0.520510313201973,4.9226688132026,57.9109132114238));
#53154=CARTESIAN_POINT('Ctrl Pts',(-1.1061840459301,5.09467128228702,57.9638334655058));
#53155=CARTESIAN_POINT('Ctrl Pts',(-2.8265673996351,4.38062043018456,58.0167537195877));
#53156=CARTESIAN_POINT('Ctrl Pts',(-3.85336605036076,3.10727683230095,58.0696739736697));
#53157=CARTESIAN_POINT('Ctrl Pts',(-4.5519012154505,2.2410161688934,58.1056758308942));
#53158=CARTESIAN_POINT('Ctrl Pts',(-4.92943605312281,1.11590730173118,58.1416776881187));
#53159=CARTESIAN_POINT('Ctrl Pts',(-4.93796046055574,-0.00400002009900308,
58.1776795453432));
#53160=CARTESIAN_POINT('Origin',(0.,0.,16.));
#53161=CARTESIAN_POINT('',(-4.94980236868244,-0.00111614563719775,59.3223204546569));
#53162=CARTESIAN_POINT('',(-4.95000952859661,-0.000636468299896517,59.1776795453432));
#53163=CARTESIAN_POINT('',(-4.942,-6.05220448138622E-16,16.));
#53164=CARTESIAN_POINT('Ctrl Pts',(-4.94980236868244,-0.00111614563719775,
59.3223204546569));
#53165=CARTESIAN_POINT('Ctrl Pts',(-4.94498060556177,1.57441454729254,59.2713573632528));
#53166=CARTESIAN_POINT('Ctrl Pts',(-4.12744131963774,3.15424986030506,59.2203942718487));
#53167=CARTESIAN_POINT('Ctrl Pts',(-2.83642564175097,4.05688157506129,59.1694311804446));
#53168=CARTESIAN_POINT('Ctrl Pts',(-1.49583040281886,4.99417753516308,59.1165109263627));
#53169=CARTESIAN_POINT('Ctrl Pts',(0.355305856754859,5.20125711678249,59.0635906722807));
#53170=CARTESIAN_POINT('Ctrl Pts',(1.86987491274258,4.58335754070639,59.0106704181987));
#53171=CARTESIAN_POINT('Ctrl Pts',(3.38444396873026,3.96545796463031,58.9577501641168));
#53172=CARTESIAN_POINT('Ctrl Pts',(4.56244582113197,2.52257923085877,58.9048299100348));
#53173=CARTESIAN_POINT('Ctrl Pts',(4.86480883102114,0.915004684618019,58.8519096559529));
#53174=CARTESIAN_POINT('Ctrl Pts',(5.16717184091031,-0.692569861622737,
58.7989894018709));
#53175=CARTESIAN_POINT('Ctrl Pts',(4.59389600828695,-2.46484022033272,58.7460691477889));
#53176=CARTESIAN_POINT('Ctrl Pts',(3.40732110962866,-3.59078840801476,58.6931488937069));
#53177=CARTESIAN_POINT('Ctrl Pts',(2.22074621097036,-4.7167365956968,58.640228639625));
#53178=CARTESIAN_POINT('Ctrl Pts',(0.42087224627713,-5.1963626123509,58.5873083855431));
#53179=CARTESIAN_POINT('Ctrl Pts',(-1.16865096927437,-4.81018226757243,
58.5343881314611));
#53180=CARTESIAN_POINT('Ctrl Pts',(-2.75817418482588,-4.42400192279397,
58.4814678773791));
#53181=CARTESIAN_POINT('Ctrl Pts',(-4.13734665123566,-3.17201521658293,
58.4285476232971));
#53182=CARTESIAN_POINT('Ctrl Pts',(-4.67503798418886,-1.62715038691743,
58.3756273692152));
#53183=CARTESIAN_POINT('Ctrl Pts',(-4.85557797114165,-1.10843293863767,
58.3578583976957));
#53184=CARTESIAN_POINT('Ctrl Pts',(-4.94124878297087,-0.556696204625704,
58.3400894261763));
#53185=CARTESIAN_POINT('Ctrl Pts',(-4.9373129524182,-0.00377529733612325,
58.3223204546568));
#53186=CARTESIAN_POINT('Ctrl Pts',(-4.93796046055574,-0.00400002009900308,
58.1776795453432));
#53187=CARTESIAN_POINT('Ctrl Pts',(-4.94196634578065,-0.530279439411995,
58.1945979422007));
#53188=CARTESIAN_POINT('Ctrl Pts',(-4.86448168129051,-1.05541017361004,
58.2115163390581));
#53189=CARTESIAN_POINT('Ctrl Pts',(-4.70052410203468,-1.55198981852916,
58.2284347359156));
#53190=CARTESIAN_POINT('Ctrl Pts',(-4.18766955523667,-3.10527652781102,
58.2813549899975));
#53191=CARTESIAN_POINT('Ctrl Pts',(-2.82874651389436,-4.37921360271005,
58.3342752440795));
#53192=CARTESIAN_POINT('Ctrl Pts',(-1.24561891614835,-4.79082798129515,
58.3871954981615));
#53193=CARTESIAN_POINT('Ctrl Pts',(0.337508681597706,-5.20244235988026,
58.4401157522434));
#53194=CARTESIAN_POINT('Ctrl Pts',(2.14484083574746,-4.75173404215139,58.4930360063254));
#53195=CARTESIAN_POINT('Ctrl Pts',(3.34931474972224,-3.6449540378337,58.5459562604074));
#53196=CARTESIAN_POINT('Ctrl Pts',(4.55378866369698,-2.53817403351603,58.5988765144893));
#53197=CARTESIAN_POINT('Ctrl Pts',(5.15540433749678,-0.775322342609574,
58.6517967685713));
#53198=CARTESIAN_POINT('Ctrl Pts',(4.87885325049583,0.836893177623885,58.7047170226533));
#53199=CARTESIAN_POINT('Ctrl Pts',(4.60230216349487,2.44910869785739,58.7576372767352));
#53200=CARTESIAN_POINT('Ctrl Pts',(3.44758431569312,3.91068804741789,58.8105575308172));
#53201=CARTESIAN_POINT('Ctrl Pts',(1.94311622990263,4.5527901936852,58.8634777848992));
#53202=CARTESIAN_POINT('Ctrl Pts',(0.438648144112182,5.19489233995249,58.9163980389811));
#53203=CARTESIAN_POINT('Ctrl Pts',(-1.41557017966698,5.01751728292666,58.969318293063));
#53204=CARTESIAN_POINT('Ctrl Pts',(-2.77102011755545,4.10183455769855,59.022238547145));
#53205=CARTESIAN_POINT('Ctrl Pts',(-4.09812694403132,3.205299199536,59.0740522132111));
#53206=CARTESIAN_POINT('Ctrl Pts',(-4.94710627363632,1.60101008771938,59.1258658792772));
#53207=CARTESIAN_POINT('Ctrl Pts',(-4.95000952859661,-0.000636468299896517,
59.1776795453432));
#53208=CARTESIAN_POINT('Origin',(0.,0.,16.));
#53209=CARTESIAN_POINT('',(-4.9405850371911,0.0044815032353801,60.3223204546569));
#53210=CARTESIAN_POINT('',(-4.93981933179839,0.00440230787564107,60.1776795453432));
#53211=CARTESIAN_POINT('',(-4.942,-6.05220448138622E-16,16.));
#53212=CARTESIAN_POINT('Ctrl Pts',(-4.9405850371911,0.0044815032353801,
60.3223204546569));
#53213=CARTESIAN_POINT('Ctrl Pts',(-4.94441025446321,0.434877172261215,
60.3084658084932));
#53214=CARTESIAN_POINT('Ctrl Pts',(-4.89283730030809,0.864370712953886,
60.2946111623296));
#53215=CARTESIAN_POINT('Ctrl Pts',(-4.78226597761638,1.27809649658665,60.2807565161659));
#53216=CARTESIAN_POINT('Ctrl Pts',(-4.3599193928029,2.85839478291331,60.2278362620839));
#53217=CARTESIAN_POINT('Ctrl Pts',(-3.07679122526311,4.20864272692144,60.1749160080019));
#53218=CARTESIAN_POINT('Ctrl Pts',(-1.52006052129332,4.71094624750269,60.12199575392));
#53219=CARTESIAN_POINT('Ctrl Pts',(0.0366701826763779,5.21324976808391,
60.069075499838));
#53220=CARTESIAN_POINT('Ctrl Pts',(1.867003423076,4.86760886523835,60.016155245756));
#53221=CARTESIAN_POINT('Ctrl Pts',(3.1333507549704,3.83219409497753,59.9632349916741));
#53222=CARTESIAN_POINT('Ctrl Pts',(4.39969808686486,2.79677932471666,59.9103147375921));
#53223=CARTESIAN_POINT('Ctrl Pts',(5.102059510254,1.07159068704033,59.8573944835102));
#53224=CARTESIAN_POINT('Ctrl Pts',(4.91902371084035,-0.55389914916401,59.8044742294282));
#53225=CARTESIAN_POINT('Ctrl Pts',(4.73598791142671,-2.1793889853683,59.7515539753462));
#53226=CARTESIAN_POINT('Ctrl Pts',(3.66755488921043,-3.70518002010068,59.6986337212642));
#53227=CARTESIAN_POINT('Ctrl Pts',(2.20265591301344,-4.43304697292067,59.6457134671823));
#53228=CARTESIAN_POINT('Ctrl Pts',(0.737756936816448,-5.16091392574066,
59.5927932131003));
#53229=CARTESIAN_POINT('Ctrl Pts',(-1.12360799336121,-5.09085679664823,
59.5398729590184));
#53230=CARTESIAN_POINT('Ctrl Pts',(-2.52964985740424,-4.25493479787751,
59.4869527049364));
#53231=CARTESIAN_POINT('Ctrl Pts',(-3.93569172144728,-3.41901279910679,
59.4340324508545));
#53232=CARTESIAN_POINT('Ctrl Pts',(-4.88641051935565,-1.8172259306578,59.3811121967725));
#53233=CARTESIAN_POINT('Ctrl Pts',(-4.94674280916461,-0.182576327141242,
59.3281919426905));
#53234=CARTESIAN_POINT('Ctrl Pts',(-4.94897409296954,-0.122121681733242,
59.3262347800127));
#53235=CARTESIAN_POINT('Ctrl Pts',(-4.94998754141356,-0.0616220879792628,
59.3242776173348));
#53236=CARTESIAN_POINT('Ctrl Pts',(-4.94980236868244,-0.00111614563719775,
59.3223204546569));
#53237=CARTESIAN_POINT('Ctrl Pts',(-4.95000952859661,-0.000636468299896517,
59.1776795453432));
#53238=CARTESIAN_POINT('Ctrl Pts',(-4.95007153361169,-0.0348429435249772,
59.1787861333591));
#53239=CARTESIAN_POINT('Ctrl Pts',(-4.94974762270576,-0.0690482134159459,
59.179892721375));
#53240=CARTESIAN_POINT('Ctrl Pts',(-4.94903421151526,-0.103245357661693,
59.1809993093909));
#53241=CARTESIAN_POINT('Ctrl Pts',(-4.9149168155888,-1.73865215436347,59.2339195634729));
#53242=CARTESIAN_POINT('Ctrl Pts',(-3.99000047173805,-3.35547535433661,
59.2868398175548));
#53243=CARTESIAN_POINT('Ctrl Pts',(-2.59754102487793,-4.21383196801951,
59.3397600716368));
#53244=CARTESIAN_POINT('Ctrl Pts',(-1.20508157801781,-5.07218858170242,
59.3926803257188));
#53245=CARTESIAN_POINT('Ctrl Pts',(0.654920971851715,-5.17207860909511,
59.4456005798008));
#53246=CARTESIAN_POINT('Ctrl Pts',(2.13130105065146,-4.46779084807236,59.4985208338827));
#53247=CARTESIAN_POINT('Ctrl Pts',(3.60768112945116,-3.76350308704963,59.5514410879647));
#53248=CARTESIAN_POINT('Ctrl Pts',(4.70043873718116,-2.25503753761151,59.6043613420466));
#53249=CARTESIAN_POINT('Ctrl Pts',(4.90951130318629,-0.632691073520989,
59.6572815961286));
#53250=CARTESIAN_POINT('Ctrl Pts',(5.11858386919144,0.98965539056958,59.7102018502105));
#53251=CARTESIAN_POINT('Ctrl Pts',(4.44397139347178,2.7258827693125,59.7631221042925));
#53252=CARTESIAN_POINT('Ctrl Pts',(3.19438684806975,3.78146689731725,59.8160423583745));
#53253=CARTESIAN_POINT('Ctrl Pts',(1.94480230266778,4.83705102532194,59.8689626124565));
#53254=CARTESIAN_POINT('Ctrl Pts',(0.120245687583507,5.21199190258845,59.9218828665384));
#53255=CARTESIAN_POINT('Ctrl Pts',(-1.44433802421679,4.7347108573205,59.9748031206203));
#53256=CARTESIAN_POINT('Ctrl Pts',(-3.00892173601718,4.25742981205253,60.0277233747023));
#53257=CARTESIAN_POINT('Ctrl Pts',(-4.31353254453361,2.92792684424999,60.0806436287843));
#53258=CARTESIAN_POINT('Ctrl Pts',(-4.7611606188609,1.35460281707783,60.1335638828663));
#53259=CARTESIAN_POINT('Ctrl Pts',(-4.88554531419032,0.917415247758462,
60.1482691036919));
#53260=CARTESIAN_POINT('Ctrl Pts',(-4.94375845579816,0.461401140068047,
60.1629743245176));
#53261=CARTESIAN_POINT('Ctrl Pts',(-4.93981933179839,0.00440230787564107,
60.1776795453432));
#53262=CARTESIAN_POINT('Origin',(0.,0.,16.));
#53263=CARTESIAN_POINT('',(-4.93439206002794,-0.00160550854955477,61.3223204546568));
#53264=CARTESIAN_POINT('',(-4.93468237204831,-0.00200522711461992,61.1776795453432));
#53265=CARTESIAN_POINT('',(-4.942,-6.05220448138622E-16,16.));
#53266=CARTESIAN_POINT('Ctrl Pts',(-4.93439206002794,-0.00160550854955477,
61.3223204546568));
#53267=CARTESIAN_POINT('Ctrl Pts',(-4.93169731118072,0.922902919227787,
61.2926539996516));
#53268=CARTESIAN_POINT('Ctrl Pts',(-4.68258000927622,1.84875941269167,61.2629875446464));
#53269=CARTESIAN_POINT('Ctrl Pts',(-4.19611032092476,2.62607248755302,61.2333210896412));
#53270=CARTESIAN_POINT('Ctrl Pts',(-3.3283254943857,4.01267582171134,61.1804008355592));
#53271=CARTESIAN_POINT('Ctrl Pts',(-1.7052638805986,4.92660054644685,61.1274805814773));
#53272=CARTESIAN_POINT('Ctrl Pts',(-0.0696632625637214,4.94962074962347,
61.0745603273953));
#53273=CARTESIAN_POINT('Ctrl Pts',(1.56593735547125,4.97264095280009,61.0216400733134));
#53274=CARTESIAN_POINT('Ctrl Pts',(3.21407697775393,4.10475663441781,60.9687198192314));
#53275=CARTESIAN_POINT('Ctrl Pts',(4.12054174158777,2.74312491350412,60.9157995651494));
#53276=CARTESIAN_POINT('Ctrl Pts',(5.02700650542156,1.3814931925905,60.8628793110674));
#53277=CARTESIAN_POINT('Ctrl Pts',(5.19179641080646,-0.473885930854428,
60.8099590569854));
#53278=CARTESIAN_POINT('Ctrl Pts',(4.53950108025175,-1.97396263329564,60.7570388029035));
#53279=CARTESIAN_POINT('Ctrl Pts',(3.88720574969703,-3.47403933573684,60.7041185488216));
#53280=CARTESIAN_POINT('Ctrl Pts',(2.41782518320256,-4.61881361717445,60.6511982947396));
#53281=CARTESIAN_POINT('Ctrl Pts',(0.803770369403307,-4.88441928262956,
60.5982780406577));
#53282=CARTESIAN_POINT('Ctrl Pts',(-0.810284444395997,-5.15002494808468,
60.5453577865757));
#53283=CARTESIAN_POINT('Ctrl Pts',(-2.56901350550008,-4.53646199755745,
60.4924375324937));
#53284=CARTESIAN_POINT('Ctrl Pts',(-3.66759553500858,-3.32450620797124,
60.4395172784117));
#53285=CARTESIAN_POINT('Ctrl Pts',(-4.47856622242051,-2.42984327576097,
60.4004516704934));
#53286=CARTESIAN_POINT('Ctrl Pts',(-4.92979916533343,-1.20909466877745,
60.3613860625752));
#53287=CARTESIAN_POINT('Ctrl Pts',(-4.9405850371911,0.0044815032353801,
60.3223204546569));
#53288=CARTESIAN_POINT('Ctrl Pts',(-4.93981933179839,0.00440230787564107,
60.1776795453432));
#53289=CARTESIAN_POINT('Ctrl Pts',(-4.9295825759933,-1.18321845466868,60.2158945785995));
#53290=CARTESIAN_POINT('Ctrl Pts',(-4.49960389811683,-2.3774895002097,60.2541096118559));
#53291=CARTESIAN_POINT('Ctrl Pts',(-3.72042358357856,-3.26527909823641,
60.2923246451122));
#53292=CARTESIAN_POINT('Ctrl Pts',(-2.64141313383085,-4.49469189983651,
60.3452448991941));
#53293=CARTESIAN_POINT('Ctrl Pts',(-0.892746894197383,-5.13637241649503,
60.3981651532761));
#53294=CARTESIAN_POINT('Ctrl Pts',(0.72535875721281,-4.89667784359578,60.451085407358));
#53295=CARTESIAN_POINT('Ctrl Pts',(2.34346440862305,-4.65698327069652,60.50400566144));
#53296=CARTESIAN_POINT('Ctrl Pts',(3.83100947181002,-3.53591360823934,60.556925915522));
#53297=CARTESIAN_POINT('Ctrl Pts',(4.50727060703144,-2.0464874555241,60.6098461696039));
#53298=CARTESIAN_POINT('Ctrl Pts',(5.18353174225287,-0.557061302808867,
60.6627664236859));
#53299=CARTESIAN_POINT('Ctrl Pts',(5.04850894950886,1.30072134016443,60.7156866777678));
#53300=CARTESIAN_POINT('Ctrl Pts',(4.16399072092151,2.67671076261644,60.7686069318498));
#53301=CARTESIAN_POINT('Ctrl Pts',(3.27947249233419,4.0527001850684,60.8215271859318));
#53302=CARTESIAN_POINT('Ctrl Pts',(1.64545882790348,4.94689638699909,60.8744474400138));
#53303=CARTESIAN_POINT('Ctrl Pts',(0.00969933627160482,4.95010152961563,
60.9273676940957));
#53304=CARTESIAN_POINT('Ctrl Pts',(-1.62606015536036,4.95330667223218,60.9802879481777));
#53305=CARTESIAN_POINT('Ctrl Pts',(-3.26356547419351,4.06552075553457,61.0332082022597));
#53306=CARTESIAN_POINT('Ctrl Pts',(-4.15346917720423,2.69300817389058,61.0861284563416));
#53307=CARTESIAN_POINT('Ctrl Pts',(-4.66664165108668,1.90153413622322,61.1166454860088));
#53308=CARTESIAN_POINT('Ctrl Pts',(-4.93120852346023,0.948870286286938,
61.147162515676));
#53309=CARTESIAN_POINT('Ctrl Pts',(-4.93468237204831,-0.00200522711461992,
61.1776795453432));
#53310=CARTESIAN_POINT('Origin',(0.,0.,16.));
#53311=CARTESIAN_POINT('',(-4.94646539259968,-0.00363051697945815,62.3223204546568));
#53312=CARTESIAN_POINT('',(-4.94715367607242,-0.003331217148393,62.1776795453432));
#53313=CARTESIAN_POINT('',(-4.942,-6.05220448138622E-16,16.));
#53314=CARTESIAN_POINT('Ctrl Pts',(-4.94646539259968,-0.00363051697945815,
62.3223204546568));
#53315=CARTESIAN_POINT('Ctrl Pts',(-4.93485651568824,1.40483737949782,62.2768421908101));
#53316=CARTESIAN_POINT('Ctrl Pts',(-4.3027525120455,2.82241015727549,62.2313639269634));
#53317=CARTESIAN_POINT('Ctrl Pts',(-3.23996042330606,3.74249315171913,62.1858856631166));
#53318=CARTESIAN_POINT('Ctrl Pts',(-2.00325473986379,4.81313705330919,62.1329654090346));
#53319=CARTESIAN_POINT('Ctrl Pts',(-0.183373993763468,5.2101527640882,62.0800451549526));
#53320=CARTESIAN_POINT('Ctrl Pts',(1.3868765910888,4.75185983130228,62.0271249008706));
#53321=CARTESIAN_POINT('Ctrl Pts',(2.95712717594107,4.29356689851636,61.9742046467886));
#53322=CARTESIAN_POINT('Ctrl Pts',(4.2777475995453,2.97996532216552,61.9212843927068));
#53323=CARTESIAN_POINT('Ctrl Pts',(4.74440178662215,1.4121792458292,61.8683641386248));
#53324=CARTESIAN_POINT('Ctrl Pts',(5.21105597369902,-0.155606830507172,
61.8154438845429));
#53325=CARTESIAN_POINT('Ctrl Pts',(4.82374392424848,-1.97757740682905,61.7625236304608));
#53326=CARTESIAN_POINT('Ctrl Pts',(3.75970554739938,-3.21997092100356,61.7096033763788));
#53327=CARTESIAN_POINT('Ctrl Pts',(2.69566717055032,-4.46236443517805,61.6566831222968));
#53328=CARTESIAN_POINT('Ctrl Pts',(0.954902466302742,-5.12518088720521,
61.603762868215));
#53329=CARTESIAN_POINT('Ctrl Pts',(-0.665988050504544,-4.90510534564135,
61.550842614133));
#53330=CARTESIAN_POINT('Ctrl Pts',(-2.28687856731188,-4.68502980407749,
61.4979223600511));
#53331=CARTESIAN_POINT('Ctrl Pts',(-3.78789489667891,-3.58206226892256,
61.4450021059691));
#53332=CARTESIAN_POINT('Ctrl Pts',(-4.4821490417169,-2.10093752955449,61.3920818518871));
#53333=CARTESIAN_POINT('Ctrl Pts',(-4.78721270168923,-1.45011342271034,
61.3688280528103));
#53334=CARTESIAN_POINT('Ctrl Pts',(-4.9365043160506,-0.726273596479458,
61.3455742537336));
#53335=CARTESIAN_POINT('Ctrl Pts',(-4.93439206002794,-0.00160550854955477,
61.3223204546568));
#53336=CARTESIAN_POINT('Ctrl Pts',(-4.93468237204831,-0.00200522711461992,
61.1776795453432));
#53337=CARTESIAN_POINT('Ctrl Pts',(-4.93723260089922,-0.700063909415997,
61.200082769758));
#53338=CARTESIAN_POINT('Ctrl Pts',(-4.79907061241107,-1.39715879423438,
61.2224859941727));
#53339=CARTESIAN_POINT('Ctrl Pts',(-4.51525583033475,-2.02880852158482,
61.2448892185875));
#53340=CARTESIAN_POINT('Ctrl Pts',(-3.84483669326632,-3.520873388826,61.2978094726695));
#53341=CARTESIAN_POINT('Ctrl Pts',(-2.36169633194117,-4.64776387671811,
61.3507297267514));
#53342=CARTESIAN_POINT('Ctrl Pts',(-0.744542427257826,-4.89379768734264,
61.4036499808334));
#53343=CARTESIAN_POINT('Ctrl Pts',(0.872611477425563,-5.13983149796717,
61.4565702349153));
#53344=CARTESIAN_POINT('Ctrl Pts',(2.62377892546721,-4.50500863132408,61.5094904889973));
#53345=CARTESIAN_POINT('Ctrl Pts',(3.7075989475901,-3.27983372664773,61.5624107430792));
#53346=CARTESIAN_POINT('Ctrl Pts',(4.79141896971299,-2.05465882197138,61.6153309971612));
#53347=CARTESIAN_POINT('Ctrl Pts',(5.20789156591715,-0.23913187926188,61.6682512512432));
#53348=CARTESIAN_POINT('Ctrl Pts',(4.76643251551905,1.33593424450079,61.7211715053252));
#53349=CARTESIAN_POINT('Ctrl Pts',(4.32497346512095,2.91100036826346,61.7740917594072));
#53350=CARTESIAN_POINT('Ctrl Pts',(3.02558276812051,4.24560567307922,61.8270120134891));
#53351=CARTESIAN_POINT('Ctrl Pts',(1.46288145266801,4.72901438843942,61.879932267571));
#53352=CARTESIAN_POINT('Ctrl Pts',(-0.099819862784441,5.2124231037996,61.932852521653));
#53353=CARTESIAN_POINT('Ctrl Pts',(-1.92583179668899,4.84463522970427,61.985772775735));
#53354=CARTESIAN_POINT('Ctrl Pts',(-3.17954339996051,3.79395611445292,62.038693029817));
#53355=CARTESIAN_POINT('Ctrl Pts',(-4.27710053403159,2.87414301265627,62.0850218683257));
#53356=CARTESIAN_POINT('Ctrl Pts',(-4.93604317278978,1.43095786114934,62.1313507068344));
#53357=CARTESIAN_POINT('Ctrl Pts',(-4.94715367607242,-0.003331217148393,
62.1776795453432));
#53358=CARTESIAN_POINT('Origin',(0.,0.,16.));
#53359=CARTESIAN_POINT('',(-4.94566965389892,0.00391030538274315,63.3223204546568));
#53360=CARTESIAN_POINT('',(-4.94490839420487,0.00412192395711707,63.1776795453432));
#53361=CARTESIAN_POINT('',(-4.942,-6.05220448138622E-16,16.));
#53362=CARTESIAN_POINT('Ctrl Pts',(-4.94566965389892,0.00391030538274314,
63.3223204546568));
#53363=CARTESIAN_POINT('Ctrl Pts',(-4.94791640205867,0.263233220344943,
63.3139506360505));
#53364=CARTESIAN_POINT('Ctrl Pts',(-4.92928016281063,0.522232554885722,
63.3055808174441));
#53365=CARTESIAN_POINT('Ctrl Pts',(-4.88863316854879,0.777730209403516,
63.2972109988377));
#53366=CARTESIAN_POINT('Ctrl Pts',(-4.63163246576532,2.39317750047789,63.2442907447558));
#53367=CARTESIAN_POINT('Ctrl Pts',(-3.49470467070217,3.86863762987662,63.1913704906738));
#53368=CARTESIAN_POINT('Ctrl Pts',(-1.99812530633611,4.52891750812856,63.1384502365919));
#53369=CARTESIAN_POINT('Ctrl Pts',(-0.501545941970182,5.18919738638045,
63.0855299825099));
#53370=CARTESIAN_POINT('Ctrl Pts',(1.35468499169859,5.0342970134857,63.0326097284279));
#53371=CARTESIAN_POINT('Ctrl Pts',(2.72112786976736,4.1351011658277,62.979689474346));
#53372=CARTESIAN_POINT('Ctrl Pts',(4.08757074783617,3.23590531816966,62.926769220264));
#53373=CARTESIAN_POINT('Ctrl Pts',(4.96422557030495,1.59241399574832,62.8738489661821));
#53374=CARTESIAN_POINT('Ctrl Pts',(4.94992170152689,-0.0432860717482803,
62.8209287121001));
#53375=CARTESIAN_POINT('Ctrl Pts',(4.93561783274882,-1.67898613924493,62.7680084580182));
#53376=CARTESIAN_POINT('Ctrl Pts',(4.03035527272386,-3.30689495181684,62.7150882039362));
#53377=CARTESIAN_POINT('Ctrl Pts',(2.64839599472191,-4.18205657427003,62.6621679498542));
#53378=CARTESIAN_POINT('Ctrl Pts',(1.26643671671996,-5.05721819672321,62.6092476957723));
#53379=CARTESIAN_POINT('Ctrl Pts',(-0.592219279258987,-5.17963262905766,
62.5563274416903));
#53380=CARTESIAN_POINT('Ctrl Pts',(-2.07702262276162,-4.49328115743837,
62.5034071876083));
#53381=CARTESIAN_POINT('Ctrl Pts',(-3.56182596626416,-3.80692968581911,
62.4504869335263));
#53382=CARTESIAN_POINT('Ctrl Pts',(-4.67277665729038,-2.31181231024634,
62.3975666794443));
#53383=CARTESIAN_POINT('Ctrl Pts',(-4.9014866924115,-0.692117576259364,
62.3446464253624));
#53384=CARTESIAN_POINT('Ctrl Pts',(-4.93364938470368,-0.464345570938786,
62.3372044351272));
#53385=CARTESIAN_POINT('Ctrl Pts',(-4.94836505061889,-0.234109947053592,
62.329762444892));
#53386=CARTESIAN_POINT('Ctrl Pts',(-4.94646539259968,-0.00363051697945815,
62.3223204546568));
#53387=CARTESIAN_POINT('Ctrl Pts',(-4.94715367607242,-0.003331217148393,
62.1776795453432));
#53388=CARTESIAN_POINT('Ctrl Pts',(-4.94873441814843,-0.207394078888273,
62.1842709609164));
#53389=CARTESIAN_POINT('Ctrl Pts',(-4.93720170764577,-0.4112768658406,62.1908623764896));
#53390=CARTESIAN_POINT('Ctrl Pts',(-4.91195301252751,-0.613446683379284,
62.1974537920628));
#53391=CARTESIAN_POINT('Ctrl Pts',(-4.70923974918446,-2.23660000955276,
62.2503740461448));
#53392=CARTESIAN_POINT('Ctrl Pts',(-3.6224019498598,-3.74933630549224,62.3032943002267));
#53393=CARTESIAN_POINT('Ctrl Pts',(-2.14879319047093,-4.45940433860991,
62.3562145543087));
#53394=CARTESIAN_POINT('Ctrl Pts',(-0.675184431082104,-5.16947237172755,
62.4091348083907));
#53395=CARTESIAN_POINT('Ctrl Pts',(1.18519528837092,-5.07687214202343,62.4620550624727));
#53396=CARTESIAN_POINT('Ctrl Pts',(2.58100779524721,-4.22397892886556,62.5149753165546));
#53397=CARTESIAN_POINT('Ctrl Pts',(3.97682030212355,-3.37108571570767,62.5678955706366));
#53398=CARTESIAN_POINT('Ctrl Pts',(4.90806559642314,-1.75789951909599,62.6208158247185));
#53399=CARTESIAN_POINT('Ctrl Pts',(4.94859160884553,-0.122638980307035,
62.6737360788005));
#53400=CARTESIAN_POINT('Ctrl Pts',(4.98911762126792,1.51262155848192,62.7266563328825));
#53401=CARTESIAN_POINT('Ctrl Pts',(4.13892435181312,3.16995643944814,62.7795765869645));
#53402=CARTESIAN_POINT('Ctrl Pts',(2.78707322532942,4.09094390908492,62.8324968410464));
#53403=CARTESIAN_POINT('Ctrl Pts',(1.43522209884579,5.01193137872164,62.8854170951284));
#53404=CARTESIAN_POINT('Ctrl Pts',(-0.418286884666658,5.19657143702902,
62.9383373492103));
#53405=CARTESIAN_POINT('Ctrl Pts',(-1.92525970626815,4.56036997337358,62.9912576032922));
#53406=CARTESIAN_POINT('Ctrl Pts',(-3.43223252786973,3.92416850971811,63.0441778573742));
#53407=CARTESIAN_POINT('Ctrl Pts',(-4.59266918756032,2.46712552409973,63.0970981114562));
#53408=CARTESIAN_POINT('Ctrl Pts',(-4.87553614686583,0.856006139716171,
63.1500183655382));
#53409=CARTESIAN_POINT('Ctrl Pts',(-4.9248205778018,0.57529784411246,63.1592387588066));
#53410=CARTESIAN_POINT('Ctrl Pts',(-4.94746485856309,0.289912292218248,
63.1684591520749));
#53411=CARTESIAN_POINT('Ctrl Pts',(-4.94490839420487,0.00412192395711708,
63.1776795453432));
#53412=CARTESIAN_POINT('Origin',(0.,0.,16.));
#53413=CARTESIAN_POINT('',(-4.93415080838549,0.00115309545102804,64.3223204546568));
#53414=CARTESIAN_POINT('',(-4.9340004404197,0.000727385793248169,64.1776795453432));
#53415=CARTESIAN_POINT('',(-4.942,-6.05220448138622E-16,16.));
#53416=CARTESIAN_POINT('Ctrl Pts',(-4.93415080838549,0.00115309545102804,
64.3223204546568));
#53417=CARTESIAN_POINT('Ctrl Pts',(-4.93572402472308,0.754827492624239,
64.2981388272089));
#53418=CARTESIAN_POINT('Ctrl Pts',(-4.77374496051519,1.5078605887699,64.273957199761));
#53419=CARTESIAN_POINT('Ctrl Pts',(-4.44472183637519,2.17900122361227,64.2497755723131));
#53420=CARTESIAN_POINT('Ctrl Pts',(-3.72467156821878,3.64775815476123,64.1968553182311));
#53421=CARTESIAN_POINT('Ctrl Pts',(-2.20459580691742,4.72430684596657,64.1439350641492));
#53422=CARTESIAN_POINT('Ctrl Pts',(-0.580104436501948,4.91600217432875,
64.0910148100672));
#53423=CARTESIAN_POINT('Ctrl Pts',(1.04438693391362,5.10769750269094,64.0380945559853));
#53424=CARTESIAN_POINT('Ctrl Pts',(2.77329391344336,4.41453946820987,63.9851743019033));
#53425=CARTESIAN_POINT('Ctrl Pts',(3.81544226317875,3.15372777385805,63.9322540478213));
#53426=CARTESIAN_POINT('Ctrl Pts',(4.85759061291414,1.89291607950622,63.8793337937393));
#53427=CARTESIAN_POINT('Ctrl Pts',(5.2129803328552,0.0644507252837223,63.8264135396574));
#53428=CARTESIAN_POINT('Ctrl Pts',(4.71897965939677,-1.49493461711666,63.7734932855754));
#53429=CARTESIAN_POINT('Ctrl Pts',(4.22497898593836,-3.05431995951699,63.7205730314935));
#53430=CARTESIAN_POINT('Ctrl Pts',(2.88158791908043,-4.34462529009514,63.6676527774115));
#53431=CARTESIAN_POINT('Ctrl Pts',(1.30356272822442,-4.77538718313377,63.6147325233296));
#53432=CARTESIAN_POINT('Ctrl Pts',(-0.274462462631595,-5.2061490761724,
63.5618122692476));
#53433=CARTESIAN_POINT('Ctrl Pts',(-2.08712177748574,-4.77736753167153,
63.5088920151656));
#53434=CARTESIAN_POINT('Ctrl Pts',(-3.30491462966089,-3.68525953304616,
63.4559717610837));
#53435=CARTESIAN_POINT('Ctrl Pts',(-4.33010248683659,-2.76587832883282,
63.4114213256081));
#53436=CARTESIAN_POINT('Ctrl Pts',(-4.93371077956384,-1.37640022865803,
63.3668708901324));
#53437=CARTESIAN_POINT('Ctrl Pts',(-4.94566965389892,0.00391030538274314,
63.3223204546568));
#53438=CARTESIAN_POINT('Ctrl Pts',(-4.94490839420487,0.00412192395711708,
63.1776795453432));
#53439=CARTESIAN_POINT('Ctrl Pts',(-4.9327920849133,-1.35037554176026,63.2213794061568));
#53440=CARTESIAN_POINT('Ctrl Pts',(-4.35459996207,-2.71396626059995,63.2650792669704));
#53441=CARTESIAN_POINT('Ctrl Pts',(-3.36357298066115,-3.6318006600574,63.308779127784));
#53442=CARTESIAN_POINT('Ctrl Pts',(-2.16344559623047,-4.74329229229879,
63.361699381866));
#53443=CARTESIAN_POINT('Ctrl Pts',(-0.35789356844863,-5.2010797736329,63.4146196359481));
#53444=CARTESIAN_POINT('Ctrl Pts',(1.22683491911902,-4.7956725609509,63.46753989003));
#53445=CARTESIAN_POINT('Ctrl Pts',(2.81156340668672,-4.39026534826889,63.520460144112));
#53446=CARTESIAN_POINT('Ctrl Pts',(4.17546835404021,-3.12166344157071,63.5733803981938));
#53447=CARTESIAN_POINT('Ctrl Pts',(4.69440602676098,-1.57039844833637,63.6263006522758));
#53448=CARTESIAN_POINT('Ctrl Pts',(5.21334369948175,-0.0191334551020692,
63.6792209063577));
#53449=CARTESIAN_POINT('Ctrl Pts',(4.88731409756984,1.81479462466838,63.7321411604398));
#53450=CARTESIAN_POINT('Ctrl Pts',(3.86551334621209,3.09215229264073,63.7850614145218));
#53451=CARTESIAN_POINT('Ctrl Pts',(2.84371259485431,4.36950996061312,63.8379816686038));
#53452=CARTESIAN_POINT('Ctrl Pts',(1.12614069405063,5.09029721678739,63.8909019226856));
#53453=CARTESIAN_POINT('Ctrl Pts',(-0.501215222432739,4.92467080437148,
63.9438221767676));
#53454=CARTESIAN_POINT('Ctrl Pts',(-2.12857113891606,4.75904439195557,63.9967424308495));
#53455=CARTESIAN_POINT('Ctrl Pts',(-3.66571107107909,3.70700431094953,64.0496626849316));
#53456=CARTESIAN_POINT('Ctrl Pts',(-4.40921630968873,2.24998016991306,64.1025829390136));
#53457=CARTESIAN_POINT('Ctrl Pts',(-4.76090724023141,1.56078236823718,64.1276151411235));
#53458=CARTESIAN_POINT('Ctrl Pts',(-4.93502599479208,0.780971213387874,
64.1526473432333));
#53459=CARTESIAN_POINT('Ctrl Pts',(-4.9340004404197,0.000727385793248169,
64.1776795453432));
#53460=CARTESIAN_POINT('Origin',(0.,0.,16.));
#53461=CARTESIAN_POINT('',(-4.94144181990917,-0.00451754960951789,65.3223204546568));
#53462=CARTESIAN_POINT('',(-4.94223974397651,-0.00450342756324047,65.1776795453432));
#53463=CARTESIAN_POINT('',(-4.942,-6.05220448138622E-16,16.));
#53464=CARTESIAN_POINT('Ctrl Pts',(-4.94144181990917,-0.00451754960951789,
65.3223204546568));
#53465=CARTESIAN_POINT('Ctrl Pts',(-4.93014544737618,1.2373328062097,65.2823270183674));
#53466=CARTESIAN_POINT('Ctrl Pts',(-4.45501720554112,2.48688539619672,65.2423335820779));
#53467=CARTESIAN_POINT('Ctrl Pts',(-3.60889481176119,3.38813765554137,65.2023401457884));
#53468=CARTESIAN_POINT('Ctrl Pts',(-2.48928579044125,4.58069580961582,65.1494198917065));
#53469=CARTESIAN_POINT('Ctrl Pts',(-0.720095544969354,5.16340781391902,
65.0964996376245));
#53470=CARTESIAN_POINT('Ctrl Pts',(0.889067448016765,4.86961575569687,65.0435793835425));
#53471=CARTESIAN_POINT('Ctrl Pts',(2.49823044100288,4.57582369747472,64.9906591294606));
#53472=CARTESIAN_POINT('Ctrl Pts',(3.94736618150317,3.40552757672724,64.9377388753786));
#53473=CARTESIAN_POINT('Ctrl Pts',(4.57332802245098,1.89427277188866,64.8848186212967));
#53474=CARTESIAN_POINT('Ctrl Pts',(5.19928986339881,0.383017967050043,64.8318983672147));
#53475=CARTESIAN_POINT('Ctrl Pts',(5.00207780479406,-1.46919552187978,64.7789781131327));
#53476=CARTESIAN_POINT('Ctrl Pts',(4.07193909661463,-2.81476651406745,64.7260578590508));
#53477=CARTESIAN_POINT('Ctrl Pts',(3.14180038843529,-4.16033750625501,64.6731376049688));
#53478=CARTESIAN_POINT('Ctrl Pts',(1.47873503068148,-4.99926600170063,64.6202173508868));
#53479=CARTESIAN_POINT('Ctrl Pts',(-0.156212869442396,-4.94764550818617,
64.5672970968049));
#53480=CARTESIAN_POINT('Ctrl Pts',(-1.79116076956636,-4.8960250146717,64.5143768427229));
#53481=CARTESIAN_POINT('Ctrl Pts',(-3.39799121206035,-3.95385553219706,
64.461456588641));
#53482=CARTESIAN_POINT('Ctrl Pts',(-4.24139404580168,-2.55228820541339,
64.408536334559));
#53483=CARTESIAN_POINT('Ctrl Pts',(-4.69940845940318,-1.7911595826268,64.379797707925));
#53484=CARTESIAN_POINT('Ctrl Pts',(-4.93228112128365,-0.89455035340317,
64.3510590812909));
#53485=CARTESIAN_POINT('Ctrl Pts',(-4.93415080838549,0.00115309545102804,
64.3223204546568));
#53486=CARTESIAN_POINT('Ctrl Pts',(-4.9340004404197,0.000727385793248169,
64.1776795453432));
#53487=CARTESIAN_POINT('Ctrl Pts',(-4.93285788358386,-0.868532151155221,
64.2055675973153));
#53488=CARTESIAN_POINT('Ctrl Pts',(-4.71432797343864,-1.73832871715993,
64.2334556492873));
#53489=CARTESIAN_POINT('Ctrl Pts',(-4.28176794905193,-2.48396104258879,
64.2613437012593));
#53490=CARTESIAN_POINT('Ctrl Pts',(-3.46094380474913,-3.89886991298749,
64.3142639553413));
#53491=CARTESIAN_POINT('Ctrl Pts',(-1.86942497108703,-4.86667945271791,
64.3671842094234));
#53492=CARTESIAN_POINT('Ctrl Pts',(-0.23551477313756,-4.94450523533559,
64.4201044635053));
#53493=CARTESIAN_POINT('Ctrl Pts',(1.39839542481181,-5.02233101795326,64.4730247175873));
#53494=CARTESIAN_POINT('Ctrl Pts',(3.0746969870487,-4.21017304345841,64.5259449716692));
#53495=CARTESIAN_POINT('Ctrl Pts',(4.0262887170445,-2.87968720482404,64.5788652257512));
#53496=CARTESIAN_POINT('Ctrl Pts',(4.97788044704027,-1.5492013661897,64.6317854798331));
#53497=CARTESIAN_POINT('Ctrl Pts',(5.20476234479506,0.299612336584008,64.6847057339151));
#53498=CARTESIAN_POINT('Ctrl Pts',(4.6031097887974,1.82070851673316,64.7376259879971));
#53499=CARTESIAN_POINT('Ctrl Pts',(4.00145723279969,3.34180469688243,64.790546242079));
#53500=CARTESIAN_POINT('Ctrl Pts',(2.57127022304931,4.535183354407,64.843466496161));
#53501=CARTESIAN_POINT('Ctrl Pts',(0.967024178023638,4.85473618951069,64.896386750243));
#53502=CARTESIAN_POINT('Ctrl Pts',(-0.637221867001943,5.17428902461436,
64.9493070043249));
#53503=CARTESIAN_POINT('Ctrl Pts',(-2.41552694730285,4.62001603729727,65.0022272584069));
#53504=CARTESIAN_POINT('Ctrl Pts',(-3.55411149861537,3.44556101180013,65.0551475124888));
#53505=CARTESIAN_POINT('Ctrl Pts',(-4.43287447301319,2.53911309775405,65.0959915234403));
#53506=CARTESIAN_POINT('Ctrl Pts',(-4.93056880366583,1.26323522569467,65.1368355343917));
#53507=CARTESIAN_POINT('Ctrl Pts',(-4.94223974397651,-0.00450342756324047,
65.1776795453432));
#53508=CARTESIAN_POINT('Origin',(0.,0.,16.));
#53509=CARTESIAN_POINT('',(-4.94946148968121,0.00162189178913478,66.3223204546568));
#53510=CARTESIAN_POINT('',(-4.94905436241693,0.00206350582114702,66.1776795453432));
#53511=CARTESIAN_POINT('',(-4.942,-6.05220448138622E-16,16.));
#53512=CARTESIAN_POINT('Ctrl Pts',(-4.94946148968121,0.00162189178913478,
66.3223204546568));
#53513=CARTESIAN_POINT('Ctrl Pts',(-4.94984329083445,0.0908281755408331,
66.3194354636078));
#53514=CARTESIAN_POINT('Ctrl Pts',(-4.94764036946139,0.180015220631608,
66.3165504725587));
#53515=CARTESIAN_POINT('Ctrl Pts',(-4.9427933546869,0.26905833589981,66.3136654815097));
#53516=CARTESIAN_POINT('Ctrl Pts',(-4.8538831123176,1.90240284342791,66.2607452274277));
#53517=CARTESIAN_POINT('Ctrl Pts',(-3.87529724194047,3.48731832979629,66.2078249733457));
#53518=CARTESIAN_POINT('Ctrl Pts',(-2.45485158348742,4.2985232625058,66.1549047192638));
#53519=CARTESIAN_POINT('Ctrl Pts',(-1.03440592503428,5.10972819521536,66.1019844651818));
#53520=CARTESIAN_POINT('Ctrl Pts',(0.827899521494876,5.14722257426599,66.0490642110999));
#53521=CARTESIAN_POINT('Ctrl Pts',(2.27984534133793,4.39384839916376,65.9961439570179));
#53522=CARTESIAN_POINT('Ctrl Pts',(3.7317911611809,3.64047422406158,65.9432237029359));
#53523=CARTESIAN_POINT('Ctrl Pts',(4.77337735433786,2.09623149480659,65.8903034488539));
#53524=CARTESIAN_POINT('Ctrl Pts',(4.9279581709879,0.467789269060101,65.8373831947719));
#53525=CARTESIAN_POINT('Ctrl Pts',(5.08253898763794,-1.16065295668643,65.78446294069));
#53526=CARTESIAN_POINT('Ctrl Pts',(4.35011442778111,-2.87329467892442,65.7315426866081));
#53527=CARTESIAN_POINT('Ctrl Pts',(3.06585315610755,-3.88640488889663,65.6786224325261));
#53528=CARTESIAN_POINT('Ctrl Pts',(1.78159188443402,-4.89951509886881,65.6257021784442));
#53529=CARTESIAN_POINT('Ctrl Pts',(-0.0545060990562027,-5.21309379657515,
65.5727819243622));
#53530=CARTESIAN_POINT('Ctrl Pts',(-1.60221431494639,-4.6836425807522,65.5198616702802));
#53531=CARTESIAN_POINT('Ctrl Pts',(-3.14992253083658,-4.15419136492924,
65.4669414161983));
#53532=CARTESIAN_POINT('Ctrl Pts',(-4.40924097912677,-2.78171023557699,
65.4140211621163));
#53533=CARTESIAN_POINT('Ctrl Pts',(-4.80388630468793,-1.19426751897802,
65.3611009080343));
#53534=CARTESIAN_POINT('Ctrl Pts',(-4.90028622386234,-0.806503266718003,
65.3481740902418));
#53535=CARTESIAN_POINT('Ctrl Pts',(-4.9450930727896,-0.405912747537303,
65.3352472724493));
#53536=CARTESIAN_POINT('Ctrl Pts',(-4.94144181990917,-0.00451754960951789,
65.3223204546568));
#53537=CARTESIAN_POINT('Ctrl Pts',(-4.94223974397651,-0.00450342756324047,
65.1776795453432));
#53538=CARTESIAN_POINT('Ctrl Pts',(-4.94569046072715,-0.379332437889885,
65.1897557884737));
#53539=CARTESIAN_POINT('Ctrl Pts',(-4.90665339169033,-0.753449924055778,
65.2018320316042));
#53540=CARTESIAN_POINT('Ctrl Pts',(-4.82241576997234,-1.11709684994147,
65.2139082747347));
#53541=CARTESIAN_POINT('Ctrl Pts',(-4.45327146769261,-2.71066262250856,
65.2668285288167));
#53542=CARTESIAN_POINT('Ctrl Pts',(-3.21611884080908,-4.10315710396555,
65.3197487828986));
#53543=CARTESIAN_POINT('Ctrl Pts',(-1.67709782604308,-4.65735355244893,
65.3726690369806));
#53544=CARTESIAN_POINT('Ctrl Pts',(-0.138076811276997,-5.21155000093235,
65.4255892910626));
#53545=CARTESIAN_POINT('Ctrl Pts',(1.70281259137165,-4.92744841644198,65.4785095451446));
#53546=CARTESIAN_POINT('Ctrl Pts',(3.00315127590115,-3.9350580230386,65.5314297992265));
#53547=CARTESIAN_POINT('Ctrl Pts',(4.30348996043062,-2.94266762963524,65.5843500533085));
#53548=CARTESIAN_POINT('Ctrl Pts',(5.06327792684106,-1.24198842731896,65.6372703073904));
#53549=CARTESIAN_POINT('Ctrl Pts',(4.93482459769029,0.388722806969066,65.6901905614724));
#53550=CARTESIAN_POINT('Ctrl Pts',(4.80637126853953,2.019434041257,65.7431108155543));
#53551=CARTESIAN_POINT('Ctrl Pts',(3.78967664382766,3.58017730751661,65.7960310696363));
#53552=CARTESIAN_POINT('Ctrl Pts',(2.34999571149359,4.35673265034576,65.8489513237183));
#53553=CARTESIAN_POINT('Ctrl Pts',(0.910314779159406,5.13328799317498,65.9018715778003));
#53554=CARTESIAN_POINT('Ctrl Pts',(-0.952352460797159,5.1256554125735,65.9547918318822));
#53555=CARTESIAN_POINT('Ctrl Pts',(-2.38562103141592,4.33732769399468,66.0077120859641));
#53556=CARTESIAN_POINT('Ctrl Pts',(-3.81888960203473,3.54899997541583,66.0606323400461));
#53557=CARTESIAN_POINT('Ctrl Pts',(-4.82275950331579,1.97997711885965,66.1135525941282));
#53558=CARTESIAN_POINT('Ctrl Pts',(-4.93784453663019,0.348267946699855,
66.1664728482101));
#53559=CARTESIAN_POINT('Ctrl Pts',(-4.94596822597675,0.233087909497783,
66.1702084139211));
#53560=CARTESIAN_POINT('Ctrl Pts',(-4.94966332434242,0.117595522185004,
66.1739439796322));
#53561=CARTESIAN_POINT('Ctrl Pts',(-4.94905436241693,0.00206350582114702,
66.1776795453432));
#53562=CARTESIAN_POINT('Origin',(0.,0.,16.));
#53563=CARTESIAN_POINT('',(-4.93665814957204,0.00348993981812262,67.3223204546568));
#53564=CARTESIAN_POINT('',(-4.93610990017314,0.00319438934087567,67.1776795453432));
#53565=CARTESIAN_POINT('',(-4.942,-6.05220448138622E-16,16.));
#53566=CARTESIAN_POINT('Ctrl Pts',(-4.93665814957204,0.00348993981812262,
67.3223204546568));
#53567=CARTESIAN_POINT('Ctrl Pts',(-4.94045351450443,0.585476451976408,
67.3036236547662));
#53568=CARTESIAN_POINT('Ctrl Pts',(-4.84535018635696,1.16626258658175,67.2849268548756));
#53569=CARTESIAN_POINT('Ctrl Pts',(-4.64586699339373,1.70865983008581,67.266230054985));
#53570=CARTESIAN_POINT('Ctrl Pts',(-4.08124089061357,3.24388511502926,67.213309800903));
#53571=CARTESIAN_POINT('Ctrl Pts',(-2.68038427233572,4.47156102489275,67.1603895468211));
#53572=CARTESIAN_POINT('Ctrl Pts',(-1.08435052194541,4.82988431339829,67.1074692927391));
#53573=CARTESIAN_POINT('Ctrl Pts',(0.511683228444911,5.18820760190384,67.0545490386571));
#53574=CARTESIAN_POINT('Ctrl Pts',(2.3028941109477,4.67717826905144,67.0016287845752));
#53575=CARTESIAN_POINT('Ctrl Pts',(3.4695966691053,3.53065114235145,66.9487085304932));
#53576=CARTESIAN_POINT('Ctrl Pts',(4.6362992272629,2.38412401565146,66.8957882764113));
#53577=CARTESIAN_POINT('Ctrl Pts',(5.17849346107531,0.602099095103884,66.8428680223293));
#53578=CARTESIAN_POINT('Ctrl Pts',(4.84806300838071,-0.999941799318743,
66.7899477682473));
#53579=CARTESIAN_POINT('Ctrl Pts',(4.51763255568609,-2.60198269374146,66.7370275141654));
#53580=CARTESIAN_POINT('Ctrl Pts',(3.31457741648437,-4.02403956203921,66.6841072600834));
#53581=CARTESIAN_POINT('Ctrl Pts',(1.78943399637315,-4.61535746263258,66.6311870060014));
#53582=CARTESIAN_POINT('Ctrl Pts',(0.264290576262007,-5.20667536322592,
66.5782667519194));
#53583=CARTESIAN_POINT('Ctrl Pts',(-1.5829411247586,-4.96725429611497,66.5253464978375));
#53584=CARTESIAN_POINT('Ctrl Pts',(-2.90693966808815,-4.00665699821556,
66.4724262437555));
#53585=CARTESIAN_POINT('Ctrl Pts',(-4.15875934507,-3.09842744975845,66.4223909807226));
#53586=CARTESIAN_POINT('Ctrl Pts',(-4.94283979803511,-1.54550938030458,
66.3723557176897));
#53587=CARTESIAN_POINT('Ctrl Pts',(-4.94946148968121,0.00162189178913478,
66.3223204546568));
#53588=CARTESIAN_POINT('Ctrl Pts',(-4.94905436241693,0.00206350582114702,
66.1776795453432));
#53589=CARTESIAN_POINT('Ctrl Pts',(-4.94103640614155,-1.51909999692026,
66.2268642337141));
#53590=CARTESIAN_POINT('Ctrl Pts',(-4.18686966888732,-3.04713356331113,
66.276048922085));
#53591=CARTESIAN_POINT('Ctrl Pts',(-2.97080189349508,-3.95953726339747,
66.3252336104559));
#53592=CARTESIAN_POINT('Ctrl Pts',(-1.66237405169773,-4.94123781357185,
66.3781538645379));
#53593=CARTESIAN_POINT('Ctrl Pts',(0.180781797244686,-5.21024342615729,
66.4310741186199));
#53594=CARTESIAN_POINT('Ctrl Pts',(1.71520938689206,-4.643453024393,66.4839943727019));
#53595=CARTESIAN_POINT('Ctrl Pts',(3.24963697653938,-4.07666262262872,66.5369146267838));
#53596=CARTESIAN_POINT('Ctrl Pts',(4.47533630689159,-2.6740762065147,66.5898348808657));
#53597=CARTESIAN_POINT('Ctrl Pts',(4.83140864464272,-1.0775387413447,66.6427551349477));
#53598=CARTESIAN_POINT('Ctrl Pts',(5.18748098239386,0.518998723825342,66.6956753890297));
#53599=CARTESIAN_POINT('Ctrl Pts',(4.67392632754393,2.30948723805131,66.7485956431117));
#53600=CARTESIAN_POINT('Ctrl Pts',(3.52575513351784,3.47457191163166,66.8015158971936));
#53601=CARTESIAN_POINT('Ctrl Pts',(2.37758393949173,4.63965658521205,66.8544361512756));
#53602=CARTESIAN_POINT('Ctrl Pts',(0.59479620628932,5.17933741814667,66.9073564053575));
#53603=CARTESIAN_POINT('Ctrl Pts',(-1.0067771713956,4.84664821890178,66.9602766594395));
#53604=CARTESIAN_POINT('Ctrl Pts',(-2.60835054908043,4.5139590196569,67.0131969135215));
#53605=CARTESIAN_POINT('Ctrl Pts',(-4.02870957124789,3.3088997882326,67.0661171676034));
#53606=CARTESIAN_POINT('Ctrl Pts',(-4.61787625663849,1.78292403343541,67.1190374216854));
#53607=CARTESIAN_POINT('Ctrl Pts',(-4.83549920786993,1.2192680163841,67.138584796238));
#53608=CARTESIAN_POINT('Ctrl Pts',(-4.93971654397597,0.611827024271365,
67.1581321707906));
#53609=CARTESIAN_POINT('Ctrl Pts',(-4.93610990017314,0.00319438934087567,
67.1776795453432));
#53610=CARTESIAN_POINT('Origin',(0.,0.,16.));
#53611=CARTESIAN_POINT('',(-4.93685333923596,-0.0035819126635156,68.3223204546569));
#53612=CARTESIAN_POINT('',(-4.9374673003319,-0.00383358773467055,68.1776795453432));
#53613=CARTESIAN_POINT('',(-4.942,-6.05220448138622E-16,16.));
#53614=CARTESIAN_POINT('Ctrl Pts',(-4.93685333923596,-0.0035819126635156,
68.3223204546569));
#53615=CARTESIAN_POINT('Ctrl Pts',(-4.92964532583484,1.0704814894781,68.2878118459247));
#53616=CARTESIAN_POINT('Ctrl Pts',(-4.585217373837,2.14875374624117,68.2533032371925));
#53617=CARTESIAN_POINT('Ctrl Pts',(-3.93928885933925,2.99759934246388,68.2187946284603));
#53618=CARTESIAN_POINT('Ctrl Pts',(-2.94873310059188,4.29933610551658,68.1658743743783));
#53619=CARTESIAN_POINT('Ctrl Pts',(-1.24912700565894,5.06152146794402,68.1129541202964));
#53620=CARTESIAN_POINT('Ctrl Pts',(0.3817637188463,4.93536776727194,68.0600338662144));
#53621=CARTESIAN_POINT('Ctrl Pts',(2.01265444335154,4.80921406659986,68.0071136121325));
#53622=CARTESIAN_POINT('Ctrl Pts',(3.57482979742896,3.79472130282827,67.9541933580505));
#53623=CARTESIAN_POINT('Ctrl Pts',(4.35341448041909,2.35613685870146,67.9012731039685));
#53624=CARTESIAN_POINT('Ctrl Pts',(5.13199916340922,0.91755241457464,67.8483528498866));
#53625=CARTESIAN_POINT('Ctrl Pts',(5.12699317531198,-0.945123709907305,
67.7954325958046));
#53626=CARTESIAN_POINT('Ctrl Pts',(4.34068733273566,-2.37950247209,67.7425123417227));
#53627=CARTESIAN_POINT('Ctrl Pts',(3.55438149015938,-3.81388123427261,67.6895920876407));
#53628=CARTESIAN_POINT('Ctrl Pts',(1.98677579310383,-4.81996263415611,67.6366718335588));
#53629=CARTESIAN_POINT('Ctrl Pts',(0.355230550111662,-4.93734845757534,
67.5837515794768));
#53630=CARTESIAN_POINT('Ctrl Pts',(-1.27631469288069,-5.05473428099459,
67.5308313253949));
#53631=CARTESIAN_POINT('Ctrl Pts',(-2.9717994818098,-4.28342452794957,67.4779110713129));
#53632=CARTESIAN_POINT('Ctrl Pts',(-3.95534408263313,-2.97638232141527,
67.4249908172309));
#53633=CARTESIAN_POINT('Ctrl Pts',(-4.59140099837083,-2.13111995717548,
67.3907673630395));
#53634=CARTESIAN_POINT('Ctrl Pts',(-4.92971094477425,-1.06180405997696,
67.3565439088482));
#53635=CARTESIAN_POINT('Ctrl Pts',(-4.93665814957204,0.00348993981812262,
67.3223204546568));
#53636=CARTESIAN_POINT('Ctrl Pts',(-4.93610990017314,0.00319438934087567,
67.1776795453432));
#53637=CARTESIAN_POINT('Ctrl Pts',(-4.929952342348,-1.03591311578948,67.2110524248726));
#53638=CARTESIAN_POINT('Ctrl Pts',(-4.60950819503561,-2.07849403525122,
67.2444253044019));
#53639=CARTESIAN_POINT('Ctrl Pts',(-4.00255393693903,-2.91258668755472,
67.2777981839313));
#53640=CARTESIAN_POINT('Ctrl Pts',(-3.0400905832352,-4.23522937557753,67.3307184380133));
#53641=CARTESIAN_POINT('Ctrl Pts',(-1.35718952721374,-5.03362247345304,
67.3836386920952));
#53642=CARTESIAN_POINT('Ctrl Pts',(0.276028005448868,-4.94240910597606,
67.4365589461772));
#53643=CARTESIAN_POINT('Ctrl Pts',(1.90924553811157,-4.85119573849907,67.4894792002592));
#53644=CARTESIAN_POINT('Ctrl Pts',(3.49277954741543,-3.87037590566948,67.5423994543411));
#53645=CARTESIAN_POINT('Ctrl Pts',(4.30198068586489,-2.4487877427561,67.5953197084231));
#53646=CARTESIAN_POINT('Ctrl Pts',(5.11118182431431,-1.0271995798428,67.6482399625051));
#53647=CARTESIAN_POINT('Ctrl Pts',(5.14605009190941,0.835156913154248,67.7011602165871));
#53648=CARTESIAN_POINT('Ctrl Pts',(4.39062923686613,2.28603896182972,67.754080470669));
#53649=CARTESIAN_POINT('Ctrl Pts',(3.63520838182284,3.73692101050519,67.8070007247509));
#53650=CARTESIAN_POINT('Ctrl Pts',(2.08949840414118,4.77632861485907,67.8599209788329));
#53651=CARTESIAN_POINT('Ctrl Pts',(0.460839796771268,4.92861298057972,67.9128412329148));
#53652=CARTESIAN_POINT('Ctrl Pts',(-1.16781881059865,5.08089734630037,67.9657614869968));
#53653=CARTESIAN_POINT('Ctrl Pts',(-2.87942604765681,4.34605847338777,68.0186817410788));
#53654=CARTESIAN_POINT('Ctrl Pts',(-3.89072430186352,3.06036985305955,68.0716019951608));
#53655=CARTESIAN_POINT('Ctrl Pts',(-4.56643308401115,2.20132447426127,68.1069611785549));
#53656=CARTESIAN_POINT('Ctrl Pts',(-4.92949771464715,1.09635914283018,68.142320361949));
#53657=CARTESIAN_POINT('Ctrl Pts',(-4.9374673003319,-0.00383358773467055,
68.1776795453432));
#53658=CARTESIAN_POINT('Origin',(0.,0.,16.));
#53659=CARTESIAN_POINT('',(-4.94957828458471,-0.00146882823891858,69.3223204546568));
#53660=CARTESIAN_POINT('',(-4.94986277816997,-0.00100007488610477,69.1776795453432));
#53661=CARTESIAN_POINT('',(-4.942,-6.05220448138622E-16,16.));
#53662=CARTESIAN_POINT('Ctrl Pts',(-4.94957828458471,-0.00146882823891858,
69.3223204546568));
#53663=CARTESIAN_POINT('Ctrl Pts',(-4.94347825971363,1.5543817607618,69.2720000370831));
#53664=CARTESIAN_POINT('Ctrl Pts',(-4.14920711766337,3.115598423098,69.2216796195094));
#53665=CARTESIAN_POINT('Ctrl Pts',(-2.8853618522021,4.0222239516356,69.1713592019357));
#53666=CARTESIAN_POINT('Ctrl Pts',(-1.55621921401708,4.97569086707049,69.1184389478537));
#53667=CARTESIAN_POINT('Ctrl Pts',(0.292272693635941,5.20517958568956,69.0655186937718));
#53668=CARTESIAN_POINT('Ctrl Pts',(1.81421574235462,4.60567256494064,69.0125984396898));
#53669=CARTESIAN_POINT('Ctrl Pts',(3.3361587910733,4.00616554419172,68.9596781856078));
#53670=CARTESIAN_POINT('Ctrl Pts',(4.53155298085772,2.57766278407475,68.9067579315258));
#53671=CARTESIAN_POINT('Ctrl Pts',(4.85336767356702,0.973868964711821,68.8538376774439));
#53672=CARTESIAN_POINT('Ctrl Pts',(5.17518236627633,-0.629924854651203,
68.8009174233619));
#53673=CARTESIAN_POINT('Ctrl Pts',(4.62341756191056,-2.40900973326008,68.74799716928));
#53674=CARTESIAN_POINT('Ctrl Pts',(3.45056926188509,-3.5492492592361,68.695076915198));
#53675=CARTESIAN_POINT('Ctrl Pts',(2.27772096185968,-4.68948878521204,68.6421566611161));
#53676=CARTESIAN_POINT('Ctrl Pts',(0.483789166174606,-5.19088295855499,
68.5892364070341));
#53677=CARTESIAN_POINT('Ctrl Pts',(-1.11029553728448,-4.82398614790096,
68.5363161529521));
#53678=CARTESIAN_POINT('Ctrl Pts',(-2.70438024074366,-4.45708933724691,
68.4833958988701));
#53679=CARTESIAN_POINT('Ctrl Pts',(-4.09861785197692,-3.22190154259576,
68.4304756447882));
#53680=CARTESIAN_POINT('Ctrl Pts',(-4.65498394631264,-1.6836635634312,68.3775553907063));
#53681=CARTESIAN_POINT('Ctrl Pts',(-4.84855095371391,-1.14849054456963,
68.3591437453565));
#53682=CARTESIAN_POINT('Ctrl Pts',(-4.94069908646524,-0.576635280213381,
68.3407321000067));
#53683=CARTESIAN_POINT('Ctrl Pts',(-4.93685333923596,-0.0035819126635156,
68.3223204546569));
#53684=CARTESIAN_POINT('Ctrl Pts',(-4.9374673003319,-0.00383358773467055,
68.1776795453432));
#53685=CARTESIAN_POINT('Ctrl Pts',(-4.94142537979325,-0.550242199503817,
68.195240616031));
#53686=CARTESIAN_POINT('Ctrl Pts',(-4.85779595713247,-1.09547360479138,
68.2128016867188));
#53687=CARTESIAN_POINT('Ctrl Pts',(-4.68137867571166,-1.60881724419501,
68.2303627574066));
#53688=CARTESIAN_POINT('Ctrl Pts',(-4.14974552399779,-3.15577735337756,
68.2832830114886));
#53689=CARTESIAN_POINT('Ctrl Pts',(-2.77548994921469,-4.41315920399872,
68.3362032655706));
#53690=CARTESIAN_POINT('Ctrl Pts',(-1.18749229097476,-4.8055656575998,68.3891235196525));
#53691=CARTESIAN_POINT('Ctrl Pts',(0.400505367265077,-5.19797211120086,
68.4420437737345));
#53692=CARTESIAN_POINT('Ctrl Pts',(2.20224510896182,-4.72540316778197,68.4949640278164));
#53693=CARTESIAN_POINT('Ctrl Pts',(3.39322331088645,-3.60411359325479,68.5478842818984));
#53694=CARTESIAN_POINT('Ctrl Pts',(4.58420151281108,-2.48282401872761,68.6008045359804));
#53695=CARTESIAN_POINT('Ctrl Pts',(5.16441817496363,-0.71281381309235,68.6537247900624));
#53696=CARTESIAN_POINT('Ctrl Pts',(4.8683572912689,0.895933320719813,68.7066450441443));
#53697=CARTESIAN_POINT('Ctrl Pts',(4.57229640757415,2.50468045453207,68.7595652982263));
#53698=CARTESIAN_POINT('Ctrl Pts',(3.39995797803181,3.95216451652107,68.8124855523082));
#53699=CARTESIAN_POINT('Ctrl Pts',(1.88782197277238,4.57599469293234,68.8654058063902));
#53700=CARTESIAN_POINT('Ctrl Pts',(0.375685967513026,5.19982486934357,68.9183260604721));
#53701=CARTESIAN_POINT('Ctrl Pts',(-1.47624761346349,5.00000116017722,68.9712463145541));
#53702=CARTESIAN_POINT('Ctrl Pts',(-2.82050567947833,4.06796594659513,69.0241665686361));
#53703=CARTESIAN_POINT('Ctrl Pts',(-4.1203297308193,3.16673885490861,69.0753375608718));
#53704=CARTESIAN_POINT('Ctrl Pts',(-4.94548567424374,1.58090626393571,69.1265085531075));
#53705=CARTESIAN_POINT('Ctrl Pts',(-4.94986277816997,-0.00100007488610477,
69.1776795453432));
#53706=CARTESIAN_POINT('Origin',(0.,0.,16.));
#53707=CARTESIAN_POINT('',(-4.94117660785543,0.00451214175946527,70.3223204546568));
#53708=CARTESIAN_POINT('',(-4.94039592783718,0.00446617472429873,70.1776795453432));
#53709=CARTESIAN_POINT('',(-4.942,-6.05220448138622E-16,16.));
#53710=CARTESIAN_POINT('Ctrl Pts',(-4.94117660785543,0.00451214175946527,
70.3223204546568));
#53711=CARTESIAN_POINT('Ctrl Pts',(-4.94488654917412,0.414817947726635,
70.3091084823236));
#53712=CARTESIAN_POINT('Ctrl Pts',(-4.8980529188199,0.824288512579107,70.2958965099902));
#53713=CARTESIAN_POINT('Ctrl Pts',(-4.79739770972192,1.22007120694207,70.2826845376569));
#53714=CARTESIAN_POINT('Ctrl Pts',(-4.39422556359881,2.80536976937794,70.229764283575));
#53715=CARTESIAN_POINT('Ctrl Pts',(-3.12754820616573,4.17106222260404,70.176844029493));
#53716=CARTESIAN_POINT('Ctrl Pts',(-1.57701654176587,4.69218684221452,70.123923775411));
#53717=CARTESIAN_POINT('Ctrl Pts',(-0.0264848773660925,5.21331146182497,
70.071003521329));
#53718=CARTESIAN_POINT('Ctrl Pts',(1.80790109400033,4.88986824781988,70.0180832672471));
#53719=CARTESIAN_POINT('Ctrl Pts',(3.0866983358117,3.86986975477877,69.9651630131651));
#53720=CARTESIAN_POINT('Ctrl Pts',(4.36549557762306,2.84987126173766,69.9122427590831));
#53721=CARTESIAN_POINT('Ctrl Pts',(5.08870408987935,1.13331748966031,69.8593225050012));
#53722=CARTESIAN_POINT('Ctrl Pts',(4.9253726120261,-0.494270338941504,69.8064022509192));
#53723=CARTESIAN_POINT('Ctrl Pts',(4.76204113417285,-2.12185816754332,69.7534819968373));
#53724=CARTESIAN_POINT('Ctrl Pts',(3.71216966621028,-3.66048005266973,69.7005617427553));
#53725=CARTESIAN_POINT('Ctrl Pts',(2.25619542624873,-4.40603912077827,69.6476414886733));
#53726=CARTESIAN_POINT('Ctrl Pts',(0.80022118628726,-5.15159818888676,69.5947212345913));
#53727=CARTESIAN_POINT('Ctrl Pts',(-1.06185582567303,-5.10409443997744,
69.5418009805094));
#53728=CARTESIAN_POINT('Ctrl Pts',(-2.47792073001783,-4.28526631506165,
69.4888807264275));
#53729=CARTESIAN_POINT('Ctrl Pts',(-3.89398563436272,-3.46643819014582,
69.4359604723455));
#53730=CARTESIAN_POINT('Ctrl Pts',(-4.864038431092,-1.87628568922347,69.3830402182635));
#53731=CARTESIAN_POINT('Ctrl Pts',(-4.94416814509815,-0.242486882636884,
69.3301199641816));
#53732=CARTESIAN_POINT('Ctrl Pts',(-4.94810471266539,-0.162222532848887,
69.3275201276733));
#53733=CARTESIAN_POINT('Ctrl Pts',(-4.94989344626512,-0.081852842476203,
69.3249202911651));
#53734=CARTESIAN_POINT('Ctrl Pts',(-4.94957828458471,-0.00146882823891858,
69.3223204546568));
#53735=CARTESIAN_POINT('Ctrl Pts',(-4.94986277816997,-0.00100007488610477,
69.1776795453432));
#53736=CARTESIAN_POINT('Ctrl Pts',(-4.95001240788323,-0.0550769704471047,
69.1794288071895));
#53737=CARTESIAN_POINT('Ctrl Pts',(-4.94920288408253,-0.10914927783116,
69.1811780690357));
#53738=CARTESIAN_POINT('Ctrl Pts',(-4.94742038040276,-0.163189491703912,
69.182927330882));
#53739=CARTESIAN_POINT('Ctrl Pts',(-4.89349446425897,-1.79806299842275,
69.2358475849639));
#53740=CARTESIAN_POINT('Ctrl Pts',(-3.94906008091826,-3.40356329386249,
69.2887678390458));
#53741=CARTESIAN_POINT('Ctrl Pts',(-2.54630482825922,-4.24498892250744,
69.3416880931278));
#53742=CARTESIAN_POINT('Ctrl Pts',(-1.14354957560017,-5.0864145511524,69.3946083472098));
#53743=CARTESIAN_POINT('Ctrl Pts',(0.717526546377131,-5.16376551300254,
69.4475286012918));
#53744=CARTESIAN_POINT('Ctrl Pts',(2.18526668060081,-4.44164482655728,69.5004488553738));
#53745=CARTESIAN_POINT('Ctrl Pts',(3.65300681482441,-3.71952414011206,69.5533691094558));
#53746=CARTESIAN_POINT('Ctrl Pts',(4.72741096129446,-2.19793180537131,69.6062893635377));
#53747=CARTESIAN_POINT('Ctrl Pts',(4.91681537353513,-0.573171713534203,
69.6592096176196));
#53748=CARTESIAN_POINT('Ctrl Pts',(5.1062197857758,1.05158837830299,69.7121298717016));
#53749=CARTESIAN_POINT('Ctrl Pts',(4.41062446378718,2.77951622723674,69.7650501257836));
#53750=CARTESIAN_POINT('Ctrl Pts',(3.14834445052908,3.81988565947332,69.8179703798655));
#53751=CARTESIAN_POINT('Ctrl Pts',(1.88606443727098,4.8602550917099,69.8708906339475));
#53752=CARTESIAN_POINT('Ctrl Pts',(0.0570997327434936,5.21306610724925,
69.9238108880295));
#53753=CARTESIAN_POINT('Ctrl Pts',(-1.50158748103454,4.71686699700421,69.9767311421114));
#53754=CARTESIAN_POINT('Ctrl Pts',(-3.06027469481266,4.22066788675913,70.0296513961934));
#53755=CARTESIAN_POINT('Ctrl Pts',(-4.34868441784121,2.87545865072958,70.0825716502754));
#53756=CARTESIAN_POINT('Ctrl Pts',(-4.77722068336862,1.29682758029823,70.1354919043573));
#53757=CARTESIAN_POINT('Ctrl Pts',(-4.8910960129131,0.877336517731382,70.1495544513526));
#53758=CARTESIAN_POINT('Ctrl Pts',(-4.9442531721895,0.441362859310636,70.1636169983479));
#53759=CARTESIAN_POINT('Ctrl Pts',(-4.94039592783718,0.00446617472429873,
70.1776795453432));
#53760=CARTESIAN_POINT('Origin',(0.,0.,16.));
#53761=CARTESIAN_POINT('',(-4.93421645959303,-0.00129368103133631,71.3223204546568));
#53762=CARTESIAN_POINT('',(-4.93445704478049,-0.00170468936910681,71.1776795453431));
#53763=CARTESIAN_POINT('',(-4.942,-6.05220448138622E-16,16.));
#53764=CARTESIAN_POINT('Ctrl Pts',(-4.93421645959303,-0.00129368103133631,
71.3223204546568));
#53765=CARTESIAN_POINT('Ctrl Pts',(-4.93209641645617,0.903267203006942,
71.293296673482));
#53766=CARTESIAN_POINT('Ctrl Pts',(-4.69429817649842,1.80886543486343,71.2642728923071));
#53767=CARTESIAN_POINT('Ctrl Pts',(-4.22761420074216,2.5750488742813,71.2352491111322));
#53768=CARTESIAN_POINT('Ctrl Pts',(-3.37669011114097,3.97206265560444,71.1823288570503));
#53769=CARTESIAN_POINT('Ctrl Pts',(-1.76481870913523,4.90558179736215,71.1294086029683));
#53770=CARTESIAN_POINT('Ctrl Pts',(-0.129616965909283,4.94841368292938,
71.0764883488863));
#53771=CARTESIAN_POINT('Ctrl Pts',(1.50558477731675,4.9912455684966,71.0235680948044));
#53772=CARTESIAN_POINT('Ctrl Pts',(3.164116861763,4.14339019787323,70.9706478407224));
#53773=CARTESIAN_POINT('Ctrl Pts',(4.08700967532571,2.79283913769631,70.9177275866405));
#53774=CARTESIAN_POINT('Ctrl Pts',(5.00990248888837,1.44228807751946,70.8648073325585));
#53775=CARTESIAN_POINT('Ctrl Pts',(5.19715603156758,-0.410958672210887,
70.8118870784765));
#53776=CARTESIAN_POINT('Ctrl Pts',(4.56308022236637,-1.91882709473861,70.7589668243946));
#53777=CARTESIAN_POINT('Ctrl Pts',(3.92900441316517,-3.42669551726634,70.7060465703126));
#53778=CARTESIAN_POINT('Ctrl Pts',(2.47359925208355,-4.58918561259145,70.6531263162307));
#53779=CARTESIAN_POINT('Ctrl Pts',(0.86288036879719,-4.87432415873202,70.6002060621487));
#53780=CARTESIAN_POINT('Ctrl Pts',(-0.747838514489167,-5.1594627048726,
70.5472858080667));
#53781=CARTESIAN_POINT('Ctrl Pts',(-2.51387111998026,-4.56724970182864,
70.4943655539847));
#53782=CARTESIAN_POINT('Ctrl Pts',(-3.62705395531922,-3.36869086448392,
70.4414452999028));
#53783=CARTESIAN_POINT('Ctrl Pts',(-4.46232163175454,-2.46936200011537,
70.4017370181541));
#53784=CARTESIAN_POINT('Ctrl Pts',(-4.93002646377116,-1.22865260726002,
70.3620287364055));
#53785=CARTESIAN_POINT('Ctrl Pts',(-4.94117660785543,0.00451214175946527,
70.3223204546568));
#53786=CARTESIAN_POINT('Ctrl Pts',(-4.94039592783718,0.00446617472429873,
70.1776795453432));
#53787=CARTESIAN_POINT('Ctrl Pts',(-4.92973756905946,-1.20276914349332,
70.2165372524299));
#53788=CARTESIAN_POINT('Ctrl Pts',(-4.48375687255021,-2.4170520476298,70.2553949595166));
#53789=CARTESIAN_POINT('Ctrl Pts',(-3.68059559417778,-3.31010805001079,
70.2942526666032));
#53790=CARTESIAN_POINT('Ctrl Pts',(-2.58677143143322,-4.52635970505561,
70.3471729206852));
#53791=CARTESIAN_POINT('Ctrl Pts',(-0.83046029791784,-5.14681011031225,
70.4000931747671));
#53792=CARTESIAN_POINT('Ctrl Pts',(0.784623008060776,-4.88753168438311,
70.453013428849));
#53793=CARTESIAN_POINT('Ctrl Pts',(2.3997063140393,-4.62825325845398,70.505933682931));
#53794=CARTESIAN_POINT('Ctrl Pts',(3.87356179248119,-3.48924600133894,70.558853937013));
#53795=CARTESIAN_POINT('Ctrl Pts',(4.53173066670028,-1.99173702960891,70.611774191095));
#53796=CARTESIAN_POINT('Ctrl Pts',(5.18989954091941,-0.494228057878804,
70.664694445177));
#53797=CARTESIAN_POINT('Ctrl Pts',(5.0323818109159,1.36178262846646,70.7176146992589));
#53798=CARTESIAN_POINT('Ctrl Pts',(4.13125999566019,2.72695619306305,70.7705349533408));
#53799=CARTESIAN_POINT('Ctrl Pts',(3.23013818040442,4.09212975765972,70.8234552074228));
#53800=CARTESIAN_POINT('Ctrl Pts',(1.58541227989642,4.96646620050757,70.8763754615048));
#53801=CARTESIAN_POINT('Ctrl Pts',(-0.0502660143879759,4.94985581188227,
70.9292957155868));
#53802=CARTESIAN_POINT('Ctrl Pts',(-1.68594430867228,4.93324542325696,70.9822159696687));
#53803=CARTESIAN_POINT('Ctrl Pts',(-3.3125749967329,4.02568820315859,71.0351362237507));
#53804=CARTESIAN_POINT('Ctrl Pts',(-4.18578703267271,2.64249619635225,71.0880564778327));
#53805=CARTESIAN_POINT('Ctrl Pts',(-4.67872962214464,1.86166150614078,71.1179308336695));
#53806=CARTESIAN_POINT('Ctrl Pts',(-4.93157361279594,0.929252063276933,
71.1478051895063));
#53807=CARTESIAN_POINT('Ctrl Pts',(-4.93445704478049,-0.00170468936910681,
71.1776795453431));
#53808=CARTESIAN_POINT('Origin',(0.,0.,16.));
#53809=CARTESIAN_POINT('',(-4.9459185577707,-0.00382965742011687,72.3223204546568));
#53810=CARTESIAN_POINT('',(-4.9466376895248,-0.00356105100536129,72.1776795453432));
#53811=CARTESIAN_POINT('',(-4.942,-6.05220448138622E-16,16.));
#53812=CARTESIAN_POINT('Ctrl Pts',(-4.9459185577707,-0.00382965742011687,
72.3223204546568));
#53813=CARTESIAN_POINT('Ctrl Pts',(-4.93404671791329,1.38513423103216,72.2774848646404));
#53814=CARTESIAN_POINT('Ctrl Pts',(-4.32176677967432,2.78326338156107,72.232649274624));
#53815=CARTESIAN_POINT('Ctrl Pts',(-3.28505857961465,3.70297024883463,72.1878136846076));
#53816=CARTESIAN_POINT('Ctrl Pts',(-2.06141322698447,4.78851682197505,72.1348934305256));
#53817=CARTESIAN_POINT('Ctrl Pts',(-0.246475391513582,5.20754910952386,
72.0819731764437));
#53818=CARTESIAN_POINT('Ctrl Pts',(1.32921165428745,4.76831153694478,72.0290529223617));
#53819=CARTESIAN_POINT('Ctrl Pts',(2.90489870008848,4.32907396436569,71.9761326682797));
#53820=CARTESIAN_POINT('Ctrl Pts',(4.24133495621976,3.03156653165866,71.9232124141978));
#53821=CARTESIAN_POINT('Ctrl Pts',(4.72694678088706,1.46954845647079,71.8702921601158));
#53822=CARTESIAN_POINT('Ctrl Pts',(5.21255860555439,-0.09246961871717,71.8173719060338));
#53823=CARTESIAN_POINT('Ctrl Pts',(4.84734599875778,-1.91899833638585,71.7644516519519));
#53824=CARTESIAN_POINT('Ctrl Pts',(3.79843582714949,-3.17419025930731,71.7115313978699));
#53825=CARTESIAN_POINT('Ctrl Pts',(2.74952565554119,-4.42938218222877,71.658611143788));
#53826=CARTESIAN_POINT('Ctrl Pts',(1.0169179191211,-5.1132373104028,71.605690889706));
#53827=CARTESIAN_POINT('Ctrl Pts',(-0.60651962032857,-4.91281309286346,
71.552770635624));
#53828=CARTESIAN_POINT('Ctrl Pts',(-2.22995715977815,-4.71238887532414,
71.4998503815421));
#53829=CARTESIAN_POINT('Ctrl Pts',(-3.74422450225742,-3.62768531207155,
71.4469301274601));
#53830=CARTESIAN_POINT('Ctrl Pts',(-4.45636978489872,-2.15507932000099,
71.3940098733781));
#53831=CARTESIAN_POINT('Ctrl Pts',(-4.77794345735694,-1.49011484084619,
71.370113400471));
#53832=CARTESIAN_POINT('Ctrl Pts',(-4.93596197831358,-0.746055865118146,
71.3462169275639));
#53833=CARTESIAN_POINT('Ctrl Pts',(-4.93421645959303,-0.00129368103133631,
71.3223204546568));
#53834=CARTESIAN_POINT('Ctrl Pts',(-4.93445704478049,-0.00170468936910681,
71.1776795453431));
#53835=CARTESIAN_POINT('Ctrl Pts',(-4.93668140337337,-0.71987028628676,
71.2007254435883));
#53836=CARTESIAN_POINT('Ctrl Pts',(-4.79015415455198,-1.43717138679696,
71.2237713418334));
#53837=CARTESIAN_POINT('Ctrl Pts',(-4.49034790212576,-2.08335665417659,
71.2468172400785));
#53838=CARTESIAN_POINT('Ctrl Pts',(-3.80190335182005,-3.56719070438483,
71.2997374941605));
#53839=CARTESIAN_POINT('Ctrl Pts',(-2.30522086738965,-4.67603201128707,
71.3526577482425));
#53840=CARTESIAN_POINT('Ctrl Pts',(-0.685205212090817,-4.90245785784546,
71.4055780023244));
#53841=CARTESIAN_POINT('Ctrl Pts',(0.934810443208014,-5.12888370440385,
71.4584982564064));
#53842=CARTESIAN_POINT('Ctrl Pts',(2.67815926937537,-4.47289409061839,71.5114185104883));
#53843=CARTESIAN_POINT('Ctrl Pts',(3.74705821791536,-3.23467988248916,71.5643387645703));
#53844=CARTESIAN_POINT('Ctrl Pts',(4.8159571664554,-1.99646567435987,71.6172590186523));
#53845=CARTESIAN_POINT('Ctrl Pts',(5.21040623736806,-0.176026871886955,
71.6701792727342));
#53846=CARTESIAN_POINT('Ctrl Pts',(4.74989951150191,1.39357592590467,71.7230995268162));
#53847=CARTESIAN_POINT('Ctrl Pts',(4.28939278563578,2.96317872369621,71.7760197808982));
#53848=CARTESIAN_POINT('Ctrl Pts',(2.97393026299076,4.28194551680631,71.8289400349801));
#53849=CARTESIAN_POINT('Ctrl Pts',(1.40548768459228,4.74638847957966,71.8818602890621));
#53850=CARTESIAN_POINT('Ctrl Pts',(-0.162954893806299,5.21083144235304,
71.934780543144));
#53851=CARTESIAN_POINT('Ctrl Pts',(-1.98437752795848,4.82095057478956,71.987700797226));
#53852=CARTESIAN_POINT('Ctrl Pts',(-3.22526940243671,3.7551613164194,72.040621051308));
#53853=CARTESIAN_POINT('Ctrl Pts',(-4.29653392126676,2.83506324782479,72.0863072159864));
#53854=CARTESIAN_POINT('Ctrl Pts',(-4.93513440489649,1.41121710573191,72.1319933806648));
#53855=CARTESIAN_POINT('Ctrl Pts',(-4.9466376895248,-0.00356105100536129,
72.1776795453432));
#53856=CARTESIAN_POINT('Origin',(0.,0.,16.));
#53857=CARTESIAN_POINT('',(-4.94622533435752,0.00372181280100414,73.3223204546568));
#53858=CARTESIAN_POINT('',(-4.94548609638219,0.00396606047658106,73.1776795453432));
#53859=CARTESIAN_POINT('',(-4.942,-6.05220448138622E-16,16.));
#53860=CARTESIAN_POINT('Ctrl Pts',(-4.94622533435752,0.00372181280100414,
73.3223204546568));
#53861=CARTESIAN_POINT('Ctrl Pts',(-4.94823216917571,0.243062776937041,
73.3145933098808));
#53862=CARTESIAN_POINT('Ctrl Pts',(-4.93236152324834,0.482136497176127,
73.3068661651048));
#53863=CARTESIAN_POINT('Ctrl Pts',(-4.89769574881769,0.718453121134063,
73.2991390203288));
#53864=CARTESIAN_POINT('Ctrl Pts',(-4.66028314118601,2.33689513900433,73.2462187662469));
#53865=CARTESIAN_POINT('Ctrl Pts',(-3.5413122266531,3.82601954517773,73.1932985121649));
#53866=CARTESIAN_POINT('Ctrl Pts',(-2.05284118541496,4.50438026844074,73.1403782580829));
#53867=CARTESIAN_POINT('Ctrl Pts',(-0.564370144176819,5.18274099170376,
73.087458004001));
#53868=CARTESIAN_POINT('Ctrl Pts',(1.29360102376645,5.05033803205637,73.034537749919));
#53869=CARTESIAN_POINT('Ctrl Pts',(2.67083633572998,4.16776100598374,72.9816174958371));
#53870=CARTESIAN_POINT('Ctrl Pts',(4.04807164769343,3.28518397991116,72.9286972417551));
#53871=CARTESIAN_POINT('Ctrl Pts',(4.9445711036771,1.6524328874135,72.8757769876731));
#53872=CARTESIAN_POINT('Ctrl Pts',(4.95008286065676,0.0166795649332413,
72.8228567335911));
#53873=CARTESIAN_POINT('Ctrl Pts',(4.95559461763642,-1.61907375754711,72.7699364795092));
#53874=CARTESIAN_POINT('Ctrl Pts',(4.07011867561174,-3.25782931001015,72.7170162254272));
#53875=CARTESIAN_POINT('Ctrl Pts',(2.69886234926083,-4.14966752342842,72.6640959713453));
#53876=CARTESIAN_POINT('Ctrl Pts',(1.32760602290984,-5.04150573684673,72.6111757172633));
#53877=CARTESIAN_POINT('Ctrl Pts',(-0.529430687767451,-5.18642661122039,
72.5582554631813));
#53878=CARTESIAN_POINT('Ctrl Pts',(-2.02243942200268,-4.51811214110315,
72.5053352090994));
#53879=CARTESIAN_POINT('Ctrl Pts',(-3.51544815623782,-3.84979767098594,
72.4524149550174));
#53880=CARTESIAN_POINT('Ctrl Pts',(-4.64442891403086,-2.36824785637795,
72.3994947009354));
#53881=CARTESIAN_POINT('Ctrl Pts',(-4.89274285803262,-0.751442519707904,
72.3465744468535));
#53882=CARTESIAN_POINT('Ctrl Pts',(-4.93067795216383,-0.50444204261031,
72.3384897827879));
#53883=CARTESIAN_POINT('Ctrl Pts',(-4.9480592642285,-0.254284852349217,
72.3304051187224));
#53884=CARTESIAN_POINT('Ctrl Pts',(-4.9459185577707,-0.00382965742011687,
72.3223204546568));
#53885=CARTESIAN_POINT('Ctrl Pts',(-4.9466376895248,-0.00356105100536129,
72.1776795453432));
#53886=CARTESIAN_POINT('Ctrl Pts',(-4.94845915538918,-0.227581424440414,
72.1849136347467));
#53887=CARTESIAN_POINT('Ctrl Pts',(-4.93455770132463,-0.451374440445247,
72.1921477241503));
#53888=CARTESIAN_POINT('Ctrl Pts',(-4.90416141521875,-0.672904186423828,
72.1993818135539));
#53889=CARTESIAN_POINT('Ctrl Pts',(-4.68180043871832,-2.29348278172022,
72.2523020676359));
#53890=CARTESIAN_POINT('Ctrl Pts',(-3.57671737091314,-3.79294232313627,
72.3052223217178));
#53891=CARTESIAN_POINT('Ctrl Pts',(-2.09461510123176,-4.48510722372598,
72.3581425757998));
#53892=CARTESIAN_POINT('Ctrl Pts',(-0.612512831550301,-5.17727212431573,
72.4110628298817));
#53893=CARTESIAN_POINT('Ctrl Pts',(1.24660864000739,-5.06214238407903,72.4639830839637));
#53894=CARTESIAN_POINT('Ctrl Pts',(2.63198693425408,-4.19240313049007,72.5169033380457));
#53895=CARTESIAN_POINT('Ctrl Pts',(4.01736522850069,-3.32266387690115,72.5698235921276));
#53896=CARTESIAN_POINT('Ctrl Pts',(4.92900034543634,-1.69831510996005,72.6227438462096));
#53897=CARTESIAN_POINT('Ctrl Pts',(4.94971413242267,-0.0626836336085702,
72.6756641002916));
#53898=CARTESIAN_POINT('Ctrl Pts',(4.97042791940901,1.57294784274291,72.7285843543735));
#53899=CARTESIAN_POINT('Ctrl Pts',(4.10022037644603,3.21986202850478,72.7815046084555));
#53900=CARTESIAN_POINT('Ctrl Pts',(2.73731176561134,4.12440583944801,72.8344248625374));
#53901=CARTESIAN_POINT('Ctrl Pts',(1.37440315477665,5.02894965039124,72.8873451166194));
#53902=CARTESIAN_POINT('Ctrl Pts',(-0.481206523929751,5.19112308651582,
72.9402653707013));
#53903=CARTESIAN_POINT('Ctrl Pts',(-1.98036194136401,4.53671310662511,72.9931856247833));
#53904=CARTESIAN_POINT('Ctrl Pts',(-3.47951735879827,3.8823031267344,73.0461058788653));
#53905=CARTESIAN_POINT('Ctrl Pts',(-4.62221851496038,2.41130973082838,73.0990261329473));
#53906=CARTESIAN_POINT('Ctrl Pts',(-4.88554790865992,0.796881962912803,
73.1519463870292));
#53907=CARTESIAN_POINT('Ctrl Pts',(-4.92823035034716,0.535203165516849,
73.1605241064672));
#53908=CARTESIAN_POINT('Ctrl Pts',(-4.94780958080646,0.269756002185876,
73.1691018259052));
#53909=CARTESIAN_POINT('Ctrl Pts',(-4.94548609638219,0.00396606047658106,
73.1776795453432));
#53910=CARTESIAN_POINT('Origin',(0.,0.,16.));
#53911=CARTESIAN_POINT('',(-4.93430944804537,0.00146807591443893,74.3223204546568));
#53912=CARTESIAN_POINT('',(-4.93410780896188,0.00104985362950368,74.1776795453432));
#53913=CARTESIAN_POINT('',(-4.942,-6.05220448138622E-16,16.));
#53914=CARTESIAN_POINT('Ctrl Pts',(-4.93430944804537,0.00146807591443893,
74.3223204546568));
#53915=CARTESIAN_POINT('Ctrl Pts',(-4.93626271862051,0.735053226945857,
74.2987815010393));
#53916=CARTESIAN_POINT('Ctrl Pts',(-4.78313292282981,1.46786315098495,74.2752425474217));
#53917=CARTESIAN_POINT('Ctrl Pts',(-4.47079173349639,2.12499877904777,74.2517035938041));
#53918=CARTESIAN_POINT('Ctrl Pts',(-3.76858655614047,3.60237049949084,74.1987833397222));
#53919=CARTESIAN_POINT('Ctrl Pts',(-2.2616634474919,4.69725412310252,74.1458630856402));
#53920=CARTESIAN_POINT('Ctrl Pts',(-0.639613436851163,4.9086141818902,74.0929428315583));
#53921=CARTESIAN_POINT('Ctrl Pts',(0.982436573789575,5.11997424067789,74.0400225774763));
#53922=CARTESIAN_POINT('Ctrl Pts',(2.71961348642258,4.44781073464159,73.9871023233943));
#53923=CARTESIAN_POINT('Ctrl Pts',(3.77695861444706,3.19971594989436,73.9341820693124));
#53924=CARTESIAN_POINT('Ctrl Pts',(4.83430374247159,1.95162116514706,73.8812618152304));
#53925=CARTESIAN_POINT('Ctrl Pts',(5.21181708588759,0.127595101688968,73.8283415611484));
#53926=CARTESIAN_POINT('Ctrl Pts',(4.73674277310034,-1.43766005604103,73.7754213070665));
#53927=CARTESIAN_POINT('Ctrl Pts',(4.26166846031312,-3.00291521377094,73.7225010529845));
#53928=CARTESIAN_POINT('Ctrl Pts',(2.9340064913226,-4.30939946577263,73.6695807989026));
#53929=CARTESIAN_POINT('Ctrl Pts',(1.36131526012037,-4.7592456647895,73.6166605448206));
#53930=CARTESIAN_POINT('Ctrl Pts',(-0.211375971081961,-5.2090918638064,
73.5637402907386));
#53931=CARTESIAN_POINT('Ctrl Pts',(-2.02909646449615,-4.80230000983842,
73.5108200366566));
#53932=CARTESIAN_POINT('Ctrl Pts',(-3.260029560838,-3.72502426807083,73.4578997825747));
#53933=CARTESIAN_POINT('Ctrl Pts',(-4.31122810355742,-2.80504681907828,
73.4127066732687));
#53934=CARTESIAN_POINT('Ctrl Pts',(-4.9344881263814,-1.3960917881023,73.3675135639628));
#53935=CARTESIAN_POINT('Ctrl Pts',(-4.94622533435752,0.00372181280100414,
73.3223204546568));
#53936=CARTESIAN_POINT('Ctrl Pts',(-4.94548609638219,0.00396606047658106,
73.1776795453432));
#53937=CARTESIAN_POINT('Ctrl Pts',(-4.9334748398561,-1.37003547728531,73.2220220799872));
#53938=CARTESIAN_POINT('Ctrl Pts',(-4.33614096919029,-2.75319733775313,
73.2663646146311));
#53939=CARTESIAN_POINT('Ctrl Pts',(-3.3193311989464,-3.67227989433378,73.3107071492751));
#53940=CARTESIAN_POINT('Ctrl Pts',(-2.10582746429627,-4.76915184373973,
73.3636274033571));
#53941=CARTESIAN_POINT('Ctrl Pts',(-0.29486236375909,-5.2050336026263,73.416547657439));
#53942=CARTESIAN_POINT('Ctrl Pts',(1.28483881433472,-4.78045902103617,73.469467911521));
#53943=CARTESIAN_POINT('Ctrl Pts',(2.86453999242835,-4.35588443944609,73.522388165603));
#53944=CARTESIAN_POINT('Ctrl Pts',(4.21297724807857,-3.07085351737952,73.5753084196849));
#53945=CARTESIAN_POINT('Ctrl Pts',(4.71308509882384,-1.51341603066432,73.6282286737669));
#53946=CARTESIAN_POINT('Ctrl Pts',(5.21319294956918,0.0440214560510618,
73.6811489278489));
#53947=CARTESIAN_POINT('Ctrl Pts',(4.8649713954092,1.87386550741532,73.7340691819308));
#53948=CARTESIAN_POINT('Ctrl Pts',(3.82777193781054,3.13875153886656,73.7869894360128));
#53949=CARTESIAN_POINT('Ctrl Pts',(2.790572480212,4.40363757031766,73.8399096900947));
#53950=CARTESIAN_POINT('Ctrl Pts',(1.06439511917504,5.10356558185611,73.8928299441767));
#53951=CARTESIAN_POINT('Ctrl Pts',(-0.560835021503018,4.91823782561222,
73.9457501982587));
#53952=CARTESIAN_POINT('Ctrl Pts',(-2.18606516218117,4.73291006936832,73.9986704523406));
#53953=CARTESIAN_POINT('Ctrl Pts',(-3.71034808250029,3.662326545342,74.0515907064226));
#53954=CARTESIAN_POINT('Ctrl Pts',(-4.43614863820842,2.1964026248274,74.1045109605045));
#53955=CARTESIAN_POINT('Ctrl Pts',(-4.77065068257367,1.52079753684611,74.1289004887841));
#53956=CARTESIAN_POINT('Ctrl Pts',(-4.9355517737741,0.761220515306077,74.1532900170636));
#53957=CARTESIAN_POINT('Ctrl Pts',(-4.93410780896188,0.00104985362950368,
74.1776795453432));
#53958=CARTESIAN_POINT('Origin',(0.,0.,16.));
#53959=CARTESIAN_POINT('',(-4.94084634488987,-0.00449823523784309,75.3223204546568));
#53960=CARTESIAN_POINT('',(-4.94163609422309,-0.00451829382380276,75.1776795453432));
#53961=CARTESIAN_POINT('',(-4.942,-6.05220448138622E-16,16.));
#53962=CARTESIAN_POINT('Ctrl Pts',(-4.94084634488987,-0.00449823523784309,
75.3223204546568));
#53963=CARTESIAN_POINT('Ctrl Pts',(-4.92989311437387,1.21777170867941,75.2829696921977));
#53964=CARTESIAN_POINT('Ctrl Pts',(-4.47139568953686,2.44738194782565,75.2436189297386));
#53965=CARTESIAN_POINT('Ctrl Pts',(-3.64967329880456,3.34417154871685,75.2042681672795));
#53966=CARTESIAN_POINT('Ctrl Pts',(-2.54459286363954,4.55020494099322,75.1513479131975));
#53967=CARTESIAN_POINT('Ctrl Pts',(-0.782591300857919,5.15430584099797,
75.0984276591155));
#53968=CARTESIAN_POINT('Ctrl Pts',(0.83001256389233,4.88002845063787,75.0455074050336));
#53969=CARTESIAN_POINT('Ctrl Pts',(2.44261642864267,4.60575106027776,74.9925871509516));
#53970=CARTESIAN_POINT('Ctrl Pts',(3.90582259536151,3.45309537955268,74.9396668968697));
#53971=CARTESIAN_POINT('Ctrl Pts',(4.55004557505128,1.94953425212549,74.8867466427877));
#53972=CARTESIAN_POINT('Ctrl Pts',(5.19426855474108,0.445973124698207,74.8338263887057));
#53973=CARTESIAN_POINT('Ctrl Pts',(5.01950834740155,-1.40849344943142,74.7809061346238));
#53974=CARTESIAN_POINT('Ctrl Pts',(4.10573789297132,-2.76523324323168,74.7279858805418));
#53975=CARTESIAN_POINT('Ctrl Pts',(3.19196743854115,-4.12197303703186,74.6750656264599));
#53976=CARTESIAN_POINT('Ctrl Pts',(1.53918673702048,-4.98098605050295,74.6221453723779));
#53977=CARTESIAN_POINT('Ctrl Pts',(-0.0962665201530125,-4.94917480923354,
74.5692251182959));
#53978=CARTESIAN_POINT('Ctrl Pts',(-1.73171977732641,-4.91736356796412,
74.516304864214));
#53979=CARTESIAN_POINT('Ctrl Pts',(-3.34984559015253,-3.99472807195434,
74.463384610132));
#53980=CARTESIAN_POINT('Ctrl Pts',(-4.21016487353403,-2.60348041531225,
74.4104643560501));
#53981=CARTESIAN_POINT('Ctrl Pts',(-4.68781373971693,-1.8310603631163,74.3810830555857));
#53982=CARTESIAN_POINT('Ctrl Pts',(-4.93187137749265,-0.914192241399431,
74.3517017551212));
#53983=CARTESIAN_POINT('Ctrl Pts',(-4.93430944804537,0.00146807591443893,
74.3223204546568));
#53984=CARTESIAN_POINT('Ctrl Pts',(-4.93410780896188,0.00104985362950368,
74.1776795453432));
#53985=CARTESIAN_POINT('Ctrl Pts',(-4.93241866747241,-0.888193286408816,
74.2062102711456));
#53986=CARTESIAN_POINT('Ctrl Pts',(-4.70309992547236,-1.77824877440845,
74.234740996948));
#53987=CARTESIAN_POINT('Ctrl Pts',(-4.25136351730091,-2.53564734819139,
74.2632717227504));
#53988=CARTESIAN_POINT('Ctrl Pts',(-3.41345964958825,-3.94050908369249,
74.3161919768324));
#53989=CARTESIAN_POINT('Ctrl Pts',(-1.8103337230659,-4.88896823769192,74.3691122309144));
#53990=CARTESIAN_POINT('Ctrl Pts',(-0.175600645770052,-4.94699541578848,
74.4220324849964));
#53991=CARTESIAN_POINT('Ctrl Pts',(1.45913243152579,-5.00502259388504,74.4749527390783));
#53992=CARTESIAN_POINT('Ctrl Pts',(3.12547265959522,-4.17261779607872,74.5278729931603));
#53993=CARTESIAN_POINT('Ctrl Pts',(4.06087730056111,-2.83070217091354,74.5807932472422));
#53994=CARTESIAN_POINT('Ctrl Pts',(4.99628194152704,-1.48878654574829,74.6337135013242));
#53995=CARTESIAN_POINT('Ctrl Pts',(5.20075099538943,0.36263990677569,74.6866337554061));
#53996=CARTESIAN_POINT('Ctrl Pts',(4.58071630030657,1.87633616570506,74.7395540094881));
#53997=CARTESIAN_POINT('Ctrl Pts',(3.96068160522376,3.39003242463435,74.7924742635701));
#53998=CARTESIAN_POINT('Ctrl Pts',(2.51614316119567,4.56599848996891,74.8453945176521));
#53999=CARTESIAN_POINT('Ctrl Pts',(0.908143822210297,4.86609433003599,74.898314771734));
#54000=CARTESIAN_POINT('Ctrl Pts',(-0.699855516775171,5.16619017010308,
74.951235025816));
#54001=CARTESIAN_POINT('Ctrl Pts',(-2.47131575071806,4.59041578490263,75.0041552798979));
#54002=CARTESIAN_POINT('Ctrl Pts',(-3.59558962158726,3.4022543267312,75.0570755339799));
#54003=CARTESIAN_POINT('Ctrl Pts',(-4.44965416990239,2.49965701001681,75.097276871101));
#54004=CARTESIAN_POINT('Ctrl Pts',(-4.93023943833446,1.2436624400959,75.1374782082221));
#54005=CARTESIAN_POINT('Ctrl Pts',(-4.94163609422309,-0.00451829382380276,
75.1776795453432));
#54006=CARTESIAN_POINT('Origin',(0.,0.,16.));
#54007=CARTESIAN_POINT('',(-4.949709811623,0.00127385101247733,76.3223204546568));
#54008=CARTESIAN_POINT('',(-4.94936999019276,0.00173199160742904,76.1776795453431));
#54009=CARTESIAN_POINT('',(-4.942,-6.05220448138622E-16,16.));
#54010=CARTESIAN_POINT('Ctrl Pts',(-4.949709811623,0.00127385101247733,
76.3223204546568));
#54011=CARTESIAN_POINT('Ctrl Pts',(-4.94994903879905,0.0705988515890139,
76.3200781374381));
#54012=CARTESIAN_POINT('Ctrl Pts',(-4.94861862980554,0.139914463982202,
76.3178358202194));
#54013=CARTESIAN_POINT('Ctrl Pts',(-4.94569000143091,0.209162484687126,
76.3155935030007));
#54014=CARTESIAN_POINT('Ctrl Pts',(-4.87657232423312,1.84346418821971,76.2626732489188));
#54015=CARTESIAN_POINT('Ctrl Pts',(-3.91725763853945,3.44011779449909,76.2097529948368));
#54016=CARTESIAN_POINT('Ctrl Pts',(-2.50674299584768,4.26847022808205,76.1568327407548));
#54017=CARTESIAN_POINT('Ctrl Pts',(-1.09622835315598,5.09682266166495,76.1039124866729));
#54018=CARTESIAN_POINT('Ctrl Pts',(0.765486246533761,5.15687392255156,76.0509922325909));
#54019=CARTESIAN_POINT('Ctrl Pts',(2.22645176899709,4.4211436366153,75.9980719785089));
#54020=CARTESIAN_POINT('Ctrl Pts',(3.68741729146043,3.68541335067904,75.9451517244269));
#54021=CARTESIAN_POINT('Ctrl Pts',(4.74763373669735,2.15390151791992,75.892231470345));
#54022=CARTESIAN_POINT('Ctrl Pts',(4.92192986700097,0.527451343327534,75.8393112162631));
#54023=CARTESIAN_POINT('Ctrl Pts',(5.09622599730458,-1.09899883126485,75.7863909621811));
#54024=CARTESIAN_POINT('Ctrl Pts',(4.38460181267489,-2.8203873476905,75.7334707080991));
#54025=CARTESIAN_POINT('Ctrl Pts',(3.1127074084203,-3.84898053058463,75.6805504540171));
#54026=CARTESIAN_POINT('Ctrl Pts',(1.84081300416571,-4.87757371347876,75.6276301999351));
#54027=CARTESIAN_POINT('Ctrl Pts',(0.00864838028622472,-5.21337156284137,
75.5747099458532));
#54028=CARTESIAN_POINT('Ctrl Pts',(-1.54535994923236,-4.70270785426469,
75.5217896917713));
#54029=CARTESIAN_POINT('Ctrl Pts',(-3.09936827875094,-4.19204414568801,
75.4688694376893));
#54030=CARTESIAN_POINT('Ctrl Pts',(-4.37522031390861,-2.83491887917204,
75.4159491836074));
#54031=CARTESIAN_POINT('Ctrl Pts',(-4.78906667771331,-1.25237330364,75.3630289295254));
#54032=CARTESIAN_POINT('Ctrl Pts',(-4.89518266041626,-0.846586534424758,
75.3494594379025));
#54033=CARTESIAN_POINT('Ctrl Pts',(-4.94462339418807,-0.425978804568305,
75.3358899462797));
#54034=CARTESIAN_POINT('Ctrl Pts',(-4.94084634488987,-0.00449823523784309,
75.3223204546568));
#54035=CARTESIAN_POINT('Ctrl Pts',(-4.94163609422309,-0.00451829382380276,
75.1776795453432));
#54036=CARTESIAN_POINT('Ctrl Pts',(-4.94524177329398,-0.3994182708838,75.1903984623041));
#54037=CARTESIAN_POINT('Ctrl Pts',(-4.90188327382623,-0.793536109632625,
75.2031173792649));
#54038=CARTESIAN_POINT('Ctrl Pts',(-4.80852961499291,-1.17543275960954,
75.2158362962258));
#54039=CARTESIAN_POINT('Ctrl Pts',(-4.42010822973382,-2.76440985663659,
75.2687565503078));
#54040=CARTESIAN_POINT('Ctrl Pts',(-3.16617795142011,-4.14181551954833,
75.3216768043897));
#54041=CARTESIAN_POINT('Ctrl Pts',(-1.62055642630759,-4.6773278802945,75.3745970584716));
#54042=CARTESIAN_POINT('Ctrl Pts',(-0.0749349011951517,-5.21284024104065,
75.4275173125536));
#54043=CARTESIAN_POINT('Ctrl Pts',(1.76237787071597,-4.90645929962131,75.4804375666356));
#54044=CARTESIAN_POINT('Ctrl Pts',(3.05059950427476,-3.89838965409382,75.5333578207175));
#54045=CARTESIAN_POINT('Ctrl Pts',(4.3388211378337,-2.8903200085662,75.5862780747995));
#54046=CARTESIAN_POINT('Ctrl Pts',(5.07795163304007,-1.18056165893029,75.6391983288815));
#54047=CARTESIAN_POINT('Ctrl Pts',(4.92975358676999,0.448473861396107,75.6921185829634));
#54048=CARTESIAN_POINT('Ctrl Pts',(4.78155554049993,2.07750938172241,75.7450388370454));
#54049=CARTESIAN_POINT('Ctrl Pts',(3.74602895275332,3.62582207273939,75.7979590911274));
#54050=CARTESIAN_POINT('Ctrl Pts',(2.29704660536897,4.38488040012382,75.8508793452094));
#54051=CARTESIAN_POINT('Ctrl Pts',(0.848064257984615,5.14393872750825,75.9037995992913));
#54052=CARTESIAN_POINT('Ctrl Pts',(-1.0143738490375,5.11374269126039,75.9567198533733));
#54053=CARTESIAN_POINT('Ctrl Pts',(-2.43798759346781,4.30811045874223,76.0096401074552));
#54054=CARTESIAN_POINT('Ctrl Pts',(-3.86160133789813,3.50247822622406,76.0625603615372));
#54055=CARTESIAN_POINT('Ctrl Pts',(-4.84639071973656,1.92140979743563,76.1154806156192));
#54056=CARTESIAN_POINT('Ctrl Pts',(-4.94170107746221,0.28842623257243,76.1684008697011));
#54057=CARTESIAN_POINT('Ctrl Pts',(-4.94727143302206,0.192987506953041,
76.1714937615818));
#54058=CARTESIAN_POINT('Ctrl Pts',(-4.94980355369306,0.0973714523878282,
76.1745866534625));
#54059=CARTESIAN_POINT('Ctrl Pts',(-4.94936999019276,0.00173199160742904,
76.1776795453431));
#54060=CARTESIAN_POINT('Origin',(0.,0.,16.));
#54061=CARTESIAN_POINT('',(-4.93710573305067,0.00369191742993435,77.3223204546568));
#54062=CARTESIAN_POINT('',(-4.93651943436554,0.00342058198068374,77.1776795453431));
#54063=CARTESIAN_POINT('',(-4.942,-6.05220448138622E-16,16.));
#54064=CARTESIAN_POINT('Ctrl Pts',(-4.93710573305067,0.00369191742993435,
77.3223204546568));
#54065=CARTESIAN_POINT('Ctrl Pts',(-4.94100558540341,0.565545404544723,
77.3042663285965));
#54066=CARTESIAN_POINT('Ctrl Pts',(-4.85249197896959,1.12620708123838,77.2862122025363));
#54067=CARTESIAN_POINT('Ctrl Pts',(-4.66622450050179,1.65225526059718,77.2681580764761));
#54068=CARTESIAN_POINT('Ctrl Pts',(-4.12023726994686,3.19420767735372,77.2152378223941));
#54069=CARTESIAN_POINT('Ctrl Pts',(-2.73435528454182,4.43876323142188,77.1623175683121));
#54070=CARTESIAN_POINT('Ctrl Pts',(-1.14277930696628,4.81639429353784,77.1093973142302));
#54071=CARTESIAN_POINT('Ctrl Pts',(0.448796670609252,5.1940253556538,77.0564770601482));
#54072=CARTESIAN_POINT('Ctrl Pts',(2.24606664035538,4.70473192581759,77.0035568060662));
#54073=CARTESIAN_POINT('Ctrl Pts',(3.42657241495318,3.57242215035347,76.9506365519843));
#54074=CARTESIAN_POINT('Ctrl Pts',(4.60707818955111,2.44011237488923,76.8977162979023));
#54075=CARTESIAN_POINT('Ctrl Pts',(5.1708197690006,0.664786253797156,76.8447960438203));
#54076=CARTESIAN_POINT('Ctrl Pts',(4.85982039669027,-0.941139865890017,
76.7918757897384));
#54077=CARTESIAN_POINT('Ctrl Pts',(4.54882102437996,-2.54706598557701,76.7389555356564));
#54078=CARTESIAN_POINT('Ctrl Pts',(3.36308070030987,-3.983592103859,76.6860352815744));
#54079=CARTESIAN_POINT('Ctrl Pts',(1.84521230622943,-4.59334192937927,76.6331150274925));
#54080=CARTESIAN_POINT('Ctrl Pts',(0.327343912148982,-5.20309175489953,
76.5801947734105));
#54081=CARTESIAN_POINT('Ctrl Pts',(-1.52265255194192,-4.98606528765813,
76.5272745193286));
#54082=CARTESIAN_POINT('Ctrl Pts',(-2.85819044963632,-4.04157715364459,
76.4743542652466));
#54083=CARTESIAN_POINT('Ctrl Pts',(-4.13713943489684,-3.13710851769457,
76.4236763283833));
#54084=CARTESIAN_POINT('Ctrl Pts',(-4.94430311018814,-1.56551963073416,
76.3729983915201));
#54085=CARTESIAN_POINT('Ctrl Pts',(-4.949709811623,0.00127385101247733,
76.3223204546568));
#54086=CARTESIAN_POINT('Ctrl Pts',(-4.94936999019276,0.00173199160742904,
76.1776795453431));
#54087=CARTESIAN_POINT('Ctrl Pts',(-4.9423851596845,-1.5390467478049,76.2275069075444));
#54088=CARTESIAN_POINT('Ctrl Pts',(-4.16568308583621,-3.08590036450939,
76.2773342697457));
#54089=CARTESIAN_POINT('Ctrl Pts',(-2.92261878913845,-3.99523449174163,
76.327161631947));
#54090=CARTESIAN_POINT('Ctrl Pts',(-1.60239480947616,-4.96101295025462,
76.380081886029));
#54091=CARTESIAN_POINT('Ctrl Pts',(0.243884483461281,-5.20767116634268,
76.4330021401109));
#54092=CARTESIAN_POINT('Ctrl Pts',(1.77133348755807,-4.62233457318728,76.4859223941929));
#54093=CARTESIAN_POINT('Ctrl Pts',(3.29878249165486,-4.03699798003188,76.5388426482749));
#54094=CARTESIAN_POINT('Ctrl Pts',(4.507401206911,-2.61966657763301,76.5917629023568));
#54095=CARTESIAN_POINT('Ctrl Pts',(4.84410725035561,-1.01893286220407,76.6446831564388));
#54096=CARTESIAN_POINT('Ctrl Pts',(5.18081329380023,0.581800853224953,76.6976034105207));
#54097=CARTESIAN_POINT('Ctrl Pts',(4.64560666543322,2.36593688168406,76.7505236646027));
#54098=CARTESIAN_POINT('Ctrl Pts',(3.483406092445,3.51702732797801,76.8034439186847));
#54099=CARTESIAN_POINT('Ctrl Pts',(2.32120551945685,4.6681177742719,76.8563641727667));
#54100=CARTESIAN_POINT('Ctrl Pts',(0.532011001847567,5.1861626384007,76.9092844268486));
#54101=CARTESIAN_POINT('Ctrl Pts',(-1.06541472329578,4.83409667859588,76.9622046809306));
#54102=CARTESIAN_POINT('Ctrl Pts',(-2.66284044843913,4.48203071879105,77.0151249350126));
#54103=CARTESIAN_POINT('Ctrl Pts',(-4.06849738111654,3.2598539350526,77.0680451890945));
#54104=CARTESIAN_POINT('Ctrl Pts',(-4.63913544075982,1.72685308955721,77.1209654431764));
#54105=CARTESIAN_POINT('Ctrl Pts',(-4.84298445708464,1.17921924512925,77.1398701438987));
#54106=CARTESIAN_POINT('Ctrl Pts',(-4.94027400061573,0.591920131780996,
77.1587748446209));
#54107=CARTESIAN_POINT('Ctrl Pts',(-4.93651943436554,0.00342058198068374,
77.1776795453431));
#54108=CARTESIAN_POINT('Origin',(0.,0.,16.));
#54109=CARTESIAN_POINT('',(-4.93642136366389,-0.0033694929564293,78.3223204546568));
#54110=CARTESIAN_POINT('',(-4.93699915860479,-0.00364661157755484,78.1776795453431));
#54111=CARTESIAN_POINT('',(-4.942,-6.05220448138622E-16,16.));
#54112=CARTESIAN_POINT('Ctrl Pts',(-4.93642136366389,-0.0033694929564293,
78.3223204546568));
#54113=CARTESIAN_POINT('Ctrl Pts',(-4.92980420575396,1.05092284524382,78.288454519755));
#54114=CARTESIAN_POINT('Ctrl Pts',(-4.59907343284897,2.10900469043804,78.2545885848532));
#54115=CARTESIAN_POINT('Ctrl Pts',(-3.975312192884,2.94965955736624,78.2207226499514));
#54116=CARTESIAN_POINT('Ctrl Pts',(-3.00059812102546,4.26330021964482,78.1678023958694));
#54117=CARTESIAN_POINT('Ctrl Pts',(-1.31034971100207,5.04601837903923,78.1148821417875));
#54118=CARTESIAN_POINT('Ctrl Pts',(0.321949550104491,4.93963025159188,78.0619618877055));
#54119=CARTESIAN_POINT('Ctrl Pts',(1.95424881121096,4.83324212414454,78.0090416336236));
#54120=CARTESIAN_POINT('Ctrl Pts',(3.52859892340051,3.83774770985554,77.9561213795416));
#54121=CARTESIAN_POINT('Ctrl Pts',(4.32455323076013,2.40870045658987,77.9032011254596));
#54122=CARTESIAN_POINT('Ctrl Pts',(5.12050753811972,0.979653203324283,77.8502808713777));
#54123=CARTESIAN_POINT('Ctrl Pts',(5.13806604064937,-0.882946888918111,
77.7973606172957));
#54124=CARTESIAN_POINT('Ctrl Pts',(4.36919369942578,-2.32674557099659,77.7444403632137));
#54125=CARTESIAN_POINT('Ctrl Pts',(3.60032135820212,-3.77054425307524,77.6915201091318));
#54126=CARTESIAN_POINT('Ctrl Pts',(2.04501817322514,-4.79554152499005,77.6385998550498));
#54127=CARTESIAN_POINT('Ctrl Pts',(0.415014635617477,-4.93268298063817,
77.5856796009678));
#54128=CARTESIAN_POINT('Ctrl Pts',(-1.21498890199009,-5.06982443628629,
77.5327593468859));
#54129=CARTESIAN_POINT('Ctrl Pts',(-2.91969279222824,-4.3191100756678,77.4798390928039));
#54130=CARTESIAN_POINT('Ctrl Pts',(-3.91899849949491,-3.02407825563606,
77.4269188387219));
#54131=CARTESIAN_POINT('Ctrl Pts',(-4.57738386303512,-2.17085587390878,
77.3920527107002));
#54132=CARTESIAN_POINT('Ctrl Pts',(-4.92957433823582,-1.08135952985832,
77.3571865826785));
#54133=CARTESIAN_POINT('Ctrl Pts',(-4.93710573305067,0.00369191742993435,
77.3223204546568));
#54134=CARTESIAN_POINT('Ctrl Pts',(-4.93651943436554,0.00342058198068374,
77.1776795453431));
#54135=CARTESIAN_POINT('Ctrl Pts',(-4.92976377869543,-1.05547678606275,
77.2116950987028));
#54136=CARTESIAN_POINT('Ctrl Pts',(-4.59587353108828,-2.11826061804498,
77.2457106520626));
#54137=CARTESIAN_POINT('Ctrl Pts',(-3.96697769860343,-2.96085919445861,
77.2797262054223));
#54138=CARTESIAN_POINT('Ctrl Pts',(-2.98856271019464,-4.27174572572668,
77.3326464595043));
#54139=CARTESIAN_POINT('Ctrl Pts',(-1.29611354676788,-5.0496938810105,77.3855667135863));
#54140=CARTESIAN_POINT('Ctrl Pts',(0.335879206226305,-4.93870270308427,
77.4384869676682));
#54141=CARTESIAN_POINT('Ctrl Pts',(1.96787195922058,-4.82771152515804,77.4914072217502));
#54142=CARTESIAN_POINT('Ctrl Pts',(3.53940830178236,-3.82778101402163,77.5443274758322));
#54143=CARTESIAN_POINT('Ctrl Pts',(4.33132920195393,-2.39649464320875,77.5972477299141));
#54144=CARTESIAN_POINT('Ctrl Pts',(5.12325010212551,-0.96520827239587,77.6501679839961));
#54145=CARTESIAN_POINT('Ctrl Pts',(5.13555555990697,0.897433958093309,77.7030882380781));
#54146=CARTESIAN_POINT('Ctrl Pts',(4.36261440987998,2.33905851601337,77.75600849216));
#54147=CARTESIAN_POINT('Ctrl Pts',(3.58967325985303,3.78068307393336,77.808928746242));
#54148=CARTESIAN_POINT('Ctrl Pts',(2.03148550201762,4.8012899592841,77.8618490003239));
#54149=CARTESIAN_POINT('Ctrl Pts',(0.40110165209169,4.93383387390743,77.9147692544059));
#54150=CARTESIAN_POINT('Ctrl Pts',(-1.22928219783424,5.06637778853077,77.9676895084879));
#54151=CARTESIAN_POINT('Ctrl Pts',(-2.93186213985079,4.31085873242671,78.0206097625698));
#54152=CARTESIAN_POINT('Ctrl Pts',(-3.92751158950039,3.01301376448353,78.0735300166518));
#54153=CARTESIAN_POINT('Ctrl Pts',(-4.58067311036902,2.16160728461073,78.1082465262156));
#54154=CARTESIAN_POINT('Ctrl Pts',(-4.92960256861,1.07680737701515,78.1429630357793));
#54155=CARTESIAN_POINT('Ctrl Pts',(-4.93699915860479,-0.00364661157755484,
78.1776795453431));
#54156=CARTESIAN_POINT('Origin',(0.,0.,16.));
#54157=CARTESIAN_POINT('',(-4.94930076406873,-0.0018103975202266,79.3223204546568));
#54158=CARTESIAN_POINT('',(-4.94965689841004,-0.00135584006909748,79.1776795453431));
#54159=CARTESIAN_POINT('',(-4.942,-6.05220448138622E-16,16.));
#54160=CARTESIAN_POINT('Ctrl Pts',(-4.94930076406873,-0.0018103975202266,
79.3223204546568));
#54161=CARTESIAN_POINT('Ctrl Pts',(-4.94206344439878,1.53439887470602,79.2726427109135));
#54162=CARTESIAN_POINT('Ctrl Pts',(-4.17064455342085,3.07688083896746,79.2229649671701));
#54163=CARTESIAN_POINT('Ctrl Pts',(-2.93387463574621,3.9869760667678,79.1732872234267));
#54164=CARTESIAN_POINT('Ctrl Pts',(-1.61637965001588,4.95647401624775,79.1203669693448));
#54165=CARTESIAN_POINT('Ctrl Pts',(0.229196639493549,5.20833819439267,79.0674467152628));
#54166=CARTESIAN_POINT('Ctrl Pts',(1.75829033577168,4.62731170663768,79.0145264611808));
#54167=CARTESIAN_POINT('Ctrl Pts',(3.28738403204981,4.04628521888269,78.9616062070989));
#54168=CARTESIAN_POINT('Ctrl Pts',(4.49999513509664,2.6323680652278,78.9086859530169));
#54169=CARTESIAN_POINT('Ctrl Pts',(4.84121428431374,1.03259032951638,78.8557656989349));
#54170=CARTESIAN_POINT('Ctrl Pts',(5.18243343353085,-0.567187406195048,
78.802845444853));
#54171=CARTESIAN_POINT('Ctrl Pts',(4.65226062891823,-2.35282572396301,78.749925190771));
#54172=CARTESIAN_POINT('Ctrl Pts',(3.49331104303619,-3.50718925806059,78.6970049366891));
#54173=CARTESIAN_POINT('Ctrl Pts',(2.33436145715409,-4.66155279215825,78.6440846826071));
#54174=CARTESIAN_POINT('Ctrl Pts',(0.546635090002505,-5.18464154258545,
78.5911644285251));
#54175=CARTESIAN_POINT('Ctrl Pts',(-1.05177716940348,-4.83708210816974,
78.5382441744432));
#54176=CARTESIAN_POINT('Ctrl Pts',(-2.65018942880937,-4.48952267375405,
78.4853239203612));
#54177=CARTESIAN_POINT('Ctrl Pts',(-4.05928758046969,-3.27131505449554,
78.4324036662792));
#54178=CARTESIAN_POINT('Ctrl Pts',(-4.63424678945294,-1.73992966228502,
78.3794834121973));
#54179=CARTESIAN_POINT('Ctrl Pts',(-4.84126499965602,-1.18854330639521,
78.3604290930171));
#54180=CARTESIAN_POINT('Ctrl Pts',(-4.94014443935181,-0.596556209328453,
78.3413747738369));
#54181=CARTESIAN_POINT('Ctrl Pts',(-4.93642136366389,-0.0033694929564293,
78.3223204546568));
#54182=CARTESIAN_POINT('Ctrl Pts',(-4.93699915860479,-0.00364661157755484,
78.1776795453431));
#54183=CARTESIAN_POINT('Ctrl Pts',(-4.94087759097782,-0.57018710251793,
78.1958832898613));
#54184=CARTESIAN_POINT('Ctrl Pts',(-4.85085250590991,-1.13553269504931,
78.2140870343795));
#54185=CARTESIAN_POINT('Ctrl Pts',(-4.66154625697823,-1.66540857589943,
78.2322907788976));
#54186=CARTESIAN_POINT('Ctrl Pts',(-4.11121251752373,-3.20581506855694,
78.2852110329796));
#54187=CARTESIAN_POINT('Ctrl Pts',(-2.72182608133198,-4.44645717408944,
78.3381312870616));
#54188=CARTESIAN_POINT('Ctrl Pts',(-1.12919140128498,-4.819598117052,78.3910515411436));
#54189=CARTESIAN_POINT('Ctrl Pts',(0.463443278761841,-5.19273906001451,
78.4439717952256));
#54190=CARTESIAN_POINT('Ctrl Pts',(2.25932620266378,-4.69837884040726,78.4968920493075));
#54191=CARTESIAN_POINT('Ctrl Pts',(3.43663391646442,-3.56274424493725,78.5498123033895));
#54192=CARTESIAN_POINT('Ctrl Pts',(4.6139416302652,-2.42710964946711,78.6027325574714));
#54193=CARTESIAN_POINT('Ctrl Pts',(5.17267413396446,-0.65020067813383,78.6556528115534));
#54194=CARTESIAN_POINT('Ctrl Pts',(4.85714690051601,0.954841985584431,78.7085730656353));
#54195=CARTESIAN_POINT('Ctrl Pts',(4.54161966706758,2.5598846493026,78.7614933197173));
#54196=CARTESIAN_POINT('Ctrl Pts',(3.35183269647175,3.99306100540591,78.8144135737993));
#54197=CARTESIAN_POINT('Ctrl Pts',(1.83225067773116,4.59852766487066,78.8673338278812));
#54198=CARTESIAN_POINT('Ctrl Pts',(0.312668658990661,5.20399432433538,78.9202540819632));
#54199=CARTESIAN_POINT('Ctrl Pts',(-1.53670840789443,4.98175128716162,78.9731743360452));
#54200=CARTESIAN_POINT('Ctrl Pts',(-2.86957733213866,4.03350036141105,79.0260945901271));
#54201=CARTESIAN_POINT('Ctrl Pts',(-4.14220208735026,3.12810930583763,79.0766229085325));
#54202=CARTESIAN_POINT('Ctrl Pts',(-4.94395467452422,1.56085664483311,79.1271512269378));
#54203=CARTESIAN_POINT('Ctrl Pts',(-4.94965689841004,-0.00135584006909748,
79.1776795453431));
#54204=CARTESIAN_POINT('Origin',(0.,0.,16.));
#54205=CARTESIAN_POINT('',(-4.94177616066966,0.00451715357047341,80.3223204546568));
#54206=CARTESIAN_POINT('',(-4.94098429374081,0.00450501606805162,80.1776795453432));
#54207=CARTESIAN_POINT('',(-4.942,-6.05220448138622E-16,16.));
#54208=CARTESIAN_POINT('Ctrl Pts',(-4.94177616066966,0.00451715357047341,
80.3223204546568));
#54209=CARTESIAN_POINT('Ctrl Pts',(-4.94534763047119,0.394743465756727,
80.3097511561539));
#54210=CARTESIAN_POINT('Ctrl Pts',(-4.90301618269456,0.784203971238864,
80.2971818576509));
#54211=CARTESIAN_POINT('Ctrl Pts',(-4.81182542362119,1.16186687182505,80.284612559148));
#54212=CARTESIAN_POINT('Ctrl Pts',(-4.42788688170829,2.75193306777578,80.231692305066));
#54213=CARTESIAN_POINT('Ctrl Pts',(-3.17784621930909,4.13286961482545,80.178772050984));
#54214=CARTESIAN_POINT('Ctrl Pts',(-1.63374113503097,4.67273885841708,80.125851796902));
#54215=CARTESIAN_POINT('Ctrl Pts',(-0.0896360507527699,5.21260810200875,
80.07293154282));
#54216=CARTESIAN_POINT('Ctrl Pts',(1.74853345540447,4.91141004214231,80.0200112887381));
#54217=CARTESIAN_POINT('Ctrl Pts',(3.03959294361313,3.90697751111939,79.9670910346562));
#54218=CARTESIAN_POINT('Ctrl Pts',(4.33065243182171,2.90254498009653,79.9141707805742));
#54219=CARTESIAN_POINT('Ctrl Pts',(5.0746019020818,1.1948779779175,79.8612505264923));
#54220=CARTESIAN_POINT('Ctrl Pts',(4.93099871468662,-0.43456899453677,79.8083302724103));
#54221=CARTESIAN_POINT('Ctrl Pts',(4.78739552729143,-2.06401596699104,79.7554100183283));
#54222=CARTESIAN_POINT('Ctrl Pts',(3.7562396822408,-3.61524290972046,79.7024897642464));
#54223=CARTESIAN_POINT('Ctrl Pts',(2.30940384276248,-4.37838468231013,79.6495695101644));
#54224=CARTESIAN_POINT('Ctrl Pts',(0.86256800328416,-5.14152645489981,79.5966492560824));
#54225=CARTESIAN_POINT('Ctrl Pts',(-0.999947830621951,-5.1165830573498,
79.5437290020005));
#54226=CARTESIAN_POINT('Ctrl Pts',(-2.4258279677168,-4.31496896933192,79.4908087479185));
#54227=CARTESIAN_POINT('Ctrl Pts',(-3.85170810481173,-3.51335488131399,
79.4378884938365));
#54228=CARTESIAN_POINT('Ctrl Pts',(-4.84095254509543,-1.93507010282805,
79.3849682397546));
#54229=CARTESIAN_POINT('Ctrl Pts',(-4.9408679242616,-0.302361853177563,
79.3320479856726));
#54230=CARTESIAN_POINT('Ctrl Pts',(-4.94698990261473,-0.202323153982769,
79.328805475334));
#54231=CARTESIAN_POINT('Ctrl Pts',(-4.94977315033439,-0.10208013749047,
79.3255629649954));
#54232=CARTESIAN_POINT('Ctrl Pts',(-4.94930076406873,-0.0018103975202266,
79.3223204546568));
#54233=CARTESIAN_POINT('Ctrl Pts',(-4.94965689841004,-0.00135584006909748,
79.1776795453431));
#54234=CARTESIAN_POINT('Ctrl Pts',(-4.9499268332343,-0.0753086628631314,
79.1800714810198));
#54235=CARTESIAN_POINT('Ctrl Pts',(-4.94841287075996,-0.149250190949008,
79.1824634166964));
#54236=CARTESIAN_POINT('Ctrl Pts',(-4.94508051525459,-0.223109677684533,
79.184855352373));
#54237=CARTESIAN_POINT('Ctrl Pts',(-4.87135399252289,-1.85720997670206,
79.237775606455));
#54238=CARTESIAN_POINT('Ctrl Pts',(-3.90754016545605,-3.45115176040958,
79.290695860537));
#54239=CARTESIAN_POINT('Ctrl Pts',(-2.49469496135826,-4.27552292478954,
79.3436161146189));
#54240=CARTESIAN_POINT('Ctrl Pts',(-1.08184975726055,-5.09989408916944,
79.3965363687009));
#54241=CARTESIAN_POINT('Ctrl Pts',(0.780026823868144,-5.15469463422192,
79.4494566227829));
#54242=CARTESIAN_POINT('Ctrl Pts',(2.23891162262289,-4.41484699357874,79.5023768768648));
#54243=CARTESIAN_POINT('Ctrl Pts',(3.69779642137764,-3.67499935293556,79.5552971309468));
#54244=CARTESIAN_POINT('Ctrl Pts',(4.75368943775855,-2.14050352659667,79.6082173850287));
#54245=CARTESIAN_POINT('Ctrl Pts',(4.92339790113362,-0.51356824058747,79.6611376391107));
#54246=CARTESIAN_POINT('Ctrl Pts',(5.0931063645087,1.11336704542182,79.7140578931926));
#54247=CARTESIAN_POINT('Ctrl Pts',(4.37663027487802,2.83274179110132,79.7669781472746));
#54248=CARTESIAN_POINT('Ctrl Pts',(3.10184003337994,3.85774385333563,79.8198984013566));
#54249=CARTESIAN_POINT('Ctrl Pts',(1.82704979188194,4.88274591556987,79.8728186554386));
#54250=CARTESIAN_POINT('Ctrl Pts',(-0.00605460148340203,5.21337529435879,
79.9257389095204));
#54251=CARTESIAN_POINT('Ctrl Pts',(-1.55861657986055,4.69833093636568,79.9786591636024));
#54252=CARTESIAN_POINT('Ctrl Pts',(-3.11117855823778,4.18328657837255,80.0315794176844));
#54253=CARTESIAN_POINT('Ctrl Pts',(-4.38319812162688,2.82256848359726,80.0844996717665));
#54254=CARTESIAN_POINT('Ctrl Pts',(-4.79257969064933,1.23886203404666,80.1374199258484));
#54255=CARTESIAN_POINT('Ctrl Pts',(-4.89639341618109,0.837255124705079,
80.1508397990133));
#54256=CARTESIAN_POINT('Ctrl Pts',(-4.94473415317796,0.421308677192607,
80.1642596721782));
#54257=CARTESIAN_POINT('Ctrl Pts',(-4.94098429374081,0.00450501606805162,
80.1776795453432));
#54258=CARTESIAN_POINT('Origin',(0.,0.,16.));
#54259=CARTESIAN_POINT('',(-4.93407925753408,-0.000975201913082646,81.3223204546568));
#54260=CARTESIAN_POINT('',(-4.93426916398102,-0.00139536187133696,81.1776795453431));
#54261=CARTESIAN_POINT('',(-4.942,-6.05220448138622E-16,16.));
#54262=CARTESIAN_POINT('Ctrl Pts',(-4.93407925753408,-0.000975201913082646,
81.3223204546568));
#54263=CARTESIAN_POINT('Ctrl Pts',(-4.93251895945243,0.883617373199263,
81.2939393473123));
#54264=CARTESIAN_POINT('Ctrl Pts',(-4.70573849196771,1.76895636928203,81.2655582399678));
#54265=CARTESIAN_POINT('Ctrl Pts',(-4.25849767807825,2.52364737255269,81.2371771326233));
#54266=CARTESIAN_POINT('Ctrl Pts',(-3.42455919852679,3.93086658925474,81.1842568785413));
#54267=CARTESIAN_POINT('Ctrl Pts',(-1.8241145504932,4.88384315405391,81.1313366244594));
#54268=CARTESIAN_POINT('Ctrl Pts',(-0.189551647970844,4.94648043642473,
81.0784163703775));
#54269=CARTESIAN_POINT('Ctrl Pts',(1.44501125455142,5.00911771879556,81.0254961162955));
#54270=CARTESIAN_POINT('Ctrl Pts',(3.11369241156233,4.18141571873815,80.9725758622135));
#54271=CARTESIAN_POINT('Ctrl Pts',(4.05287784031979,2.84214351269564,80.9196556081315));
#54272=CARTESIAN_POINT('Ctrl Pts',(4.99206326907725,1.50287130665312,80.8667353540495));
#54273=CARTESIAN_POINT('Ctrl Pts',(5.20175296958118,-0.347971105374417,
80.8138150999676));
#54274=CARTESIAN_POINT('Ctrl Pts',(4.58598973236862,-1.86340996827063,80.7608948458856));
#54275=CARTESIAN_POINT('Ctrl Pts',(3.97022649515609,-3.37884883116675,80.7079745918037));
#54276=CARTESIAN_POINT('Ctrl Pts',(2.52901032022692,-4.5588841449317,80.6550543377218));
#54277=CARTESIAN_POINT('Ctrl Pts',(0.92186374048162,-4.86351372766964,80.6021340836398));
#54278=CARTESIAN_POINT('Ctrl Pts',(-0.685282839263774,-5.16814331040758,
80.5492138295578));
#54279=CARTESIAN_POINT('Ctrl Pts',(-2.45835982382543,-4.59736716211862,
80.4962935754758));
#54280=CARTESIAN_POINT('Ctrl Pts',(-3.58598010539301,-3.41238116554821,
80.4433733213938));
#54281=CARTESIAN_POINT('Ctrl Pts',(-4.44577484147009,-2.5088458719475,80.4030223658148));
#54282=CARTESIAN_POINT('Ctrl Pts',(-4.93031074601031,-1.24821819877227,
80.3626714102358));
#54283=CARTESIAN_POINT('Ctrl Pts',(-4.94177616066966,0.00451715357047341,
80.3223204546568));
#54284=CARTESIAN_POINT('Ctrl Pts',(-4.94098429374081,0.00450501606805162,
80.1776795453432));
#54285=CARTESIAN_POINT('Ctrl Pts',(-4.92994686631264,-1.22232501277905,
80.2171799262602));
#54286=CARTESIAN_POINT('Ctrl Pts',(-4.46760970741441,-2.45658172320469,
80.2566803071772));
#54287=CARTESIAN_POINT('Ctrl Pts',(-3.64022747730309,-3.35445124336543,
80.2961806880942));
#54288=CARTESIAN_POINT('Ctrl Pts',(-2.53175012027843,-4.55736326690124,
80.3491009421762));
#54289=CARTESIAN_POINT('Ctrl Pts',(-0.768051831573162,-5.1564925096469,
80.4020211962582));
#54290=CARTESIAN_POINT('Ctrl Pts',(0.843772115467599,-4.87766827980189,
80.4549414503402));
#54291=CARTESIAN_POINT('Ctrl Pts',(2.45559606250818,-4.59884404995691,80.5078617044222));
#54292=CARTESIAN_POINT('Ctrl Pts',(3.91554566788429,-3.4420663475215,80.5607819585041));
#54293=CARTESIAN_POINT('Ctrl Pts',(4.55552569480652,-1.93669431624669,80.613702212586));
#54294=CARTESIAN_POINT('Ctrl Pts',(5.19550572172878,-0.431322284971791,
80.666622466668));
#54295=CARTESIAN_POINT('Ctrl Pts',(5.01551617019705,1.42264407514254,80.71954272075));
#54296=CARTESIAN_POINT('Ctrl Pts',(4.09792300791601,2.7768014426365,80.7724629748319));
#54297=CARTESIAN_POINT('Ctrl Pts',(3.18032984563491,4.13095881013054,80.8253832289139));
#54298=CARTESIAN_POINT('Ctrl Pts',(1.52513307260442,4.98530718500416,80.8783034829959));
#54299=CARTESIAN_POINT('Ctrl Pts',(-0.110223988510079,4.94888370271273,
80.9312237370779));
#54300=CARTESIAN_POINT('Ctrl Pts',(-1.74558104962448,4.9124602204213,80.9841439911598));
#54301=CARTESIAN_POINT('Ctrl Pts',(-3.36109839882289,3.98526488096493,81.0370642452417));
#54302=CARTESIAN_POINT('Ctrl Pts',(-4.21749062381118,2.59159643244825,81.0899844993237));
#54303=CARTESIAN_POINT('Ctrl Pts',(-4.69053795942863,1.82177259814856,81.1192161813301));
#54304=CARTESIAN_POINT('Ctrl Pts',(-4.93196472022524,0.909620752018895,
81.1484478633366));
#54305=CARTESIAN_POINT('Ctrl Pts',(-4.93426916398102,-0.00139536187133696,
81.1776795453431));
#54306=CARTESIAN_POINT('Origin',(0.,0.,16.));
#54307=CARTESIAN_POINT('',(-4.94535283272668,-0.00400458364991862,82.3223204546568));
#54308=CARTESIAN_POINT('',(-4.94609777444767,-0.00376784846301249,82.1776795453432));
#54309=CARTESIAN_POINT('',(-4.942,-6.05220448138622E-16,16.));
#54310=CARTESIAN_POINT('Ctrl Pts',(-4.94535283272668,-0.00400458364991862,
82.3223204546568));
#54311=CARTESIAN_POINT('Ctrl Pts',(-4.93330953662462,1.36545649397123,82.2781275384708));
#54312=CARTESIAN_POINT('Ctrl Pts',(-4.34046622285376,2.74406818932791,82.2339346222847));
#54313=CARTESIAN_POINT('Ctrl Pts',(-3.32967465270896,3.66290393572493,82.1897417060986));
#54314=CARTESIAN_POINT('Ctrl Pts',(-2.11926920015238,4.76319387708596,82.1368214520167));
#54315=CARTESIAN_POINT('Ctrl Pts',(-0.309540619040862,5.20418124698654,
82.0839011979348));
#54316=CARTESIAN_POINT('Ctrl Pts',(1.27135165523017,4.78406349239674,82.0309809438528));
#54317=CARTESIAN_POINT('Ctrl Pts',(2.85224392950138,4.3639457378069,81.9780606897708));
#54318=CARTESIAN_POINT('Ctrl Pts',(4.20429989693216,3.08272285872646,81.9251404356888));
#54319=CARTESIAN_POINT('Ctrl Pts',(4.7087980958408,1.52670201104665,81.8722201816068));
#54320=CARTESIAN_POINT('Ctrl Pts',(5.21329629474935,-0.0293188366329011,
81.8192999275248));
#54321=CARTESIAN_POINT('Ctrl Pts',(4.87023672513615,-1.86013765291182,81.7663796734429));
#54322=CARTESIAN_POINT('Ctrl Pts',(3.83660868625431,-3.12794378523385,81.713459419361));
#54323=CARTESIAN_POINT('Ctrl Pts',(2.80298064737236,-4.39574991755603,81.660539165279));
#54324=CARTESIAN_POINT('Ctrl Pts',(1.07878413922189,-5.10054336592114,81.607618911197));
#54325=CARTESIAN_POINT('Ctrl Pts',(-0.546962183326737,-4.91979988461579,
81.554698657115));
#54326=CARTESIAN_POINT('Ctrl Pts',(-2.17270850587518,-4.73905640331046,
81.5017784030331));
#54327=CARTESIAN_POINT('Ctrl Pts',(-3.70000464282163,-3.6727759923347,81.4488581489512));
#54328=CARTESIAN_POINT('Ctrl Pts',(-4.42993655576027,-2.20890485254455,
81.3959378948692));
#54329=CARTESIAN_POINT('Ctrl Pts',(-4.7684063275082,-1.53010711570026,81.3713987481318));
#54330=CARTESIAN_POINT('Ctrl Pts',(-4.93542833750884,-0.765820165151225,
81.3468596013943));
#54331=CARTESIAN_POINT('Ctrl Pts',(-4.93407925753408,-0.000975201913082646,
81.3223204546568));
#54332=CARTESIAN_POINT('Ctrl Pts',(-4.93426916398102,-0.00139536187133696,
81.1776795453431));
#54333=CARTESIAN_POINT('Ctrl Pts',(-4.93613662347209,-0.739658417382295,
81.2013681174186));
#54334=CARTESIAN_POINT('Ctrl Pts',(-4.78097132279663,-1.47717563214288,
81.2250566894941));
#54335=CARTESIAN_POINT('Ctrl Pts',(-4.46478101528126,-2.13759905414229,
81.2487452615696));
#54336=CARTESIAN_POINT('Ctrl Pts',(-3.75841208098482,-3.61298453463955,
81.3016655156515));
#54337=CARTESIAN_POINT('Ctrl Pts',(-2.24840711161364,-4.7036139380569,81.3545857697334));
#54338=CARTESIAN_POINT('Ctrl Pts',(-0.625767443036273,-4.91039859255742,
81.4075060238154));
#54339=CARTESIAN_POINT('Ctrl Pts',(0.996872225541001,-5.11718324705793,
81.4604262778974));
#54340=CARTESIAN_POINT('Ctrl Pts',(2.73214659332435,-4.44012315264172,81.5133465319795));
#54341=CARTESIAN_POINT('Ctrl Pts',(3.7859676073568,-3.18905134900772,81.5662667860614));
#54342=CARTESIAN_POINT('Ctrl Pts',(4.83978862138919,-1.9379795453738,81.6191870401434));
#54343=CARTESIAN_POINT('Ctrl Pts',(5.21215628167071,-0.112896032521955,
81.6721072942252));
#54344=CARTESIAN_POINT('Ctrl Pts',(4.7326694596758,1.45101310003748,81.7250275483072));
#54345=CARTESIAN_POINT('Ctrl Pts',(4.25318263768082,3.01492223259719,81.7779478023891));
#54346=CARTESIAN_POINT('Ctrl Pts',(2.92184133340926,4.31765698486456,81.8308680564712));
#54347=CARTESIAN_POINT('Ctrl Pts',(1.34788766110338,4.7630660380761,81.8837883105532));
#54348=CARTESIAN_POINT('Ctrl Pts',(-0.226066011202234,5.20847509128757,
81.9367085646351));
#54349=CARTESIAN_POINT('Ctrl Pts',(-2.04263205154196,4.79655844544351,81.989628818717));
#54350=CARTESIAN_POINT('Ctrl Pts',(-3.27052209643622,3.71581544847434,82.042549072799));
#54351=CARTESIAN_POINT('Ctrl Pts',(-4.31565037405029,2.79593253903751,82.087592563647));
#54352=CARTESIAN_POINT('Ctrl Pts',(-4.93430071630666,1.39150518826543,82.1326360544951));
#54353=CARTESIAN_POINT('Ctrl Pts',(-4.94609777444767,-0.00376784846301249,
82.1776795453432));
#54354=CARTESIAN_POINT('Origin',(0.,0.,16.));
#54355=CARTESIAN_POINT('',(-4.94676006163664,0.00350952918951444,83.3223204546568));
#54356=CARTESIAN_POINT('',(-4.94604776483535,0.00378542647206983,83.1776795453431));
#54357=CARTESIAN_POINT('',(-4.942,-6.05220448138622E-16,16.));
#54358=CARTESIAN_POINT('Ctrl Pts',(-4.94676006163664,0.00350952918951444,
83.3223204546568));
#54359=CARTESIAN_POINT('Ctrl Pts',(-4.94852531327494,0.222882433779423,
83.3152359837111));
#54360=CARTESIAN_POINT('Ctrl Pts',(-4.93519531289187,0.442039477932862,
83.3081515127655));
#54361=CARTESIAN_POINT('Ctrl Pts',(-4.90603966821321,0.659070530865341,
83.3010670418199));
#54362=CARTESIAN_POINT('Ctrl Pts',(-4.68825006385762,2.28026970762846,83.2481467877379));
#54363=CARTESIAN_POINT('Ctrl Pts',(-3.58740009065817,3.78283999594482,83.1952265336559));
#54364=CARTESIAN_POINT('Ctrl Pts',(-2.10725577029135,4.47918204688364,83.1423062795739));
#54365=CARTESIAN_POINT('Ctrl Pts',(-0.627111449924431,5.1755240978225,83.089386025492));
#54366=CARTESIAN_POINT('Ctrl Pts',(1.23232721760991,5.06563791138373,83.0364657714101));
#54367=CARTESIAN_POINT('Ctrl Pts',(2.62015283567102,4.19980920832437,82.9835455173281));
#54368=CARTESIAN_POINT('Ctrl Pts',(4.00797845373196,3.33398050526512,82.9306252632462));
#54369=CARTESIAN_POINT('Ctrl Pts',(4.9241910223198,1.71220928558549,82.8777050091641));
#54370=CARTESIAN_POINT('Ctrl Pts',(4.94951760585997,0.0766427637077434,
82.8247847550821));
#54371=CARTESIAN_POINT('Ctrl Pts',(4.97484418940015,-1.55892375817019,82.7718645010002));
#54372=CARTESIAN_POINT('Ctrl Pts',(4.10928478789245,-3.20828558224624,82.7189442469183));
#54373=CARTESIAN_POINT('Ctrl Pts',(2.74893264004429,-4.11666951392571,82.6660239928363));
#54374=CARTESIAN_POINT('Ctrl Pts',(1.38858049219621,-5.02505344560512,82.6131037387543));
#54375=CARTESIAN_POINT('Ctrl Pts',(-0.466564401992278,-5.19245948488802,
82.5601834846723));
#54376=CARTESIAN_POINT('Ctrl Pts',(-1.96755942526789,-4.5422800890475,82.5072632305904));
#54377=CARTESIAN_POINT('Ctrl Pts',(-3.4685544485435,-3.89210069320699,82.4543429765084));
#54378=CARTESIAN_POINT('Ctrl Pts',(-4.61539960090623,-2.42433586224305,
82.4014227224265));
#54379=CARTESIAN_POINT('Ctrl Pts',(-4.88328101508674,-0.810657190350331,
82.3485024683445));
#54380=CARTESIAN_POINT('Ctrl Pts',(-4.92745864911638,-0.544537549215846,
82.3397751304486));
#54381=CARTESIAN_POINT('Ctrl Pts',(-4.94773117576294,-0.274449500871191,
82.3310477925527));
#54382=CARTESIAN_POINT('Ctrl Pts',(-4.94535283272668,-0.00400458364991862,
82.3223204546568));
#54383=CARTESIAN_POINT('Ctrl Pts',(-4.94609777444767,-0.00376784846301249,
82.1776795453432));
#54384=CARTESIAN_POINT('Ctrl Pts',(-4.94816072809722,-0.247759491874606,
82.1855563085771));
#54385=CARTESIAN_POINT('Ctrl Pts',(-4.93166636384428,-0.49147120021732,
82.193433071811));
#54386=CARTESIAN_POINT('Ctrl Pts',(-4.89565013237716,-0.732262940926013,
82.201309835045));
#54387=CARTESIAN_POINT('Ctrl Pts',(-4.65367407397507,-2.35002898526266,
82.2542300891269));
#54388=CARTESIAN_POINT('Ctrl Pts',(-3.53050790772224,-3.83599172584166,
82.3071503432088));
#54389=CARTESIAN_POINT('Ctrl Pts',(-2.04012962670993,-4.51015191896435,
82.3600705972908));
#54390=CARTESIAN_POINT('Ctrl Pts',(-0.549751345697456,-5.18431211208712,
82.4129908513727));
#54391=CARTESIAN_POINT('Ctrl Pts',(1.3078390500746,-5.04666975775335,82.4659111054547));
#54392=CARTESIAN_POINT('Ctrl Pts',(2.68257982821446,-4.16021209746218,82.5188313595367));
#54393=CARTESIAN_POINT('Ctrl Pts',(4.05732060635432,-3.273754437171,82.5717516136187));
#54394=CARTESIAN_POINT('Ctrl Pts',(4.94921176686199,-1.63848147092241,82.6246718677007));
#54395=CARTESIAN_POINT('Ctrl Pts',(4.95011028710458,-0.00271908696136483,
82.6775921217826));
#54396=CARTESIAN_POINT('Ctrl Pts',(4.95100880734717,1.63304329699958,82.7305123758646));
#54397=CARTESIAN_POINT('Ctrl Pts',(4.06091468732478,3.26929509867298,82.7834326299465));
#54398=CARTESIAN_POINT('Ctrl Pts',(2.68714860199004,4.15726251102139,82.8363528840285));
#54399=CARTESIAN_POINT('Ctrl Pts',(1.31338251665521,5.04522992336985,82.8892731381104));
#54400=CARTESIAN_POINT('Ctrl Pts',(-0.544055533992037,5.18491294639323,
82.9421933921924));
#54401=CARTESIAN_POINT('Ctrl Pts',(-2.0351735518924,4.51239048126625,82.9951136462744));
#54402=CARTESIAN_POINT('Ctrl Pts',(-3.52629156979259,3.83986801613934,83.0480339003563));
#54403=CARTESIAN_POINT('Ctrl Pts',(-4.651089554946,2.35514006286229,83.1009541544383));
#54404=CARTESIAN_POINT('Ctrl Pts',(-4.8948427284911,0.737640835765265,83.1538744085202));
#54405=CARTESIAN_POINT('Ctrl Pts',(-4.9313919209059,0.495107417134616,83.1618094541278));
#54406=CARTESIAN_POINT('Ctrl Pts',(-4.94813254848979,0.249588896780995,
83.1697444997355));
#54407=CARTESIAN_POINT('Ctrl Pts',(-4.94604776483535,0.00378542647206983,
83.1776795453431));
#54408=CARTESIAN_POINT('Origin',(0.,0.,16.));
#54409=CARTESIAN_POINT('',(-4.93450205841395,0.0017791821159216,84.3223204546568));
#54410=CARTESIAN_POINT('',(-4.93425329604086,0.00136738585504144,84.1776795453431));
#54411=CARTESIAN_POINT('',(-4.942,-6.05220448138622E-16,16.));
#54412=CARTESIAN_POINT('Ctrl Pts',(-4.93450205841395,0.0017791821159216,
84.3223204546568));
#54413=CARTESIAN_POINT('Ctrl Pts',(-4.9368080070955,0.715261896051447,84.2994241748696));
#54414=CARTESIAN_POINT('Ctrl Pts',(-4.79225594661696,1.42785481900567,84.2765278950824));
#54415=CARTESIAN_POINT('Ctrl Pts',(-4.49620929648531,2.07068108576527,84.2536316152951));
#54416=CARTESIAN_POINT('Ctrl Pts',(-3.81195560589931,3.55644775544483,84.2007113612132));
#54417=CARTESIAN_POINT('Ctrl Pts',(-2.31839897625278,4.66951227096791,84.1477911071313));
#54418=CARTESIAN_POINT('Ctrl Pts',(-0.699026613519106,4.90050762812279,
84.0948708530493));
#54419=CARTESIAN_POINT('Ctrl Pts',(0.92034574921447,5.13150298527765,84.0419505989674));
#54420=CARTESIAN_POINT('Ctrl Pts',(2.66553384503535,4.48042918406423,83.9890303448854));
#54421=CARTESIAN_POINT('Ctrl Pts',(3.73791967339092,3.24523363926685,83.9361100908034));
#54422=CARTESIAN_POINT('Ctrl Pts',(4.81030550174656,2.01003809446939,83.8831898367214));
#54423=CARTESIAN_POINT('Ctrl Pts',(5.20988906263709,0.190720806087873,83.8302695826395));
#54424=CARTESIAN_POINT('Ctrl Pts',(4.75381130414694,-1.38017403364147,83.7773493285575));
#54425=CARTESIAN_POINT('Ctrl Pts',(4.29773354565674,-2.951068873371,83.7244290744756));
#54426=CARTESIAN_POINT('Ctrl Pts',(2.9859944677857,-4.27354126444818,83.6715088203937));
#54427=CARTESIAN_POINT('Ctrl Pts',(1.41886773993217,-4.74240598011873,83.6185885663117));
#54428=CARTESIAN_POINT('Ctrl Pts',(-0.148258987921171,-5.21127069578923,
83.5656683122296));
#54429=CARTESIAN_POINT('Ctrl Pts',(-1.97077336575683,-4.82652773605328,
83.5127480581476));
#54430=CARTESIAN_POINT('Ctrl Pts',(-3.21466593691877,-3.76424222358033,
83.4598278040656));
#54431=CARTESIAN_POINT('Ctrl Pts',(-4.29203775090064,-2.84416560597453,
83.4139920209293));
#54432=CARTESIAN_POINT('Ctrl Pts',(-4.93533906889132,-1.41581012896607,
83.3681562377931));
#54433=CARTESIAN_POINT('Ctrl Pts',(-4.94676006163664,0.00350952918951444,
83.3223204546568));
#54434=CARTESIAN_POINT('Ctrl Pts',(-4.94604776483535,0.00378542647206983,
83.1776795453431));
#54435=CARTESIAN_POINT('Ctrl Pts',(-4.93422874929891,-1.38971889629444,
83.2226647538174));
#54436=CARTESIAN_POINT('Ctrl Pts',(-4.31736833349613,-2.79238139987207,
83.2676499622918));
#54437=CARTESIAN_POINT('Ctrl Pts',(-3.27460228178232,-3.71222020633235,
83.3126351707661));
#54438=CARTESIAN_POINT('Ctrl Pts',(-2.04790029959144,-4.7943115204161,83.3655554248481));
#54439=CARTESIAN_POINT('Ctrl Pts',(-0.231787973272793,-5.20822364766616,
83.4184756789301));
#54440=CARTESIAN_POINT('Ctrl Pts',(1.34265411435701,-4.76454397765274,83.4713959330121));
#54441=CARTESIAN_POINT('Ctrl Pts',(2.91709620198673,-4.32086430763936,83.524316187094));
#54442=CARTESIAN_POINT('Ctrl Pts',(4.24986805092773,-3.01959284036256,83.577236441176));
#54443=CARTESIAN_POINT('Ctrl Pts',(4.73107261188716,-1.45621146364564,83.630156695258));
#54444=CARTESIAN_POINT('Ctrl Pts',(5.21227717284655,0.107169913071196,83.6830769493399));
#54445=CARTESIAN_POINT('Ctrl Pts',(4.84191444582465,1.93266119922796,83.7359972034218));
#54446=CARTESIAN_POINT('Ctrl Pts',(3.78946863845564,3.18489006691465,83.7889174575038));
#54447=CARTESIAN_POINT('Ctrl Pts',(2.73702283108663,4.43711893460135,83.8418377115857));
#54448=CARTESIAN_POINT('Ctrl Pts',(1.00249394337044,5.11608538381779,83.8947579656677));
#54449=CARTESIAN_POINT('Ctrl Pts',(-0.620372201325573,4.91108329901265,
83.9476782197497));
#54450=CARTESIAN_POINT('Ctrl Pts',(-2.24323834602159,4.70608121420751,84.0005984738317));
#54451=CARTESIAN_POINT('Ctrl Pts',(-3.75444174769753,3.6171105953808,84.0535187279136));
#54452=CARTESIAN_POINT('Ctrl Pts',(-4.4624305684118,2.14250236754745,84.1064389819956));
#54453=CARTESIAN_POINT('Ctrl Pts',(-4.78012570742429,1.48080284317098,84.1301858364447));
#54454=CARTESIAN_POINT('Ctrl Pts',(-4.93608736949663,0.741452199377731,
84.1539326908939));
#54455=CARTESIAN_POINT('Ctrl Pts',(-4.93425329604086,0.00136738585504144,
84.1776795453431));
#54456=CARTESIAN_POINT('Origin',(0.,0.,16.));
#54457=CARTESIAN_POINT('',(-4.93983901057914,-0.00407131671605609,85.3223204546568));
#54458=CARTESIAN_POINT('',(-4.94096920053978,-0.0044629540342261,85.1776795453431));
#54459=CARTESIAN_POINT('',(-4.942,-6.05220448138622E-16,16.));
#54460=CARTESIAN_POINT('Ctrl Pts',(-4.93983901057914,-0.00407131671605609,
85.3223204546568));
#54461=CARTESIAN_POINT('Ctrl Pts',(-4.92935782359351,1.19852489561668,85.283612366028));
#54462=CARTESIAN_POINT('Ctrl Pts',(-4.48753687762877,2.40778661262928,85.2449042773993));
#54463=CARTESIAN_POINT('Ctrl Pts',(-3.69010132050912,3.2995468819145,85.2061961887705));
#54464=CARTESIAN_POINT('Ctrl Pts',(-2.59987718928131,4.51872823916,85.1532759346885));
#54465=CARTESIAN_POINT('Ctrl Pts',(-0.844961773498813,5.14445691330988,
85.1003556806066));
#54466=CARTESIAN_POINT('Ctrl Pts',(0.770932612771407,4.88981272332166,85.0474354265247));
#54467=CARTESIAN_POINT('Ctrl Pts',(2.38682699904172,4.63516853333343,84.9945151724427));
#54468=CARTESIAN_POINT('Ctrl Pts',(3.86370035579973,3.500151479207,84.9415949183607));
#54469=CARTESIAN_POINT('Ctrl Pts',(4.52604489048226,2.00446382425534,84.8886746642787));
#54470=CARTESIAN_POINT('Ctrl Pts',(5.18838942516471,0.508776169303851,84.8357544101967));
#54471=CARTESIAN_POINT('Ctrl Pts',(5.0362051377719,-1.34758208647277,84.7828341561149));
#54472=CARTESIAN_POINT('Ctrl Pts',(4.13896054991356,-2.7152702523835,84.7299139020329));
#54473=CARTESIAN_POINT('Ctrl Pts',(3.24171596205511,-4.08295841829439,84.6769936479509));
#54474=CARTESIAN_POINT('Ctrl Pts',(1.59941107373096,-4.96197649433929,84.6240733938688));
#54475=CARTESIAN_POINT('Ctrl Pts',(-0.0363198163526684,-4.94999030922869,
84.5711531397869));
#54476=CARTESIAN_POINT('Ctrl Pts',(-1.67205070643629,-4.93800412411811,
84.518232885705));
#54477=CARTESIAN_POINT('Ctrl Pts',(-3.30120759827939,-4.03501367785208,
84.4653126316231));
#54478=CARTESIAN_POINT('Ctrl Pts',(-4.17831066843813,-2.65428404280099,
84.4123923775412));
#54479=CARTESIAN_POINT('Ctrl Pts',(-4.67592959505013,-1.87093574279885,
84.3823684032464));
#54480=CARTESIAN_POINT('Ctrl Pts',(-4.93147825958796,-0.9338132749143,84.3523444289516));
#54481=CARTESIAN_POINT('Ctrl Pts',(-4.93450205841395,0.0017791821159216,
84.3223204546568));
#54482=CARTESIAN_POINT('Ctrl Pts',(-4.93425329604086,0.00136738585504144,
84.1776795453431));
#54483=CARTESIAN_POINT('Ctrl Pts',(-4.93200010676076,-0.907838929165127,
84.2068529449759));
#54484=CARTESIAN_POINT('Ctrl Pts',(-4.6915933103023,-1.81815329167953,84.2360263446087));
#54485=CARTESIAN_POINT('Ctrl Pts',(-4.22033403606684,-2.58696080038834,
84.2651997442415));
#54486=CARTESIAN_POINT('Ctrl Pts',(-3.36547444325506,-3.98156990365044,
84.3181199983235));
#54487=CARTESIAN_POINT('Ctrl Pts',(-1.75098101787896,-4.91054227333463,
84.3710402524054));
#54488=CARTESIAN_POINT('Ctrl Pts',(-0.115662974249316,-4.94876105553069,
84.4239605064874));
#54489=CARTESIAN_POINT('Ctrl Pts',(1.51965506938033,-4.98697983772675,84.4768807605693));
#54490=CARTESIAN_POINT('Ctrl Pts',(3.17579773126353,-4.1344450324347,84.5298010146513));
#54491=CARTESIAN_POINT('Ctrl Pts',(4.09487421234139,-2.78129899063739,84.5827212687333));
#54492=CARTESIAN_POINT('Ctrl Pts',(5.01395069341925,-1.42815294884008,84.6356415228152));
#54493=CARTESIAN_POINT('Ctrl Pts',(5.19596099369178,0.425604329462498,84.6885617768972));
#54494=CARTESIAN_POINT('Ctrl Pts',(4.55764242829978,1.93168321282745,84.7414820309791));
#54495=CARTESIAN_POINT('Ctrl Pts',(3.91932386290774,3.43776209619249,84.7944022850611));
#54496=CARTESIAN_POINT('Ctrl Pts',(2.46067643185109,4.59616258461988,84.8473225391431));
#54497=CARTESIAN_POINT('Ctrl Pts',(0.849145831707845,4.87674842560418,84.9002427932251));
#54498=CARTESIAN_POINT('Ctrl Pts',(-0.762384768435213,5.15733426658845,
84.9531630473071));
#54499=CARTESIAN_POINT('Ctrl Pts',(-2.52679853766482,4.5601054601299,85.006083301389));
#54500=CARTESIAN_POINT('Ctrl Pts',(-3.63657003853315,3.35842910333814,85.059003555471));
#54501=CARTESIAN_POINT('Ctrl Pts',(-4.46614045337841,2.46015846561364,85.0985622187617));
#54502=CARTESIAN_POINT('Ctrl Pts',(-4.92991110676884,1.22413577549367,85.1381208820524));
#54503=CARTESIAN_POINT('Ctrl Pts',(-4.94096920053978,-0.0044629540342261,
85.1776795453431));
#54504=CARTESIAN_POINT('Origin',(0.,0.,24.1514101080949));
#54505=CARTESIAN_POINT('',(-4.37008825460381,-0.00360173951420115,85.6514101080948));
#54506=CARTESIAN_POINT('',(-4.37741404908174,0.00054794132368214,85.8485898919049));
#54507=CARTESIAN_POINT('',(-4.372,3.82579154166093E-12,24.1514101080949));
#54508=CARTESIAN_POINT('',(2.54472701347433,-3.56250531650779,85.9999999999999));
#54509=CARTESIAN_POINT('Ctrl Pts',(-4.37008825460381,-0.00360173951420056,
85.6514101080948));
#54510=CARTESIAN_POINT('Ctrl Pts',(-4.37349270028371,-0.394222905349127,
85.665622273548));
#54511=CARTESIAN_POINT('Ctrl Pts',(-4.14658524106498,-2.2356015936124,85.7327546930832));
#54512=CARTESIAN_POINT('Ctrl Pts',(-1.63914477126166,-4.84388062782939,
85.8489513237184));
#54513=CARTESIAN_POINT('Ctrl Pts',(1.44818750565376,-4.33531680853971,85.9509357889001));
#54514=CARTESIAN_POINT('Ctrl Pts',(2.54472701347433,-3.56250531650779,85.9999999999999));
#54515=CARTESIAN_POINT('',(-2.53835875722777,-3.5596515025498,86.));
#54516=CARTESIAN_POINT('Origin',(0.,0.,86.));
#54517=CARTESIAN_POINT('Ctrl Pts',(-4.37741404908174,0.000547941323682409,
85.8485898919049));
#54518=CARTESIAN_POINT('Ctrl Pts',(-4.37702756934774,-0.658293262144059,
85.8725998008956));
#54519=CARTESIAN_POINT('Ctrl Pts',(-4.04502790407186,-2.04740376323306,
85.9230698369273));
#54520=CARTESIAN_POINT('Ctrl Pts',(-3.130164636136,-3.13763950664809,85.973539872959));
#54521=CARTESIAN_POINT('Ctrl Pts',(-2.53835875722777,-3.5596515025498,86.));
#54522=CARTESIAN_POINT('Origin',(0.,0.,24.1514101080949));
#54523=CARTESIAN_POINT('',(-4.3653668553998,0.00157397495328755,84.6514101080948));
#54524=CARTESIAN_POINT('',(-4.37108809080528,-0.00394820619502134,84.8485898919049));
#54525=CARTESIAN_POINT('',(-4.372,3.82579154166093E-12,24.1514101080949));
#54526=CARTESIAN_POINT('Ctrl Pts',(-4.3653668553998,0.00157397495328733,
84.6514101080948));
#54527=CARTESIAN_POINT('Ctrl Pts',(-4.36269181524081,-0.826109194237039,
84.6814340823896));
#54528=CARTESIAN_POINT('Ctrl Pts',(-3.73813921667308,-3.11640593107392,
84.7643783107663));
#54529=CARTESIAN_POINT('Ctrl Pts',(-0.0379465312430282,-5.16730640666113,
84.9002427932251));
#54530=CARTESIAN_POINT('Ctrl Pts',(4.32070804489202,-2.83440452778566,85.059003555471));
#54531=CARTESIAN_POINT('Ctrl Pts',(4.72460304963626,2.09234474027741,85.2177643177169));
#54532=CARTESIAN_POINT('Ctrl Pts',(0.805001482004623,5.10466438453535,85.3765250799626));
#54533=CARTESIAN_POINT('Ctrl Pts',(-3.43558144629758,3.5926517202867,85.5210736767555));
#54534=CARTESIAN_POINT('Ctrl Pts',(-4.3608159459227,1.06028952724385,85.6127020194661));
#54535=CARTESIAN_POINT('Ctrl Pts',(-4.37008825460381,-0.00360173951420056,
85.6514101080948));
#54536=CARTESIAN_POINT('Ctrl Pts',(-4.37108809080528,-0.00394820619502242,
84.8485898919049));
#54537=CARTESIAN_POINT('Ctrl Pts',(-4.37439235100703,-0.371064815037356,
84.8619514826962));
#54538=CARTESIAN_POINT('Ctrl Pts',(-4.16412636077677,-2.18847582560682,
84.9282333275694));
#54539=CARTESIAN_POINT('Ctrl Pts',(-1.63279460579437,-4.90302030367583,
85.0474354265246));
#54540=CARTESIAN_POINT('Ctrl Pts',(3.23428855022947,-4.03017982392474,85.2061961887705));
#54541=CARTESIAN_POINT('Ctrl Pts',(5.13873193725801,0.529582954402255,85.3649569510164));
#54542=CARTESIAN_POINT('Ctrl Pts',(2.34489518331184,4.6077777382683,85.5237177132623));
#54543=CARTESIAN_POINT('Ctrl Pts',(-2.60449736313211,4.46265913321349,85.6824784755082));
#54544=CARTESIAN_POINT('Ctrl Pts',(-4.34126539015093,1.58670061603872,85.7907692017224));
#54545=CARTESIAN_POINT('Ctrl Pts',(-4.37745348944865,0.0677828737684449,
85.8461396738546));
#54546=CARTESIAN_POINT('Ctrl Pts',(-4.37741404908174,0.000547941323682409,
85.8485898919049));
#54547=CARTESIAN_POINT('Origin',(0.,0.,24.1514101080949));
#54548=CARTESIAN_POINT('',(-4.37621104602901,0.00310474739351271,83.6514101080948));
#54549=CARTESIAN_POINT('',(-4.36514678476137,0.00120967441979231,83.8485898919049));
#54550=CARTESIAN_POINT('',(-4.372,3.82579154166093E-12,24.1514101080949));
#54551=CARTESIAN_POINT('Ctrl Pts',(-4.37621104602901,0.00310474739351276,
83.6514101080948));
#54552=CARTESIAN_POINT('Ctrl Pts',(-4.36610732682993,-1.25251353375917,
83.6972458912311));
#54553=CARTESIAN_POINT('Ctrl Pts',(-3.13993685867563,-3.97504379283746,
83.7960019284495));
#54554=CARTESIAN_POINT('Ctrl Pts',(1.4811502559097,-4.9505810809301,83.9476782197498));
#54555=CARTESIAN_POINT('Ctrl Pts',(4.96248771955931,-1.44075755171813,84.1064389819956));
#54556=CARTESIAN_POINT('Ctrl Pts',(3.90199844707087,3.38768549854763,84.2651997442416));
#54557=CARTESIAN_POINT('Ctrl Pts',(-0.729706746127024,5.11562640844579,
84.4239605064874));
#54558=CARTESIAN_POINT('Ctrl Pts',(-3.94395824097378,2.72022390956171,84.5526972944385));
#54559=CARTESIAN_POINT('Ctrl Pts',(-4.36740684075686,0.63276507679951,84.6285138283076));
#54560=CARTESIAN_POINT('Ctrl Pts',(-4.3653668553998,0.00157397495328733,
84.6514101080948));
#54561=CARTESIAN_POINT('Ctrl Pts',(-4.36514678476137,0.00120967441979238,
83.8485898919049));
#54562=CARTESIAN_POINT('Ctrl Pts',(-4.36315347364677,-0.803130675494322,
83.8777632915377));
#54563=CARTESIAN_POINT('Ctrl Pts',(-3.76467753114223,-3.06929475283447,
83.9598569452526));
#54564=CARTESIAN_POINT('Ctrl Pts',(-0.120745397495975,-5.1659971710397,
84.0948708530492));
#54565=CARTESIAN_POINT('Ctrl Pts',(4.27463443926266,-2.90338152834273,84.2536316152952));
#54566=CARTESIAN_POINT('Ctrl Pts',(4.75768727179541,2.01646478129229,84.412392377541));
#54567=CARTESIAN_POINT('Ctrl Pts',(0.886457060193665,5.09084373843816,84.571153139787));
#54568=CARTESIAN_POINT('Ctrl Pts',(-3.40216585276062,3.63920626636618,84.7165523112416));
#54569=CARTESIAN_POINT('Ctrl Pts',(-4.36130541456655,1.08294650151228,84.8090312286142));
#54570=CARTESIAN_POINT('Ctrl Pts',(-4.37108809080528,-0.00394820619502242,
84.8485898919049));
#54571=CARTESIAN_POINT('Origin',(0.,0.,24.1514101080949));
#54572=CARTESIAN_POINT('',(-4.37496612397431,-0.00354270330085218,82.6514101080948));
#54573=CARTESIAN_POINT('',(-4.37558090405915,0.00334882326136696,82.8485898919049));
#54574=CARTESIAN_POINT('',(-4.372,3.82579154166093E-12,24.1514101080949));
#54575=CARTESIAN_POINT('Ctrl Pts',(-4.37496612397431,-0.00354270330085171,
82.6514101080948));
#54576=CARTESIAN_POINT('Ctrl Pts',(-4.37707015387208,-0.242795066330439,
82.6601374459907));
#54577=CARTESIAN_POINT('Ctrl Pts',(-4.25038678075279,-1.93057999813071,
82.7217850379685));
#54578=CARTESIAN_POINT('Ctrl Pts',(-2.05392817541576,-4.74166978382725,
82.8363528840287));
#54579=CARTESIAN_POINT('Ctrl Pts',(2.86960084768762,-4.29737645901297,82.9951136462743));
#54580=CARTESIAN_POINT('Ctrl Pts',(5.16678358952832,0.0800071275065655,
83.1538744085204));
#54581=CARTESIAN_POINT('Ctrl Pts',(2.73516803922529,4.38416562959496,83.312635170766));
#54582=CARTESIAN_POINT('Ctrl Pts',(-2.19975659925683,4.67580205641259,83.4713959330121));
#54583=CARTESIAN_POINT('Ctrl Pts',(-4.27789107195956,1.83931825768632,83.5843209121216));
#54584=CARTESIAN_POINT('Ctrl Pts',(-4.37777269721528,0.197175637492073,
83.6443256371492));
#54585=CARTESIAN_POINT('Ctrl Pts',(-4.37621104602901,0.00310474739351276,
83.6514101080948));
#54586=CARTESIAN_POINT('Ctrl Pts',(-4.37558090405915,0.0033488232613671,
82.8485898919049));
#54587=CARTESIAN_POINT('Ctrl Pts',(-4.36512506919086,-1.22943160958811,
82.8935751003793));
#54588=CARTESIAN_POINT('Ctrl Pts',(-3.17743944272853,-3.93007838737006,
82.9914805629356));
#54589=CARTESIAN_POINT('Ctrl Pts',(1.40159167776471,-4.9736903294079,83.142306279574));
#54590=CARTESIAN_POINT('Ctrl Pts',(4.93874982643145,-1.52013376024582,83.3010670418199));
#54591=CARTESIAN_POINT('Ctrl Pts',(3.95581224496304,3.32469499516411,83.4598278040656));
#54592=CARTESIAN_POINT('Ctrl Pts',(-0.647603556591826,5.12666260907039,
83.6185885663118));
#54593=CARTESIAN_POINT('Ctrl Pts',(-3.92132004033239,2.76762804019117,83.7481759289246));
#54594=CARTESIAN_POINT('Ctrl Pts',(-4.36676931999915,0.655934645021535,
83.8248430374557));
#54595=CARTESIAN_POINT('Ctrl Pts',(-4.36514678476137,0.00120967441979238,
83.8485898919049));
#54596=CARTESIAN_POINT('Origin',(0.,0.,24.1514101080949));
#54597=CARTESIAN_POINT('',(-4.36499281949393,-0.000862724152283187,81.6514101080949));
#54598=CARTESIAN_POINT('',(-4.37562514566675,-0.00333327265474082,81.8485898919049));
#54599=CARTESIAN_POINT('',(-4.372,3.82579154166093E-12,24.1514101080949));
#54600=CARTESIAN_POINT('Ctrl Pts',(-4.36499281949393,-0.000862724152282945,
81.6514101080949));
#54601=CARTESIAN_POINT('Ctrl Pts',(-4.36618629939077,-0.677492060307118,
81.6759492548323));
#54602=CARTESIAN_POINT('Ctrl Pts',(-3.8997785113075,-2.81175799367349,81.7534086556517));
#54603=CARTESIAN_POINT('Ctrl Pts',(-0.57097184883837,-5.13576134197884,
81.8837883105532));
#54604=CARTESIAN_POINT('Ctrl Pts',(4.00502195951943,-3.26524922770216,82.0425490727989));
#54605=CARTESIAN_POINT('Ctrl Pts',(4.91549733690694,1.59371871934676,82.2013098350451));
#54606=CARTESIAN_POINT('Ctrl Pts',(1.32715940311121,4.99406661129702,82.3600705972907));
#54607=CARTESIAN_POINT('Ctrl Pts',(-3.21180689907642,3.88802958864094,82.510104021641));
#54608=CARTESIAN_POINT('Ctrl Pts',(-4.36431187659278,1.20796758228371,82.6072171919088));
#54609=CARTESIAN_POINT('Ctrl Pts',(-4.37496612397431,-0.00354270330085171,
82.6514101080948));
#54610=CARTESIAN_POINT('Ctrl Pts',(-4.37562514566675,-0.00333327265474043,
81.8485898919049));
#54611=CARTESIAN_POINT('Ctrl Pts',(-4.37745016253379,-0.219183427450699,
81.8564666551388));
#54612=CARTESIAN_POINT('Ctrl Pts',(-4.26482187642182,-1.88331740650866,
81.9172636724547));
#54613=CARTESIAN_POINT('Ctrl Pts',(-2.12968395259116,-4.7081313086182,82.0309809438528));
#54614=CARTESIAN_POINT('Ctrl Pts',(2.80033539806548,-4.3428303941221,82.1897417060986));
#54615=CARTESIAN_POINT('Ctrl Pts',(5.16740226597732,-0.00283844241944707,
82.3485024683445));
#54616=CARTESIAN_POINT('Ctrl Pts',(2.80510471878759,4.33975132503298,82.5072632305904));
#54617=CARTESIAN_POINT('Ctrl Pts',(-2.12451031000386,4.71046814615349,82.6660239928362));
#54618=CARTESIAN_POINT('Ctrl Pts',(-4.26384621089875,1.88655500314254,82.7797995466078));
#54619=CARTESIAN_POINT('Ctrl Pts',(-4.37742523310327,0.220801832606586,
82.8406548462974));
#54620=CARTESIAN_POINT('Ctrl Pts',(-4.37558090405915,0.0033488232613671,
82.8485898919049));
#54621=CARTESIAN_POINT('Origin',(0.,0.,24.1514101080949));
#54622=CARTESIAN_POINT('',(-4.37180197783241,0.00399615447510604,80.6514101080948));
#54623=CARTESIAN_POINT('',(-4.3651608225263,-0.00123442373144794,80.8485898919049));
#54624=CARTESIAN_POINT('',(-4.372,3.82579154166093E-12,24.1514101080949));
#54625=CARTESIAN_POINT('Ctrl Pts',(-4.37180197783241,0.00399615447510625,
80.6514101080948));
#54626=CARTESIAN_POINT('Ctrl Pts',(-4.36165896025063,-1.10425130818043,
80.6917610636739));
#54627=CARTESIAN_POINT('Ctrl Pts',(-3.37083349090091,-3.68210362881494,
80.7850322733349));
#54628=CARTESIAN_POINT('Ctrl Pts',(0.962330231331446,-5.07700442602626,
80.9312237370778));
#54629=CARTESIAN_POINT('Ctrl Pts',(4.78729812901886,-1.94520694012218,81.0899844993237));
#54630=CARTESIAN_POINT('Ctrl Pts',(4.2307845491307,2.96690335452649,81.2487452615696));
#54631=CARTESIAN_POINT('Ctrl Pts',(-0.19787228117179,5.16361307382143,81.4075060238155));
#54632=CARTESIAN_POINT('Ctrl Pts',(-3.78889879581372,3.02535473653369,81.541727639324));
#54633=CARTESIAN_POINT('Ctrl Pts',(-4.36361248294727,0.781702783413628,
81.6230290007504));
#54634=CARTESIAN_POINT('Ctrl Pts',(-4.36499281949393,-0.000862724152282945,
81.6514101080949));
#54635=CARTESIAN_POINT('Ctrl Pts',(-4.3651608225263,-0.00123442373144732,
80.8485898919049));
#54636=CARTESIAN_POINT('Ctrl Pts',(-4.36681289312482,-0.654347754103861,
80.8722784639804));
#54637=CARTESIAN_POINT('Ctrl Pts',(-3.92288549979199,-2.76438197736347,
80.9488872901379));
#54638=CARTESIAN_POINT('Ctrl Pts',(-0.653236375128765,-5.12594736724498,
81.0784163703773));
#54639=CARTESIAN_POINT('Ctrl Pts',(3.95215792026738,-3.32903919274863,81.2371771326234));
#54640=CARTESIAN_POINT('Ctrl Pts',(4.94041656702063,1.51470733791976,81.3959378948691));
#54641=CARTESIAN_POINT('Ctrl Pts',(1.40705506422376,4.97214744531344,81.5546986571151));
#54642=CARTESIAN_POINT('Ctrl Pts',(-3.17488990257063,3.9331654538798,81.7055826561271));
#54643=CARTESIAN_POINT('Ctrl Pts',(-4.36518873567112,1.23101187436481,81.8035464010569));
#54644=CARTESIAN_POINT('Ctrl Pts',(-4.37562514566675,-0.00333327265474043,
81.8485898919049));
#54645=CARTESIAN_POINT('Origin',(0.,0.,24.1514101080949));
#54646=CARTESIAN_POINT('',(-4.37845870912757,-0.00160159003492085,79.6514101080949));
#54647=CARTESIAN_POINT('',(-4.37110144318797,0.00398541688994905,79.8485898919049));
#54648=CARTESIAN_POINT('',(-4.372,3.82579154166093E-12,24.1514101080949));
#54649=CARTESIAN_POINT('Ctrl Pts',(-4.37845870912757,-0.00160159003492056,
79.6514101080949));
#54650=CARTESIAN_POINT('Ctrl Pts',(-4.37887661134401,-0.0903064267712891,
79.6546526184335));
#54651=CARTESIAN_POINT('Ctrl Pts',(-4.3362288360819,-1.62633270599671,79.7108153828541));
#54652=CARTESIAN_POINT('Ctrl Pts',(-2.53231305975701,-4.50438053270811,
79.8198984013567));
#54653=CARTESIAN_POINT('Ctrl Pts',(2.41077833593552,-4.57057996659486,79.9786591636024));
#54654=CARTESIAN_POINT('Ctrl Pts',(5.14745176039643,-0.453645004871452,
80.1374199258484));
#54655=CARTESIAN_POINT('Ctrl Pts',(3.1730201027819,4.07847972207792,80.2961806880942));
#54656=CARTESIAN_POINT('Ctrl Pts',(-1.70545647406065,4.87785522859546,80.4549414503402));
#54657=CARTESIAN_POINT('Ctrl Pts',(-4.17984164299754,2.14436901967187,80.573351257007));
#54658=CARTESIAN_POINT('Ctrl Pts',(-4.37496152173606,0.349214575534816,
80.6388408095919));
#54659=CARTESIAN_POINT('Ctrl Pts',(-4.37180197783241,0.00399615447510625,
80.6514101080948));
#54660=CARTESIAN_POINT('Ctrl Pts',(-4.37110144318797,0.00398541688994905,
79.8485898919049));
#54661=CARTESIAN_POINT('Ctrl Pts',(-4.36133704968111,-1.0813445883965,79.888090272822));
#54662=CARTESIAN_POINT('Ctrl Pts',(-3.40435481309659,-3.63610732924809,
79.980510907821));
#54663=CARTESIAN_POINT('Ctrl Pts',(0.880810665839244,-5.09178031191025,
80.125851796902));
#54664=CARTESIAN_POINT('Ctrl Pts',(4.75549683016874,-2.02170820645871,80.2846125591479));
#54665=CARTESIAN_POINT('Ctrl Pts',(4.27780703699033,2.89869300342805,80.4433733213939));
#54666=CARTESIAN_POINT('Ctrl Pts',(-0.11506242376767,5.16612183484124,80.6021340836397));
#54667=CARTESIAN_POINT('Ctrl Pts',(-3.76287956508864,3.07252682993506,80.7372062738101));
#54668=CARTESIAN_POINT('Ctrl Pts',(-4.36312216851904,0.804706986612936,
80.8193582098985));
#54669=CARTESIAN_POINT('Ctrl Pts',(-4.3651608225263,-0.00123442373144732,
80.8485898919049));
#54670=CARTESIAN_POINT('Origin',(0.,0.,24.1514101080949));
#54671=CARTESIAN_POINT('',(-4.36706479197461,-0.00298086264687759,78.6514101080949));
#54672=CARTESIAN_POINT('',(-4.37877376767475,-0.00119946029119966,78.8485898919049));
#54673=CARTESIAN_POINT('',(-4.372,3.82579154166093E-12,24.1514101080949));
#54674=CARTESIAN_POINT('Ctrl Pts',(-4.36706479197461,-0.00298086264687698,
78.6514101080949));
#54675=CARTESIAN_POINT('Ctrl Pts',(-4.37035845585727,-0.527750657057906,
78.670464427275));
#54676=CARTESIAN_POINT('Ctrl Pts',(-4.03993636744864,-2.50597397148776,
78.7424390005372));
#54677=CARTESIAN_POINT('Ctrl Pts',(-1.0979463908737,-5.04941255383462,78.8673338278812));
#54678=CARTESIAN_POINT('Ctrl Pts',(3.64665478912629,-3.66114220769932,79.0260945901272));
#54679=CARTESIAN_POINT('Ctrl Pts',(5.05372611759689,1.07791731796727,79.184855352373));
#54680=CARTESIAN_POINT('Ctrl Pts',(1.83547293516864,4.83043398881696,79.3436161146189));
#54681=CARTESIAN_POINT('Ctrl Pts',(-2.96262225304742,4.17564214514766,79.4991343665262));
#54682=CARTESIAN_POINT('Ctrl Pts',(-4.37205612685341,1.35742450024673,79.6017323643515));
#54683=CARTESIAN_POINT('Ctrl Pts',(-4.37845870912757,-0.00160159003492056,
79.6514101080949));
#54684=CARTESIAN_POINT('Ctrl Pts',(-4.37877376767475,-0.00119946029119964,
78.8485898919049));
#54685=CARTESIAN_POINT('Ctrl Pts',(-4.37901256877795,-0.0666227183370213,
78.8509818275816));
#54686=CARTESIAN_POINT('Ctrl Pts',(-4.34804095188971,-1.57926832145057,
78.9062940173403));
#54687=CARTESIAN_POINT('Ctrl Pts',(-2.60420306585193,-4.46320294918618,
79.0145264611808));
#54688=CARTESIAN_POINT('Ctrl Pts',(2.33719176176521,-4.60864284172174,79.1732872234268));
#54689=CARTESIAN_POINT('Ctrl Pts',(5.13951729856278,-0.536112032685121,
79.3320479856725));
#54690=CARTESIAN_POINT('Ctrl Pts',(3.23799961511593,4.02708488442023,79.4908087479186));
#54691=CARTESIAN_POINT('Ctrl Pts',(-1.62703422207133,4.90457070639472,79.6495695101643));
#54692=CARTESIAN_POINT('Ctrl Pts',(-4.16301218854004,2.19175778571074,79.7688298914932));
#54693=CARTESIAN_POINT('Ctrl Pts',(-4.37441880163748,0.372715810744746,
79.83517001874));
#54694=CARTESIAN_POINT('Ctrl Pts',(-4.37110144318797,0.00398541688994905,
79.8485898919049));
#54695=CARTESIAN_POINT('Origin',(0.,0.,24.1514101080949));
#54696=CARTESIAN_POINT('',(-4.36767022761989,0.00326609935392151,77.6514101080949));
#54697=CARTESIAN_POINT('',(-4.36757594524889,-0.00322601897944697,77.8485898919049));
#54698=CARTESIAN_POINT('',(-4.372,3.82579154166093E-12,24.1514101080949));
#54699=CARTESIAN_POINT('Ctrl Pts',(-4.36767022761989,0.00326609935392137,
77.6514101080949));
#54700=CARTESIAN_POINT('Ctrl Pts',(-4.36100748821687,-0.956637771051708,
77.6862762361166));
#54701=CARTESIAN_POINT('Ctrl Pts',(-3.57653367776381,-3.38339660944801,
77.7740626182202));
#54702=CARTESIAN_POINT('Ctrl Pts',(0.433232280173729,-5.14920995954434,
77.9147692544059));
#54703=CARTESIAN_POINT('Ctrl Pts',(4.56098553273524,-2.42888130344712,78.0735300166518));
#54704=CARTESIAN_POINT('Ctrl Pts',(4.51438550862023,2.51443371271033,78.2322907788977));
#54705=CARTESIAN_POINT('Ctrl Pts',(0.336081973315249,5.15646219061744,78.3910515411436));
#54706=CARTESIAN_POINT('Ctrl Pts',(-3.61142097688492,3.32845736892325,78.5307579842093));
#54707=CARTESIAN_POINT('Ctrl Pts',(-4.36121084329327,0.929711590329863,
78.6175441731931));
#54708=CARTESIAN_POINT('Ctrl Pts',(-4.36706479197461,-0.00298086264687698,
78.6514101080949));
#54709=CARTESIAN_POINT('Ctrl Pts',(-4.36757594524889,-0.00322601897944683,
77.8485898919049));
#54710=CARTESIAN_POINT('Ctrl Pts',(-4.37100704730013,-0.504422908173594,
77.8667936364231));
#54711=CARTESIAN_POINT('Ctrl Pts',(-4.05983800326864,-2.45852322858237,
77.9379176350233));
#54712=CARTESIAN_POINT('Ctrl Pts',(-1.17875882811733,-5.03116107861318,
78.0619618877055));
#54713=CARTESIAN_POINT('Ctrl Pts',(3.58748974126774,-3.71913585798031,78.2207226499514));
#54714=CARTESIAN_POINT('Ctrl Pts',(5.07035811814355,0.996756102360001,78.3794834121972));
#54715=CARTESIAN_POINT('Ctrl Pts',(1.91267986918918,4.80038643150889,78.5382441744432));
#54716=CARTESIAN_POINT('Ctrl Pts',(-2.92159273453857,4.2194430180671,78.6946130010123));
#54717=CARTESIAN_POINT('Ctrl Pts',(-4.37372922642899,1.38083068620526,78.7980615734996));
#54718=CARTESIAN_POINT('Ctrl Pts',(-4.37877376767475,-0.00119946029119964,
78.8485898919049));
#54719=CARTESIAN_POINT('Origin',(0.,0.,24.1514101080949));
#54720=CARTESIAN_POINT('',(-4.37882057798781,0.00112692768741051,76.6514101080949));
#54721=CARTESIAN_POINT('',(-4.36715155140556,0.00302605917446269,76.8485898919049));
#54722=CARTESIAN_POINT('',(-4.372,3.82579154166093E-12,24.1514101080949));
#54723=CARTESIAN_POINT('Ctrl Pts',(-4.37882057798781,0.00112692768741048,
76.6514101080949));
#54724=CARTESIAN_POINT('Ctrl Pts',(-4.37403747425012,-1.38495585300809,
76.7020880449581));
#54725=CARTESIAN_POINT('Ctrl Pts',(-2.91430837048911,-4.22712294708155,
76.8056862359034));
#54726=CARTESIAN_POINT('Ctrl Pts',(1.92621046639379,-4.79497306094723,76.9622046809306));
#54727=CARTESIAN_POINT('Ctrl Pts',(5.07314897115,-0.982452509068445,77.1209654431764));
#54728=CARTESIAN_POINT('Ctrl Pts',(3.5769865761566,3.7292385885125,77.2797262054224));
#54729=CARTESIAN_POINT('Ctrl Pts',(-1.19294319381297,5.02781661881079,77.4384869676682));
#54730=CARTESIAN_POINT('Ctrl Pts',(-4.06328911396928,2.45017653498889,77.5623816018925));
#54731=CARTESIAN_POINT('Ctrl Pts',(-4.37112027911439,0.500316573992826,
77.6333559820347));
#54732=CARTESIAN_POINT('Ctrl Pts',(-4.36767022761989,0.00326609935392137,
77.6514101080949));
#54733=CARTESIAN_POINT('Ctrl Pts',(-4.36715155140556,0.00302605917446276,
76.8485898919049));
#54734=CARTESIAN_POINT('Ctrl Pts',(-4.36117507900865,-0.933740289083742,
76.8826054452647));
#54735=CARTESIAN_POINT('Ctrl Pts',(-3.60625270295825,-3.33668347601213,
76.9695412527065));
#54736=CARTESIAN_POINT('Ctrl Pts',(0.350623091062388,-5.15549392607834,
77.1093973142301));
#54737=CARTESIAN_POINT('Ctrl Pts',(4.52145892049186,-2.50169210817825,77.268158076476));
#54738=CARTESIAN_POINT('Ctrl Pts',(4.55411743612604,2.44173474230699,77.4269188387219));
#54739=CARTESIAN_POINT('Ctrl Pts',(0.4187085668894,5.15041137287398,77.5856796009678));
#54740=CARTESIAN_POINT('Ctrl Pts',(-3.58180307113106,3.37518619718569,77.7262366186955));
#54741=CARTESIAN_POINT('Ctrl Pts',(-4.36103246255736,0.952610654051967,
77.8138733823412));
#54742=CARTESIAN_POINT('Ctrl Pts',(-4.36757594524889,-0.00322601897944683,
77.8485898919049));
#54743=CARTESIAN_POINT('Origin',(0.,0.,24.1514101080949));
#54744=CARTESIAN_POINT('',(-4.37097940507052,-0.00397941814148454,75.6514101080949));
#54745=CARTESIAN_POINT('',(-4.37851995085447,0.0015322273023494,75.8485898919049));
#54746=CARTESIAN_POINT('',(-4.372,3.82579154166093E-12,24.1514101080949));
#54747=CARTESIAN_POINT('Ctrl Pts',(-4.37097940507052,-0.00397941814148494,
75.6514101080949));
#54748=CARTESIAN_POINT('Ctrl Pts',(-4.3743208173595,-0.376847295339705,
75.6649795997177));
#54749=CARTESIAN_POINT('Ctrl Pts',(-4.16000539985281,-2.20009534110889,
75.7314693454226));
#54750=CARTESIAN_POINT('Ctrl Pts',(-1.61319567320764,-4.90913975519121,
75.8508793452094));
#54751=CARTESIAN_POINT('Ctrl Pts',(3.24934402869518,-4.01793688343129,76.0096401074552));
#54752=CARTESIAN_POINT('Ctrl Pts',(5.13798482303055,0.550604553524979,76.1684008697012));
#54753=CARTESIAN_POINT('Ctrl Pts',(2.32418496553848,4.61521588466023,76.3271616319469));
#54754=CARTESIAN_POINT('Ctrl Pts',(-2.61677996556865,4.45584066454958,76.485922394193));
#54755=CARTESIAN_POINT('Ctrl Pts',(-4.35007811558771,1.57099298812344,76.5940052195755));
#54756=CARTESIAN_POINT('Ctrl Pts',(-4.37903221319898,0.0624561269022633,
76.6491677908762));
#54757=CARTESIAN_POINT('Ctrl Pts',(-4.37882057798781,0.00112692768741048,
76.6514101080949));
#54758=CARTESIAN_POINT('Ctrl Pts',(-4.37851995085447,0.00153222730234961,
75.8485898919049));
#54759=CARTESIAN_POINT('Ctrl Pts',(-4.37234073616906,-1.36153629732671,
75.8984172541062));
#54760=CARTESIAN_POINT('Ctrl Pts',(-2.9554520406374,-4.18336396709743,76.0011648703895));
#54761=CARTESIAN_POINT('Ctrl Pts',(1.84908863423975,-4.82523837717284,76.1568327407549));
#54762=CARTESIAN_POINT('Ctrl Pts',(5.05674607440601,-1.06366033713594,76.3155935030006));
#54763=CARTESIAN_POINT('Ctrl Pts',(3.63631504695578,3.6714121333759,76.4743542652466));
#54764=CARTESIAN_POINT('Ctrl Pts',(-1.11218258415778,5.04629607467818,76.6331150274925));
#54765=CARTESIAN_POINT('Ctrl Pts',(-4.04347203458464,2.49762731386996,76.7578602363785));
#54766=CARTESIAN_POINT('Ctrl Pts',(-4.37047307379395,0.523649295054832,
76.8296851911827));
#54767=CARTESIAN_POINT('Ctrl Pts',(-4.36715155140556,0.00302605917446276,
76.8485898919049));
#54768=CARTESIAN_POINT('Origin',(0.,0.,24.1514101080949));
#54769=CARTESIAN_POINT('',(-4.36519646031047,0.00129875109319553,74.6514101080949));
#54770=CARTESIAN_POINT('',(-4.37167806635839,-0.00399716320838295,74.8485898919049));
#54771=CARTESIAN_POINT('',(-4.372,3.82579154166093E-12,24.1514101080949));
#54772=CARTESIAN_POINT('Ctrl Pts',(-4.36519646031047,0.00129875109319548,
74.6514101080949));
#54773=CARTESIAN_POINT('Ctrl Pts',(-4.36303959174397,-0.808751209913892,
74.6807914085593));
#54774=CARTESIAN_POINT('Ctrl Pts',(-3.75824647517972,-3.08081912741743,
74.7630929631056));
#54775=CARTESIAN_POINT('Ctrl Pts',(-0.100492272925181,-5.16642571988962,
74.898314771734));
#54776=CARTESIAN_POINT('Ctrl Pts',(4.28596496729055,-2.88661700182285,75.0570755339799));
#54777=CARTESIAN_POINT('Ctrl Pts',(4.74977615293751,2.03511176917654,75.2158362962258));
#54778=CARTESIAN_POINT('Ctrl Pts',(0.866447119614458,5.09424408572719,75.3745970584717));
#54779=CARTESIAN_POINT('Ctrl Pts',(-3.41018887347201,3.62800267766814,75.5197883290947));
#54780=CARTESIAN_POINT('Ctrl Pts',(-4.36128949737787,1.07731645292395,75.6120593456358));
#54781=CARTESIAN_POINT('Ctrl Pts',(-4.37097940507052,-0.00397941814148494,
75.6514101080949));
#54782=CARTESIAN_POINT('Ctrl Pts',(-4.37167806635839,-0.00399716320838302,
74.8485898919049));
#54783=CARTESIAN_POINT('Ctrl Pts',(-4.37486787390589,-0.3533501983587,74.8613088088659));
#54784=CARTESIAN_POINT('Ctrl Pts',(-4.1769137234544,-2.15270356402942,74.9269479799088));
#54785=CARTESIAN_POINT('Ctrl Pts',(-1.69169300421356,-4.88264569196979,
75.0455074050335));
#54786=CARTESIAN_POINT('Ctrl Pts',(3.18450981172911,-4.06951488912588,75.2042681672795));
#54787=CARTESIAN_POINT('Ctrl Pts',(5.14615197585861,0.468160245196775,75.3630289295254));
#54788=CARTESIAN_POINT('Ctrl Pts',(2.39787866042351,4.57736082297456,75.5217896917712));
#54789=CARTESIAN_POINT('Ctrl Pts',(-2.54500644918866,4.49722095825909,75.6805504540172));
#54790=CARTESIAN_POINT('Ctrl Pts',(-4.33833518668749,1.61805156266242,75.7894838540617));
#54791=CARTESIAN_POINT('Ctrl Pts',(-4.37890350804243,0.0861408316175627,
75.8454970000243));
#54792=CARTESIAN_POINT('Ctrl Pts',(-4.37851995085447,0.00153222730234961,
75.8485898919049));
#54793=CARTESIAN_POINT('Origin',(0.,0.,24.1514101080949));
#54794=CARTESIAN_POINT('',(-4.37573799308197,0.00329254665532695,73.6514101080949));
#54795=CARTESIAN_POINT('',(-4.36501807785945,0.000928765700389245,73.8485898919049));
#54796=CARTESIAN_POINT('',(-4.372,3.82579154166093E-12,24.1514101080949));
#54797=CARTESIAN_POINT('Ctrl Pts',(-4.37573799308197,0.00329254665532727,
73.6514101080949));
#54798=CARTESIAN_POINT('Ctrl Pts',(-4.36535453025917,-1.23506946531353,
73.6966032174009));
#54799=CARTESIAN_POINT('Ctrl Pts',(-3.16833117156948,-3.94108625070045,
73.7947165807888));
#54800=CARTESIAN_POINT('Ctrl Pts',(1.42107208653042,-4.9681593715318,73.9457501982587));
#54801=CARTESIAN_POINT('Ctrl Pts',(4.94466868411869,-1.50076814343543,74.1045109605046));
#54802=CARTESIAN_POINT('Ctrl Pts',(3.94275346512999,3.34017193109278,74.2632717227505));
#54803=CARTESIAN_POINT('Ctrl Pts',(-0.667690158118302,5.12408462740484,
74.4220324849963));
#54804=CARTESIAN_POINT('Ctrl Pts',(-3.9268970087966,2.75604594892831,74.5514119467779));
#54805=CARTESIAN_POINT('Ctrl Pts',(-4.3669244447204,0.650273716756605,74.6278711544774));
#54806=CARTESIAN_POINT('Ctrl Pts',(-4.36519646031047,0.00129875109319548,
74.6514101080949));
#54807=CARTESIAN_POINT('Ctrl Pts',(-4.36501807785945,0.000928765700389245,
73.8485898919049));
#54808=CARTESIAN_POINT('Ctrl Pts',(-4.36352375843653,-0.785750920308218,
73.8771206177074));
#54809=CARTESIAN_POINT('Ctrl Pts',(-3.78436122884701,-3.0336560998423,73.9585715975918));
#54810=CARTESIAN_POINT('Ctrl Pts',(-0.183308880309829,-5.16415065893858,
74.0929428315583));
#54811=CARTESIAN_POINT('Ctrl Pts',(4.23913515679244,-2.95495977912772,74.2517035938041));
#54812=CARTESIAN_POINT('Ctrl Pts',(4.78179321232898,1.95870055096247,74.4104643560501));
#54813=CARTESIAN_POINT('Ctrl Pts',(0.948008058166557,5.07969830752458,74.5692251182959));
#54814=CARTESIAN_POINT('Ctrl Pts',(-3.37677384390662,3.67402258696438,74.7152669635808));
#54815=CARTESIAN_POINT('Ctrl Pts',(-4.36159587705234,1.10022100123729,74.8083885547839));
#54816=CARTESIAN_POINT('Ctrl Pts',(-4.37167806635839,-0.00399716320838302,
74.8485898919049));
#54817=CARTESIAN_POINT('Origin',(0.,0.,24.1514101080949));
#54818=CARTESIAN_POINT('',(-4.37546659946853,-0.00338795269852561,72.6514101080949));
#54819=CARTESIAN_POINT('',(-4.37508401727703,0.00350862331529297,72.848589891905));
#54820=CARTESIAN_POINT('',(-4.372,3.82579154166093E-12,24.1514101080949));
#54821=CARTESIAN_POINT('Ctrl Pts',(-4.37546659946853,-0.00338795269852542,
72.6514101080949));
#54822=CARTESIAN_POINT('Ctrl Pts',(-4.37736040129649,-0.224956166423907,
72.6594947721605));
#54823=CARTESIAN_POINT('Ctrl Pts',(-4.26133239251396,-1.89486696261105,
72.720499690308));
#54824=CARTESIAN_POINT('Ctrl Pts',(-2.1112172128698,-4.71644095649861,72.8344248625374));
#54825=CARTESIAN_POINT('Ctrl Pts',(2.81733266516402,-4.33182294996633,72.9931856247833));
#54826=CARTESIAN_POINT('Ctrl Pts',(5.16737363149282,0.0174117376300544,
73.1519463870293));
#54827=CARTESIAN_POINT('Ctrl Pts',(2.78807641079671,4.35071067109887,73.3107071492751));
#54828=CARTESIAN_POINT('Ctrl Pts',(-2.14295350396336,4.70210630419026,73.469467911521));
#54829=CARTESIAN_POINT('Ctrl Pts',(-4.26731753777204,1.87500660994908,73.5830355644609));
#54830=CARTESIAN_POINT('Ctrl Pts',(-4.37751336374666,0.215028421847947,
73.6436829633189));
#54831=CARTESIAN_POINT('Ctrl Pts',(-4.37573799308197,0.00329254665532727,
73.6514101080949));
#54832=CARTESIAN_POINT('Ctrl Pts',(-4.37508401727703,0.00350862331529318,
72.848589891905));
#54833=CARTESIAN_POINT('Ctrl Pts',(-4.36445811409486,-1.21201843518349,
72.892932426549));
#54834=CARTESIAN_POINT('Ctrl Pts',(-3.20535851125622,-3.89598203052578,
72.9901952152748));
#54835=CARTESIAN_POINT('Ctrl Pts',(1.34123860080759,-4.99030391755056,73.140378258083));
#54836=CARTESIAN_POINT('Ctrl Pts',(4.91997252333115,-1.57984953191204,73.2991390203287));
#54837=CARTESIAN_POINT('Ctrl Pts',(3.99579730998455,3.27653140246455,73.4578997825747));
#54838=CARTESIAN_POINT('Ctrl Pts',(-0.585453654677876,5.13413071435083,
73.6166605448206));
#54839=CARTESIAN_POINT('Ctrl Pts',(-3.90388041542688,2.80342624447369,73.746890581264));
#54840=CARTESIAN_POINT('Ctrl Pts',(-4.36629549877317,0.673422924511184,
73.8242003636254));
#54841=CARTESIAN_POINT('Ctrl Pts',(-4.36501807785945,0.000928765700389245,
73.8485898919049));
#54842=CARTESIAN_POINT('Origin',(0.,0.,24.1514101080949));
#54843=CARTESIAN_POINT('',(-4.3651141969528,-0.00114447055126671,71.6514101080949));
#54844=CARTESIAN_POINT('',(-4.37610278806197,-0.00315032678594118,71.8485898919049));
#54845=CARTESIAN_POINT('',(-4.372,3.82579154166093E-12,24.1514101080949));
#54846=CARTESIAN_POINT('Ctrl Pts',(-4.3651141969528,-0.00114447055126629,
71.6514101080949));
#54847=CARTESIAN_POINT('Ctrl Pts',(-4.36665839117516,-0.660007333527467,
71.675306581002));
#54848=CARTESIAN_POINT('Ctrl Pts',(-3.91728495207162,-2.77596398718315,
71.7521233079911));
#54849=CARTESIAN_POINT('Ctrl Pts',(-0.63314364249968,-5.12846785541421,
71.8818602890621));
#54850=CARTESIAN_POINT('Ctrl Pts',(3.9651734499498,-3.31352575482195,72.040621051308));
#54851=CARTESIAN_POINT('Ctrl Pts',(4.93444268320512,1.53405632954553,72.1993818135539));
#54852=CARTESIAN_POINT('Ctrl Pts',(1.38755924827672,4.97762320275213,72.3581425757998));
#54853=CARTESIAN_POINT('Ctrl Pts',(-3.18397114357576,3.92214967618973,72.50881867398));
#54854=CARTESIAN_POINT('Ctrl Pts',(-4.36496403292504,1.22537573008428,72.6065745180785));
#54855=CARTESIAN_POINT('Ctrl Pts',(-4.37546659946853,-0.00338795269852542,
72.6514101080949));
#54856=CARTESIAN_POINT('Ctrl Pts',(-4.37610278806197,-0.00315032678594042,
71.8485898919049));
#54857=CARTESIAN_POINT('Ctrl Pts',(-4.37771416984263,-0.201332656341541,
71.8558239813086));
#54858=CARTESIAN_POINT('Ctrl Pts',(-4.27545064435103,-1.84762538881353,
71.9159783247941));
#54859=CARTESIAN_POINT('Ctrl Pts',(-2.18656114390733,-4.68198724237597,
72.0290529223616));
#54860=CARTESIAN_POINT('Ctrl Pts',(2.74752166081747,-4.3764344959288,72.1878136846077));
#54861=CARTESIAN_POINT('Ctrl Pts',(5.16698871742013,-0.0654352188752399,
72.3465744468534));
#54862=CARTESIAN_POINT('Ctrl Pts',(2.85746987211454,4.30545236923763,72.5053352090995));
#54863=CARTESIAN_POINT('Ctrl Pts',(-2.06729268270395,4.73585843726931,72.6640959713451));
#54864=CARTESIAN_POINT('Ctrl Pts',(-4.2529565583671,1.92226442851864,72.7785141989471));
#54865=CARTESIAN_POINT('Ctrl Pts',(-4.37713951584072,0.238642906024094,
72.840012172467));
#54866=CARTESIAN_POINT('Ctrl Pts',(-4.37508401727703,0.00350862331529318,
72.848589891905));
#54867=CARTESIAN_POINT('Origin',(0.,0.,24.1514101080949));
#54868=CARTESIAN_POINT('',(-4.37127157619262,0.00399172071570709,70.6514101080949));
#54869=CARTESIAN_POINT('',(-4.36532703354517,-0.00150807403881736,70.8485898919049));
#54870=CARTESIAN_POINT('',(-4.372,3.82579154166093E-12,24.1514101080949));
#54871=CARTESIAN_POINT('Ctrl Pts',(-4.37127157619262,0.00399172071570714,
70.6514101080949));
#54872=CARTESIAN_POINT('Ctrl Pts',(-4.36140746653353,-1.08694237129441,
70.6911183898435));
#54873=CARTESIAN_POINT('Ctrl Pts',(-3.39621711134158,-3.64736222930015,
70.7837469256742));
#54874=CARTESIAN_POINT('Ctrl Pts',(0.900757702520816,-5.08828939599587,
70.9292957155868));
#54875=CARTESIAN_POINT('Ctrl Pts',(4.76338297422217,-2.00305667841551,71.0880564778326));
#54876=CARTESIAN_POINT('Ctrl Pts',(4.26641464848803,2.9154346954137,71.2468172400786));
#54877=CARTESIAN_POINT('Ctrl Pts',(-0.135306682874774,5.16563118288797,
71.4055780023244));
#54878=CARTESIAN_POINT('Ctrl Pts',(-3.76928933575608,3.06100151884775,71.5404422916632));
#54879=CARTESIAN_POINT('Ctrl Pts',(-4.36323867518121,0.799086242725653,
71.62238632692));
#54880=CARTESIAN_POINT('Ctrl Pts',(-4.3651141969528,-0.00114447055126629,
71.6514101080949));
#54881=CARTESIAN_POINT('Ctrl Pts',(-4.36532703354517,-0.00150807403881757,
70.8485898919049));
#54882=CARTESIAN_POINT('Ctrl Pts',(-4.36729483924552,-0.636841944886774,
70.8716357901501));
#54883=CARTESIAN_POINT('Ctrl Pts',(-3.94000526365074,-2.72857085726927,
70.9476019424773));
#54884=CARTESIAN_POINT('Ctrl Pts',(-0.715283247733823,-5.11765806295492,
71.0764883488864));
#54885=CARTESIAN_POINT('Ctrl Pts',(3.91154054911197,-3.37667065413102,71.2352491111322));
#54886=CARTESIAN_POINT('Ctrl Pts',(4.95840295584866,1.45474887910182,71.3940098733782));
#54887=CARTESIAN_POINT('Ctrl Pts',(1.46718352100222,4.95473780229749,71.552770635624));
#54888=CARTESIAN_POINT('Ctrl Pts',(-3.14657975547223,3.96714821422749,71.7042973084663));
#54889=CARTESIAN_POINT('Ctrl Pts',(-4.36592626835323,1.24845026027391,71.8029037272266));
#54890=CARTESIAN_POINT('Ctrl Pts',(-4.37610278806197,-0.00315032678594042,
71.8485898919049));
#54891=CARTESIAN_POINT('Origin',(0.,0.,24.1514101080949));
#54892=CARTESIAN_POINT('',(-4.37870422100453,-0.0012994166445059,69.6514101080949));
#54893=CARTESIAN_POINT('',(-4.3705809381838,0.00395105542623939,69.848589891905));
#54894=CARTESIAN_POINT('',(-4.372,3.82579154166093E-12,24.1514101080949));
#54895=CARTESIAN_POINT('Ctrl Pts',(-4.37870422100453,-0.00129941664450634,
69.6514101080949));
#54896=CARTESIAN_POINT('Ctrl Pts',(-4.3789830325923,-0.0724121058889038,
69.6540099446031));
#54897=CARTESIAN_POINT('Ctrl Pts',(-4.34518999704772,-1.59076889411841,
69.7095300351934));
#54898=CARTESIAN_POINT('Ctrl Pts',(-2.58669250630018,-4.47337403912361,
69.8179703798655));
#54899=CARTESIAN_POINT('Ctrl Pts',(2.35523426198658,-4.5994483350962,69.9767311421114));
#54900=CARTESIAN_POINT('Ctrl Pts',(5.14157869213602,-0.51596702281012,70.1354919043573));
#54901=CARTESIAN_POINT('Ctrl Pts',(3.22219325167658,4.03974306916968,70.2942526666032));
#54902=CARTESIAN_POINT('Ctrl Pts',(-1.6462418758917,4.89815690868675,70.4530134288491));
#54903=CARTESIAN_POINT('Ctrl Pts',(-4.16716700492617,2.18017319825989,70.5720659093463));
#54904=CARTESIAN_POINT('Ctrl Pts',(-4.3745536205967,0.366973708511667,70.6381981357616));
#54905=CARTESIAN_POINT('Ctrl Pts',(-4.37127157619262,0.00399172071570714,
70.6514101080949));
#54906=CARTESIAN_POINT('Ctrl Pts',(-4.3705809381838,0.00395105542623928,
69.848589891905));
#54907=CARTESIAN_POINT('Ctrl Pts',(-4.36115189233779,-1.06404425239527,
69.8874475989916));
#54908=CARTESIAN_POINT('Ctrl Pts',(-3.42928322572819,-3.60126660220352,
69.9792255601602));
#54909=CARTESIAN_POINT('Ctrl Pts',(0.819065126108891,-5.102076684352,70.1239237754111));
#54910=CARTESIAN_POINT('Ctrl Pts',(4.73065728621489,-2.07916709626671,70.2826845376568));
#54911=CARTESIAN_POINT('Ctrl Pts',(4.31260739816882,2.84665972730784,70.4414452999028));
#54912=CARTESIAN_POINT('Ctrl Pts',(-0.0524725109896868,5.16713661609669,
70.6002060621488));
#54913=CARTESIAN_POINT('Ctrl Pts',(-3.74285914641375,3.1081338808624,70.7359209261493));
#54914=CARTESIAN_POINT('Ctrl Pts',(-4.36277617060702,0.822074063266301,
70.8187155360681));
#54915=CARTESIAN_POINT('Ctrl Pts',(-4.36532703354517,-0.00150807403881757,
70.8485898919049));
#54916=CARTESIAN_POINT('Origin',(0.,0.,24.1514101080949));
#54917=CARTESIAN_POINT('',(-4.36744694438276,-0.00316878230680772,68.6514101080949));
#54918=CARTESIAN_POINT('',(-4.37895590169143,-0.000884728325120654,68.848589891905));
#54919=CARTESIAN_POINT('',(-4.372,3.82579154166093E-12,24.1514101080949));
#54920=CARTESIAN_POINT('Ctrl Pts',(-4.36744694438276,-0.0031687823068071,
68.6514101080949));
#54921=CARTESIAN_POINT('Ctrl Pts',(-4.37084913112638,-0.510127366468858,
68.6698217534447));
#54922=CARTESIAN_POINT('Ctrl Pts',(-4.05501785193817,-2.47012128343436,
68.7411536528764));
#54923=CARTESIAN_POINT('Ctrl Pts',(-1.15903350388962,-5.03574172817834,
68.8654058063903));
#54924=CARTESIAN_POINT('Ctrl Pts',(3.60203679805415,-3.70504849111566,69.0241665686361));
#54925=CARTESIAN_POINT('Ctrl Pts',(5.06641299677213,1.01661829719571,69.182927330882));
#54926=CARTESIAN_POINT('Ctrl Pts',(1.89385326524434,4.80784496690336,69.3416880931279));
#54927=CARTESIAN_POINT('Ctrl Pts',(-2.93168118063718,4.20875891624129,69.4978490188655));
#54928=CARTESIAN_POINT('Ctrl Pts',(-4.37330776031301,1.37510260179151,69.6010896905212));
#54929=CARTESIAN_POINT('Ctrl Pts',(-4.37870422100453,-0.00129941664450634,
69.6514101080949));
#54930=CARTESIAN_POINT('Ctrl Pts',(-4.37895590169143,-0.00088472832512114,
68.848589891905));
#54931=CARTESIAN_POINT('Ctrl Pts',(-4.37908827342486,-0.0487245072402155,
68.8503391537513));
#54932=CARTESIAN_POINT('Ctrl Pts',(-4.35670634828455,-1.54372976222875,
68.9050086696796));
#54933=CARTESIAN_POINT('Ctrl Pts',(-2.65807841962993,-4.43132861441282,
69.0125984396897));
#54934=CARTESIAN_POINT('Ctrl Pts',(2.2811920004135,-4.63661700284439,69.1713592019357));
#54935=CARTESIAN_POINT('Ctrl Pts',(5.1326458217616,-0.598331882962418,69.3301199641815));
#54936=CARTESIAN_POINT('Ctrl Pts',(3.28654540832559,3.98756485249208,69.4888807264275));
#54937=CARTESIAN_POINT('Ctrl Pts',(-1.56750175164667,4.92392043319156,69.6476414886732));
#54938=CARTESIAN_POINT('Ctrl Pts',(-4.14999820818835,2.2275746797718,69.7675445438326));
#54939=CARTESIAN_POINT('Ctrl Pts',(-4.37399329599569,0.390456985212737,
69.8345273449097));
#54940=CARTESIAN_POINT('Ctrl Pts',(-4.3705809381838,0.00395105542623928,
69.848589891905));
#54941=CARTESIAN_POINT('Origin',(0.,0.,24.1514101080949));
#54942=CARTESIAN_POINT('',(-4.36727426748866,0.00308741741996557,67.6514101080949));
#54943=CARTESIAN_POINT('',(-4.36799009248299,-0.00339142969553563,67.8485898919049));
#54944=CARTESIAN_POINT('',(-4.372,3.82579154166093E-12,24.1514101080949));
#54945=CARTESIAN_POINT('Ctrl Pts',(-4.36727426748866,0.0030874174199657,
67.6514101080949));
#54946=CARTESIAN_POINT('Ctrl Pts',(-4.36112833884136,-0.939337788388386,
67.6856335622863));
#54947=CARTESIAN_POINT('Ctrl Pts',(-3.59904165290846,-3.34810943987296,
67.7727772705596));
#54948=CARTESIAN_POINT('Ctrl Pts',(0.370823889097725,-5.15408023407956,
67.9128412329148));
#54949=CARTESIAN_POINT('Ctrl Pts',(4.53122783943781,-2.48395404207855,68.0716019951608));
#54950=CARTESIAN_POINT('Ctrl Pts',(4.5445136629679,2.45956276259679,68.2303627574067));
#54951=CARTESIAN_POINT('Ctrl Pts',(0.398521768172548,5.15201259862078,68.3891235196525));
#54952=CARTESIAN_POINT('Ctrl Pts',(-3.58909538685354,3.36377270257325,68.5294726365487));
#54953=CARTESIAN_POINT('Ctrl Pts',(-4.36107028825353,0.947014381222592,
68.6169014993627));
#54954=CARTESIAN_POINT('Ctrl Pts',(-4.36744694438276,-0.0031687823068071,
68.6514101080949));
#54955=CARTESIAN_POINT('Ctrl Pts',(-4.36799009248299,-0.00339142969553514,
67.8485898919049));
#54956=CARTESIAN_POINT('Ctrl Pts',(-4.37149165529305,-0.486778408785156,
67.8661509625928));
#54957=CARTESIAN_POINT('Ctrl Pts',(-4.07455789488293,-2.42267137940883,
67.9366322873626));
#54958=CARTESIAN_POINT('Ctrl Pts',(-1.23961891643423,-5.01651264483955,
68.0600338662145));
#54959=CARTESIAN_POINT('Ctrl Pts',(3.54217356679019,-3.76232117137135,68.2187946284603));
#54960=CARTESIAN_POINT('Ctrl Pts',(5.08206060458778,0.935261559732356,68.3775553907062));
#54961=CARTESIAN_POINT('Ctrl Pts',(1.97069054350433,4.77686434343271,68.5363161529522));
#54962=CARTESIAN_POINT('Ctrl Pts',(-2.89016105242335,4.25237825733215,68.6933276533517));
#54963=CARTESIAN_POINT('Ctrl Pts',(-4.37508364382578,1.39856782394589,68.7974188996693));
#54964=CARTESIAN_POINT('Ctrl Pts',(-4.37895590169143,-0.00088472832512114,
68.848589891905));
#54965=CARTESIAN_POINT('Origin',(0.,0.,24.1514101080949));
#54966=CARTESIAN_POINT('',(-4.37860089698225,0.00143482616460942,66.6514101080949));
#54967=CARTESIAN_POINT('',(-4.36678925203502,0.00282595512297229,66.8485898919049));
#54968=CARTESIAN_POINT('',(-4.372,3.82579154166093E-12,24.1514101080949));
#54969=CARTESIAN_POINT('Ctrl Pts',(-4.37860089698225,0.00143482616460969,
66.6514101080949));
#54970=CARTESIAN_POINT('Ctrl Pts',(-4.37274293747686,-1.3672535432393,66.7014453711278));
#54971=CARTESIAN_POINT('Ctrl Pts',(-2.94545539126712,-4.19408159696058,
66.8044008882426));
#54972=CARTESIAN_POINT('Ctrl Pts',(1.86798369006022,-4.81795499664787,66.9602766594396));
#54973=CARTESIAN_POINT('Ctrl Pts',(5.06087547593053,-1.04383563513614,67.1190374216854));
#54974=CARTESIAN_POINT('Ctrl Pts',(3.62189943977487,3.68563398402679,67.2777981839313));
#54975=CARTESIAN_POINT('Ctrl Pts',(-1.13194959602156,5.04189880185246,67.4365589461772));
#54976=CARTESIAN_POINT('Ctrl Pts',(-4.04836008668961,2.48602916041319,67.5610962542317));
#54977=CARTESIAN_POINT('Ctrl Pts',(-4.37063188292449,0.517948815873062,
67.6327133082043));
#54978=CARTESIAN_POINT('Ctrl Pts',(-4.36727426748866,0.0030874174199657,
67.6514101080949));
#54979=CARTESIAN_POINT('Ctrl Pts',(-4.36678925203502,0.00282595512297222,
66.8485898919049));
#54980=CARTESIAN_POINT('Ctrl Pts',(-4.36134189412171,-0.916433051844979,
66.8819627714344));
#54981=CARTESIAN_POINT('Ctrl Pts',(-3.62832781641238,-3.30133069322053,
66.9682559050458));
#54982=CARTESIAN_POINT('Ctrl Pts',(0.288144638596748,-5.15936302667923,
67.1074692927391));
#54983=CARTESIAN_POINT('Ctrl Pts',(4.49082211047655,-2.55628068604989,67.266230054985));
#54984=CARTESIAN_POINT('Ctrl Pts',(4.58336201290063,2.38638782106256,67.4249908172308));
#54985=CARTESIAN_POINT('Ctrl Pts',(0.481069000502546,5.14496130117338,67.5837515794768));
#54986=CARTESIAN_POINT('Ctrl Pts',(-3.55904252406398,3.41043311335412,67.7249512710348));
#54987=CARTESIAN_POINT('Ctrl Pts',(-4.36093970223245,0.969907359868089,
67.8132307085108));
#54988=CARTESIAN_POINT('Ctrl Pts',(-4.36799009248299,-0.00339142969553514,
67.8485898919049));
#54989=CARTESIAN_POINT('Origin',(0.,0.,24.1514101080949));
#54990=CARTESIAN_POINT('',(-4.37150619923976,-0.00399650483370713,65.6514101080949));
#54991=CARTESIAN_POINT('',(-4.37824072692977,0.00182550535674644,65.8485898919049));
#54992=CARTESIAN_POINT('',(-4.372,3.82579154166093E-12,24.1514101080949));
#54993=CARTESIAN_POINT('Ctrl Pts',(-4.37150619923976,-0.00399650483370689,
65.6514101080949));
#54994=CARTESIAN_POINT('Ctrl Pts',(-4.37473632420811,-0.359095615586663,
65.6643369258874));
#54995=CARTESIAN_POINT('Ctrl Pts',(-4.17282222069464,-2.16428561428065,
65.7301839977619));
#54996=CARTESIAN_POINT('Ctrl Pts',(-1.67254574036732,-4.88923758498539,
65.8489513237183));
#54997=CARTESIAN_POINT('Ctrl Pts',(3.20043304382085,-4.05700403599433,66.0077120859643));
#54998=CARTESIAN_POINT('Ctrl Pts',(5.14427774780404,0.488323529540513,66.16647284821));
#54999=CARTESIAN_POINT('Ctrl Pts',(2.3799223229872,4.58672248480354,66.3252336104561));
#55000=CARTESIAN_POINT('Ctrl Pts',(-2.56261070750152,4.48721291871176,66.4839943727018));
#55001=CARTESIAN_POINT('Ctrl Pts',(-4.34124164729195,1.60654622778481,66.5927198719149));
#55002=CARTESIAN_POINT('Ctrl Pts',(-4.37893866198466,0.0803522427089276,
66.6485251170459));
#55003=CARTESIAN_POINT('Ctrl Pts',(-4.37860089698225,0.00143482616460969,
66.6514101080949));
#55004=CARTESIAN_POINT('Ctrl Pts',(-4.37824072692977,0.00182550535674642,
65.8485898919049));
#55005=CARTESIAN_POINT('Ctrl Pts',(-4.37114754505431,-1.34389016319695,
65.8977745802759));
#55006=CARTESIAN_POINT('Ctrl Pts',(-2.98610974303986,-4.15014526257514,
65.9998795227288));
#55007=CARTESIAN_POINT('Ctrl Pts',(1.79050088812788,-4.84728385216189,66.1549047192638));
#55008=CARTESIAN_POINT('Ctrl Pts',(5.04349004573647,-1.12483880283976,66.3136654815096));
#55009=CARTESIAN_POINT('Ctrl Pts',(3.68052305807757,3.62709307749002,66.4724262437556));
#55010=CARTESIAN_POINT('Ctrl Pts',(-1.05097105537457,5.05939858230018,66.6311870060014));
#55011=CARTESIAN_POINT('Ctrl Pts',(-4.02817917541877,2.53347937952348,66.7565748887179));
#55012=CARTESIAN_POINT('Ctrl Pts',(-4.36997991304344,0.541260167974116,
66.8290425173524));
#55013=CARTESIAN_POINT('Ctrl Pts',(-4.36678925203502,0.00282595512297222,
66.8485898919049));
#55014=CARTESIAN_POINT('Origin',(0.,0.,24.1514101080949));
#55015=CARTESIAN_POINT('',(-4.36505611781897,0.00102009982110932,64.6514101080949));
#55016=CARTESIAN_POINT('',(-4.37221209240493,-0.00398401159164008,64.848589891905));
#55017=CARTESIAN_POINT('',(-4.372,3.82579154166093E-12,24.1514101080949));
#55018=CARTESIAN_POINT('Ctrl Pts',(-4.36505611781897,0.00102009982110941,
64.6514101080949));
#55019=CARTESIAN_POINT('Ctrl Pts',(-4.36340207653842,-0.791374776421536,
64.680148734729));
#55020=CARTESIAN_POINT('Ctrl Pts',(-3.7780282066601,-3.04518855619851,64.7618076154451));
#55021=CARTESIAN_POINT('Ctrl Pts',(-0.163070050579303,-5.16482928804609,
64.8963867502428));
#55022=CARTESIAN_POINT('Ctrl Pts',(4.25068252576661,-2.93832460446375,65.0551475124889));
#55023=CARTESIAN_POINT('Ctrl Pts',(4.77408061574266,1.97742450941745,65.2139082747347));
#55024=CARTESIAN_POINT('Ctrl Pts',(0.928094299999949,5.08337431106172,65.3726690369806));
#55025=CARTESIAN_POINT('Ctrl Pts',(-3.38499698876322,3.66278651613716,65.518502981434));
#55026=CARTESIAN_POINT('Ctrl Pts',(-4.36151272681657,1.09462141415472,65.6114166718055));
#55027=CARTESIAN_POINT('Ctrl Pts',(-4.37150619923976,-0.00399650483370689,
65.6514101080949));
#55028=CARTESIAN_POINT('Ctrl Pts',(-4.37221209240492,-0.00398401159164036,
64.848589891905));
#55029=CARTESIAN_POINT('Ctrl Pts',(-4.37526481066381,-0.335581023561335,
64.8606661350355));
#55030=CARTESIAN_POINT('Ctrl Pts',(-4.18939334686749,-2.11690750379085,
64.925662632248));
#55031=CARTESIAN_POINT('Ctrl Pts',(-1.75071636731768,-4.86179456322688,
65.0435793835425));
#55032=CARTESIAN_POINT('Ctrl Pts',(3.1349787773885,-4.10779286711735,65.2023401457884));
#55033=CARTESIAN_POINT('Ctrl Pts',(5.15144558585509,0.405786335144852,65.3611009080343));
#55034=CARTESIAN_POINT('Ctrl Pts',(2.45315204119292,4.54797748857745,65.5198616702802));
#55035=CARTESIAN_POINT('Ctrl Pts',(-2.49034118407384,4.52772072468283,65.6786224325261));
#55036=CARTESIAN_POINT('Ctrl Pts',(-4.32920116011288,1.65362984026736,65.788198506401));
#55037=CARTESIAN_POINT('Ctrl Pts',(-4.37877945245337,0.104032299273348,
65.844854326194));
#55038=CARTESIAN_POINT('Ctrl Pts',(-4.37824072692977,0.00182550535674642,
65.8485898919049));
#55039=CARTESIAN_POINT('Origin',(0.,0.,24.1514101080949));
#55040=CARTESIAN_POINT('',(-4.37524640365158,0.00345929889477671,63.6514101080949));
#55041=CARTESIAN_POINT('',(-4.36492309298158,0.000643490633093768,63.848589891905));
#55042=CARTESIAN_POINT('',(-4.372,3.82579154166093E-12,24.1514101080949));
#55043=CARTESIAN_POINT('Ctrl Pts',(-4.37524640365158,0.00345929889477663,
63.6514101080949));
#55044=CARTESIAN_POINT('Ctrl Pts',(-4.36466684100657,-1.21764908937452,
63.6959605435705));
#55045=CARTESIAN_POINT('Ctrl Pts',(-3.19636598506899,-3.90702309781776,
63.7934312331281));
#55046=CARTESIAN_POINT('Ctrl Pts',(1.36078442693529,-4.98500944427043,63.9438221767676));
#55047=CARTESIAN_POINT('Ctrl Pts',(4.92612583383742,-1.56055685101642,64.1025829390136));
#55048=CARTESIAN_POINT('Ctrl Pts',(3.98292640713875,3.29216504011747,64.2613437012594));
#55049=CARTESIAN_POINT('Ctrl Pts',(-0.605568927444514,5.13179692604536,
64.4201044635054));
#55050=CARTESIAN_POINT('Ctrl Pts',(-3.90955357406592,2.79184753823524,64.5501265991171));
#55051=CARTESIAN_POINT('Ctrl Pts',(-4.36644788265656,0.667767259764548,
64.627228480647));
#55052=CARTESIAN_POINT('Ctrl Pts',(-4.36505611781897,0.00102009982110941,
64.6514101080949));
#55053=CARTESIAN_POINT('Ctrl Pts',(-4.36492309298158,0.000643490633093699,
63.8485898919049));
#55054=CARTESIAN_POINT('Ctrl Pts',(-4.36391231627522,-0.768357459497397,
63.876477943877));
#55055=CARTESIAN_POINT('Ctrl Pts',(-3.80373422012026,-2.9979881039429,63.9572862499311));
#55056=CARTESIAN_POINT('Ctrl Pts',(-0.245853021615901,-5.16155116855183,
64.0910148100673));
#55057=CARTESIAN_POINT('Ctrl Pts',(4.20302825930282,-3.00609507922124,64.249775572313));
#55058=CARTESIAN_POINT('Ctrl Pts',(4.80516969413782,1.90063104898239,64.408536334559));
#55059=CARTESIAN_POINT('Ctrl Pts',(1.00947304907845,5.06784158562605,64.5672970968048));
#55060=CARTESIAN_POINT('Ctrl Pts',(-3.35112485942778,3.70870379987186,64.7139816159202));
#55061=CARTESIAN_POINT('Ctrl Pts',(-4.36188725407156,1.11753630245885,64.8077458809536));
#55062=CARTESIAN_POINT('Ctrl Pts',(-4.37221209240492,-0.00398401159164036,
64.848589891905));
#55063=CARTESIAN_POINT('Origin',(0.,0.,24.1514101080949));
#55064=CARTESIAN_POINT('',(-4.37595036350582,-0.00321178070193251,62.6514101080949));
#55065=CARTESIAN_POINT('',(-4.37457294606715,0.00364650982632456,62.848589891905));
#55066=CARTESIAN_POINT('',(-4.372,3.82579154166093E-12,24.1514101080949));
#55067=CARTESIAN_POINT('Ctrl Pts',(-4.37595036350582,-0.00321178070193263,
62.6514101080949));
#55068=CARTESIAN_POINT('Ctrl Pts',(-4.37763091892069,-0.207108192738585,
62.6588520983301));
#55069=CARTESIAN_POINT('Ctrl Pts',(-4.27203828701875,-1.85916971844638,
62.7192143426473));
#55070=CARTESIAN_POINT('Ctrl Pts',(-2.16819641913028,-4.69051998227545,
62.8324968410464));
#55071=CARTESIAN_POINT('Ctrl Pts',(2.76465101981334,-4.3656337632353,62.9912576032923));
#55072=CARTESIAN_POINT('Ctrl Pts',(5.16720539805885,-0.0451861740625634,
63.1500183655382));
#55073=CARTESIAN_POINT('Ctrl Pts',(2.8405755616569,4.31661718184185,63.308779127784));
#55074=CARTESIAN_POINT('Ctrl Pts',(-2.08583579528372,4.72772064013601,63.46753989003));
#55075=CARTESIAN_POINT('Ctrl Pts',(-4.25650552345673,1.91071093035616,63.5817502168002));
#55076=CARTESIAN_POINT('Ctrl Pts',(-4.37723401655206,0.232872448270317,
63.6430402894885));
#55077=CARTESIAN_POINT('Ctrl Pts',(-4.37524640365158,0.00345929889477663,
63.6514101080949));
#55078=CARTESIAN_POINT('Ctrl Pts',(-4.37457294606715,0.00364650982632473,
62.848589891905));
#55079=CARTESIAN_POINT('Ctrl Pts',(-4.36385410668696,-1.19462603572661,
62.8922897527186));
#55080=CARTESIAN_POINT('Ctrl Pts',(-3.23292058066413,-3.86178527014851,
62.9889098676142));
#55081=CARTESIAN_POINT('Ctrl Pts',(1.28068854395033,-5.00618527695598,63.1384502365919));
#55082=CARTESIAN_POINT('Ctrl Pts',(4.90047350742458,-1.63933327204883,63.2972109988377));
#55083=CARTESIAN_POINT('Ctrl Pts',(4.03519542999152,3.22788661752423,63.4559717610837));
#55084=CARTESIAN_POINT('Ctrl Pts',(-0.523216761619089,5.14084607765855,
63.6147325233295));
#55085=CARTESIAN_POINT('Ctrl Pts',(-3.886148042221,2.83920884682887,63.7456052336033));
#55086=CARTESIAN_POINT('Ctrl Pts',(-4.3658303620453,0.690895618159912,63.8235576897951));
#55087=CARTESIAN_POINT('Ctrl Pts',(-4.36492309298158,0.000643490633093699,
63.8485898919049));
#55088=CARTESIAN_POINT('Origin',(0.,0.,24.1514101080949));
#55089=CARTESIAN_POINT('',(-4.36526954399882,-0.00142033253192601,61.6514101080949));
#55090=CARTESIAN_POINT('',(-4.37655926179451,-0.0029470014875782,61.848589891905));
#55091=CARTESIAN_POINT('',(-4.372,3.82579154166093E-12,24.1514101080949));
#55092=CARTESIAN_POINT('Ctrl Pts',(-4.36526954399882,-0.00142033253192606,
61.6514101080949));
#55093=CARTESIAN_POINT('Ctrl Pts',(-4.36713817680575,-0.642506710603713,
61.6746639071717));
#55094=CARTESIAN_POINT('Ctrl Pts',(-3.93449886856382,-2.74015675637768,
61.7508379603305));
#55095=CARTESIAN_POINT('Ctrl Pts',(-0.695222522116061,-5.12042176590928,
61.879932267571));
#55096=CARTESIAN_POINT('Ctrl Pts',(3.92474305071123,-3.3613160223265,62.038693029817));
#55097=CARTESIAN_POINT('Ctrl Pts',(4.95266390069012,1.47416881762428,62.1974537920629));
#55098=CARTESIAN_POINT('Ctrl Pts',(1.4477554676688,4.96044932661243,62.3562145543087));
#55099=CARTESIAN_POINT('Ctrl Pts',(-3.15577720759182,3.95616660035224,62.5075333263195));
#55100=CARTESIAN_POINT('Ctrl Pts',(-4.36568043030908,1.24280635839108,62.6059318442481));
#55101=CARTESIAN_POINT('Ctrl Pts',(-4.37595036350582,-0.00321178070193263,
62.6514101080949));
#55102=CARTESIAN_POINT('Ctrl Pts',(-4.37655926179451,-0.00294700148757761,
61.848589891905));
#55103=CARTESIAN_POINT('Ctrl Pts',(-4.37795768436782,-0.183473677232841,
61.8551813074782));
#55104=CARTESIAN_POINT('Ctrl Pts',(-4.28584228404936,-1.81194987404807,
61.9146929771335));
#55105=CARTESIAN_POINT('Ctrl Pts',(-2.24311745571471,-4.65515609337478,
62.0271249008706));
#55106=CARTESIAN_POINT('Ctrl Pts',(2.69430472161155,-4.40939635788372,62.1858856631165));
#55107=CARTESIAN_POINT('Ctrl Pts',(5.16581691910958,-0.128022388891978,
62.3446464253625));
#55108=CARTESIAN_POINT('Ctrl Pts',(2.90941568030617,4.27052158090844,62.5034071876082));
#55109=CARTESIAN_POINT('Ctrl Pts',(-2.00977165837252,4.76055375508134,62.6621679498542));
#55110=CARTESIAN_POINT('Ctrl Pts',(-4.24182569275328,1.95798917979278,62.7772288512864));
#55111=CARTESIAN_POINT('Ctrl Pts',(-4.37683455314381,0.256474411491908,
62.8393694986367));
#55112=CARTESIAN_POINT('Ctrl Pts',(-4.37457294606715,0.00364650982632473,
62.848589891905));
#55113=CARTESIAN_POINT('Origin',(0.,0.,24.1514101080949));
#55114=CARTESIAN_POINT('',(-4.37074823605818,0.00396461597538121,60.6514101080949));
#55115=CARTESIAN_POINT('',(-4.36552637203463,-0.001773948386046,60.848589891905));
#55116=CARTESIAN_POINT('',(-4.372,3.82579154166093E-12,24.1514101080949));
#55117=CARTESIAN_POINT('Ctrl Pts',(-4.37074823605818,0.00396461597538186,
60.6514101080949));
#55118=CARTESIAN_POINT('Ctrl Pts',(-4.36120638422482,-1.0696402047533,60.6904757160132));
#55119=CARTESIAN_POINT('Ctrl Pts',(-3.42125648388678,-3.61254525965742,
60.7824615780135));
#55120=CARTESIAN_POINT('Ctrl Pts',(0.839052987504236,-5.09882765939536,
60.9273676940957));
#55121=CARTESIAN_POINT('Ctrl Pts',(4.73876879287487,-2.06061246810993,61.0861284563416));
#55122=CARTESIAN_POINT('Ctrl Pts',(4.30141865142892,2.86353819621711,61.2448892185875));
#55123=CARTESIAN_POINT('Ctrl Pts',(-0.0727212283482856,5.16689123545314,
61.4036499808334));
#55124=CARTESIAN_POINT('Ctrl Pts',(-3.74936971792349,3.0966186529212,61.5391569440025));
#55125=CARTESIAN_POINT('Ctrl Pts',(-4.36288560187799,0.816457216282587,
61.6217436530897));
#55126=CARTESIAN_POINT('Ctrl Pts',(-4.36526954399882,-0.00142033253192606,
61.6514101080949));
#55127=CARTESIAN_POINT('Ctrl Pts',(-4.36552637203463,-0.00177394838604503,
60.848589891905));
#55128=CARTESIAN_POINT('Ctrl Pts',(-4.36778246279527,-0.619319994324535,
60.8709931163198));
#55129=CARTESIAN_POINT('Ctrl Pts',(-3.95683545179798,-2.6927488906017,60.9463165948165));
#55130=CARTESIAN_POINT('Ctrl Pts',(-0.777225152475865,-5.10861774222493,
61.0745603273954));
#55131=CARTESIAN_POINT('Ctrl Pts',(3.87034915924295,-3.42380658907068,61.2333210896411));
#55132=CARTESIAN_POINT('Ctrl Pts',(4.97566169906822,1.39457693593507,61.3920818518871));
#55133=CARTESIAN_POINT('Ctrl Pts',(1.52709666834069,4.93660105126586,61.550842614133));
#55134=CARTESIAN_POINT('Ctrl Pts',(-3.11790932935563,4.00102289357066,61.7030119608056));
#55135=CARTESIAN_POINT('Ctrl Pts',(-4.36673022084793,1.26591415802506,61.8022610533963));
#55136=CARTESIAN_POINT('Ctrl Pts',(-4.37655926179451,-0.00294700148757761,
61.848589891905));
#55137=CARTESIAN_POINT('Origin',(0.,0.,24.1514101080949));
#55138=CARTESIAN_POINT('',(-4.37890245970854,-0.00098741172007078,59.6514101080949));
#55139=CARTESIAN_POINT('',(-4.37007084553272,0.00389455484668386,59.848589891905));
#55140=CARTESIAN_POINT('',(-4.372,3.82579154166093E-12,24.1514101080949));
#55141=CARTESIAN_POINT('Ctrl Pts',(-4.37890245970854,-0.000987411720070989,
59.6514101080949));
#55142=CARTESIAN_POINT('Ctrl Pts',(-4.37906627500205,-0.054514724532804,
59.6533672707728));
#55143=CARTESIAN_POINT('Ctrl Pts',(-4.35392740184128,-1.55522413176342,
59.7082446875327));
#55144=CARTESIAN_POINT('Ctrl Pts',(-2.6406923556686,-4.44171107781315,59.8160423583745));
#55145=CARTESIAN_POINT('Ctrl Pts',(2.29934455736468,-4.62764173446609,59.9748031206204));
#55146=CARTESIAN_POINT('Ctrl Pts',(5.13495109710383,-0.578213322578349,
60.1335638828663));
#55147=CARTESIAN_POINT('Ctrl Pts',(3.27089354364999,4.00041358388897,60.2923246451122));
#55148=CARTESIAN_POINT('Ctrl Pts',(-1.58678569169648,4.91773978415717,60.451085407358));
#55149=CARTESIAN_POINT('Ctrl Pts',(-4.15423631088884,2.21598713963915,60.5707805616856));
#55150=CARTESIAN_POINT('Ctrl Pts',(-4.37413226072698,0.384719343814296,
60.6375554619313));
#55151=CARTESIAN_POINT('Ctrl Pts',(-4.37074823605818,0.00396461597538186,
60.6514101080949));
#55152=CARTESIAN_POINT('Ctrl Pts',(-4.37007084553272,0.00389455484668389,
59.848589891905));
#55153=CARTESIAN_POINT('Ctrl Pts',(-4.36101477584936,-1.0467484993519,59.8868049251613));
#55154=CARTESIAN_POINT('Ctrl Pts',(-3.45386988791881,-3.56635453916342,
59.9779402124996));
#55155=CARTESIAN_POINT('Ctrl Pts',(0.757199388556149,-5.11162432694214,
60.12199575392));
#55156=CARTESIAN_POINT('Ctrl Pts',(4.70512351821232,-2.13632086826434,60.2807565161658));
#55157=CARTESIAN_POINT('Ctrl Pts',(4.34677488413138,2.79420870381954,60.4395172784118));
#55158=CARTESIAN_POINT('Ctrl Pts',(0.0101251021257834,5.16739311995163,
60.5982780406576));
#55159=CARTESIAN_POINT('Ctrl Pts',(-3.72252569100569,3.14370820853236,60.7346355784887));
#55160=CARTESIAN_POINT('Ctrl Pts',(-4.36245318991586,0.839429561242695,
60.8180728622378));
#55161=CARTESIAN_POINT('Ctrl Pts',(-4.36552637203463,-0.00177394838604503,
60.848589891905));
#55162=CARTESIAN_POINT('Origin',(0.,0.,24.1514101080949));
#55163=CARTESIAN_POINT('',(-4.36785354673662,-0.00333986239341869,58.6514101080949));
#55164=CARTESIAN_POINT('',(-4.37908572622912,-0.000563059365845109,58.848589891905));
#55165=CARTESIAN_POINT('',(-4.372,3.82579154166093E-12,24.1514101080949));
#55166=CARTESIAN_POINT('Ctrl Pts',(-4.36785354673662,-0.00333986239341826,
58.6514101080949));
#55167=CARTESIAN_POINT('Ctrl Pts',(-4.3713354267805,-0.492488022383476,
58.6691790796144));
#55168=CARTESIAN_POINT('Ctrl Pts',(-4.0698257693161,-2.43426901092249,58.7398683052158));
#55169=CARTESIAN_POINT('Ctrl Pts',(-1.21995052871669,-5.02133190732686,
58.8634777848992));
#55170=CARTESIAN_POINT('Ctrl Pts',(3.55689020801282,-3.74841105859499,59.022238547145));
#55171=CARTESIAN_POINT('Ctrl Pts',(5.07835637974298,0.955170087669591,59.1809993093909));
#55172=CARTESIAN_POINT('Ctrl Pts',(1.95195567231696,4.78455039364876,59.3397600716368));
#55173=CARTESIAN_POINT('Ctrl Pts',(-2.90036961753982,4.24173919554959,59.4965636712048));
#55174=CARTESIAN_POINT('Ctrl Pts',(-4.37463682871597,1.39282484839483,59.6004470166909));
#55175=CARTESIAN_POINT('Ctrl Pts',(-4.37890245970854,-0.000987411720070989,
59.6514101080949));
#55176=CARTESIAN_POINT('Ctrl Pts',(-4.37908572622912,-0.000563059365844233,
58.848589891905));
#55177=CARTESIAN_POINT('Ctrl Pts',(-4.37914057971478,-0.0308242308936409,
58.8496964799209));
#55178=CARTESIAN_POINT('Ctrl Pts',(-4.36515029335745,-1.50821048731078,
58.9037233220189));
#55179=CARTESIAN_POINT('Ctrl Pts',(-2.71156370034918,-4.39880398208026,
59.0106704181988));
#55180=CARTESIAN_POINT('Ctrl Pts',(2.22485747409188,-4.66391074033302,59.1694311804446));
#55181=CARTESIAN_POINT('Ctrl Pts',(5.12502112908765,-0.660463928024547,
59.3281919426906));
#55182=CARTESIAN_POINT('Ctrl Pts',(3.33460890093368,3.94745964534539,59.4869527049363));
#55183=CARTESIAN_POINT('Ctrl Pts',(-1.5077392503099,4.94254757457034,59.6457134671823));
#55184=CARTESIAN_POINT('Ctrl Pts',(-4.13672535981933,2.2634000371691,59.7662591961718));
#55185=CARTESIAN_POINT('Ctrl Pts',(-4.37355563916387,0.408184092349566,
59.8338846710794));
#55186=CARTESIAN_POINT('Ctrl Pts',(-4.37007084553272,0.00389455484668389,
59.848589891905));
#55187=CARTESIAN_POINT('Origin',(0.,0.,24.1514101080949));
#55188=CARTESIAN_POINT('',(-4.36690348533115,0.0028923709500598,57.6514101080949));
#55189=CARTESIAN_POINT('',(-4.36842637263245,-0.00353866609716813,57.848589891905));
#55190=CARTESIAN_POINT('',(-4.372,3.82579154166093E-12,24.1514101080949));
#55191=CARTESIAN_POINT('Ctrl Pts',(-4.36690348533115,0.00289237095005987,
57.6514101080949));
#55192=CARTESIAN_POINT('Ctrl Pts',(-4.36128421030265,-0.922032505654121,
57.6849908884559));
#55193=CARTESIAN_POINT('Ctrl Pts',(-3.62122223271516,-3.31277225264101,
57.7714919228989));
#55194=CARTESIAN_POINT('Ctrl Pts',(0.308361079608735,-5.1581941472416,57.9109132114238));
#55195=CARTESIAN_POINT('Ctrl Pts',(4.50080518836808,-2.53866226040682,58.0696739736697));
#55196=CARTESIAN_POINT('Ctrl Pts',(4.57397490984839,2.40433087160068,58.2284347359156));
#55197=CARTESIAN_POINT('Ctrl Pts',(0.460903079952699,5.14680694867653,58.3871954981615));
#55198=CARTESIAN_POINT('Ctrl Pts',(-3.56644148611271,3.39903679271645,58.5281872888879));
#55199=CARTESIAN_POINT('Ctrl Pts',(-4.36096555385885,0.964312382866099,
58.6162588255324));
#55200=CARTESIAN_POINT('Ctrl Pts',(-4.36785354673662,-0.00333986239341826,
58.6514101080949));
#55201=CARTESIAN_POINT('Ctrl Pts',(-4.36842637263245,-0.00353866609716848,
57.848589891905));
#55202=CARTESIAN_POINT('Ctrl Pts',(-4.37197022738872,-0.469118111917197,
57.8655082887625));
#55203=CARTESIAN_POINT('Ctrl Pts',(-4.08900712877109,-2.3868217079302,57.935346939702));
#55204=CARTESIAN_POINT('Ctrl Pts',(-1.30029709065152,-5.00112803773905,
58.0581058447233));
#55205=CARTESIAN_POINT('Ctrl Pts',(3.49633757827368,-3.80495436405849,58.2168666069693));
#55206=CARTESIAN_POINT('Ctrl Pts',(5.09301729854088,0.873629767452735,58.3756273692151));
#55207=CARTESIAN_POINT('Ctrl Pts',(2.02841201894453,4.75264125042254,58.5343881314611));
#55208=CARTESIAN_POINT('Ctrl Pts',(-2.85835725119982,4.28517149950547,58.6920423056909));
#55209=CARTESIAN_POINT('Ctrl Pts',(-4.37651732665532,1.41635291451315,58.796776225839));
#55210=CARTESIAN_POINT('Ctrl Pts',(-4.37908572622912,-0.000563059365844233,
58.848589891905));
#55211=CARTESIAN_POINT('Origin',(0.,0.,24.1514101080949));
#55212=CARTESIAN_POINT('',(-4.37833561871486,0.00173199218209078,56.6514101080949));
#55213=CARTESIAN_POINT('',(-4.36645415447485,0.00261097933498017,56.848589891905));
#55214=CARTESIAN_POINT('',(-4.372,3.82579154166093E-12,24.1514101080949));
#55215=CARTESIAN_POINT('Ctrl Pts',(-4.37833561871486,0.00173199218209092,
56.6514101080949));
#55216=CARTESIAN_POINT('Ctrl Pts',(-4.3715252071243,-1.34959412873374,56.7008026972975));
#55217=CARTESIAN_POINT('Ctrl Pts',(-2.97623248528167,-4.16090558093235,
56.803115540582));
#55218=CARTESIAN_POINT('Ctrl Pts',(1.8094827870843,-4.8402298973603,56.9583486379485));
#55219=CARTESIAN_POINT('Ctrl Pts',(5.04785929713791,-1.10506557830443,57.1171094001944));
#55220=CARTESIAN_POINT('Ctrl Pts',(3.66628078958101,3.64148851268323,57.2758701624403));
#55221=CARTESIAN_POINT('Ctrl Pts',(-1.07078988460527,5.05524108614831,57.4346309246862));
#55222=CARTESIAN_POINT('Ctrl Pts',(-4.03315651405818,2.52188158975817,57.559810906571));
#55223=CARTESIAN_POINT('Ctrl Pts',(-4.37013967640761,0.535564934025079,
57.632070634374));
#55224=CARTESIAN_POINT('Ctrl Pts',(-4.36690348533115,0.00289237095005987,
57.6514101080949));
#55225=CARTESIAN_POINT('Ctrl Pts',(-4.36645415447485,0.00261097933498031,
56.848589891905));
#55226=CARTESIAN_POINT('Ctrl Pts',(-4.36154135054989,-0.899119064739272,
56.881320097604));
#55227=CARTESIAN_POINT('Ctrl Pts',(-3.65007828630307,-3.26593148213623,
56.9669705573851));
#55228=CARTESIAN_POINT('Ctrl Pts',(0.225623900899773,-5.162474990657,57.1055412712481));
#55229=CARTESIAN_POINT('Ctrl Pts',(4.45952627223033,-2.61049412968195,57.2643020334939));
#55230=CARTESIAN_POINT('Ctrl Pts',(4.61193398121205,2.33069069735948,57.4230627957398));
#55231=CARTESIAN_POINT('Ctrl Pts',(0.543358837230748,5.13875620630321,57.5818235579857));
#55232=CARTESIAN_POINT('Ctrl Pts',(-3.53595095853239,3.44562506237492,57.7236659233741));
#55233=CARTESIAN_POINT('Ctrl Pts',(-4.36088515262005,0.98720087478414,57.8125880346805));
#55234=CARTESIAN_POINT('Ctrl Pts',(-4.36842637263245,-0.00353866609716848,
57.848589891905));
#55235=CARTESIAN_POINT('Origin',(0.,0.,24.1514101080949));
#55236=CARTESIAN_POINT('',(-4.37203889039062,-0.00399078471529107,55.6514101080949));
#55237=CARTESIAN_POINT('',(-4.37792086111113,0.00210556704416318,55.848589891905));
#55238=CARTESIAN_POINT('',(-4.372,3.82579154166093E-12,24.1514101080949));
#55239=CARTESIAN_POINT('Ctrl Pts',(-4.37203889039062,-0.0039907847152907,
55.6514101080949));
#55240=CARTESIAN_POINT('Ctrl Pts',(-4.37513795036318,-0.341330640933386,
55.6636942520571));
#55241=CARTESIAN_POINT('Ctrl Pts',(-4.18538392269166,-2.12848606629693,
55.7288986501012));
#55242=CARTESIAN_POINT('Ctrl Pts',(-1.7316503614075,-4.86861791907028,55.8470233022273));
#55243=CARTESIAN_POINT('Ctrl Pts',(3.15105239533607,-4.09547582313724,56.0057840644731));
#55244=CARTESIAN_POINT('Ctrl Pts',(5.14981574971942,0.425970844068908,56.1645448267191));
#55245=CARTESIAN_POINT('Ctrl Pts',(2.43531042678924,4.55755598333432,56.3233055889649));
#55246=CARTESIAN_POINT('Ctrl Pts',(-2.50806538626398,4.517926674292,56.4820663512109));
#55247=CARTESIAN_POINT('Ctrl Pts',(-4.33218063910257,1.64211842271798,56.5914345242541));
#55248=CARTESIAN_POINT('Ctrl Pts',(-4.37882202467515,0.0982449665847532,
56.6478824432155));
#55249=CARTESIAN_POINT('Ctrl Pts',(-4.37833561871486,0.00173199218209092,
56.6514101080949));
#55250=CARTESIAN_POINT('Ctrl Pts',(-4.37792086111113,0.00210556704416347,
55.848589891905));
#55251=CARTESIAN_POINT('Ctrl Pts',(-4.37002924341455,-1.32628327647185,
55.8971319064456));
#55252=CARTESIAN_POINT('Ctrl Pts',(-3.01639925320847,-4.11679727890053,
55.9985941750683));
#55253=CARTESIAN_POINT('Ctrl Pts',(1.73165038597632,-4.86861798815274,56.1529766977727));
#55254=CARTESIAN_POINT('Ctrl Pts',(5.02949388480597,-1.18585219842773,56.3117374600186));
#55255=CARTESIAN_POINT('Ctrl Pts',(3.72419095237009,3.58224174562538,56.4704982222645));
#55256=CARTESIAN_POINT('Ctrl Pts',(-0.989605296568694,5.07175862308326,
56.6292589845104));
#55257=CARTESIAN_POINT('Ctrl Pts',(-4.01260884555851,2.56932936205486,56.7552895410572));
#55258=CARTESIAN_POINT('Ctrl Pts',(-4.36948468076768,0.558854755667328,
56.8283998435221));
#55259=CARTESIAN_POINT('Ctrl Pts',(-4.36645415447485,0.00261097933498031,
56.848589891905));
#55260=CARTESIAN_POINT('Origin',(0.,0.,24.1514101080949));
#55261=CARTESIAN_POINT('',(-4.36494997391578,0.000736207605459677,54.651410108095));
#55262=CARTESIAN_POINT('',(-4.37274842293649,-0.00394778047225652,54.848589891905));
#55263=CARTESIAN_POINT('',(-4.372,3.82579154166093E-12,24.1514101080949));
#55264=CARTESIAN_POINT('Ctrl Pts',(-4.36494997391578,0.000736207605459838,
54.651410108095));
#55265=CARTESIAN_POINT('Ctrl Pts',(-4.36378453680234,-0.773985575709198,
54.6795060608986));
#55266=CARTESIAN_POINT('Ctrl Pts',(-3.79750074957444,-3.0095293451424,54.7605222677843));
#55267=CARTESIAN_POINT('Ctrl Pts',(-0.22562389770033,-5.16247491740555,
54.8944587287519));
#55268=CARTESIAN_POINT('Ctrl Pts',(4.21477629650059,-2.98960100791253,55.0532194909978));
#55269=CARTESIAN_POINT('Ctrl Pts',(4.79768448212587,1.91944706257383,55.2119802532437));
#55270=CARTESIAN_POINT('Ctrl Pts',(0.989605282528937,5.07175855111871,55.3707410154895));
#55271=CARTESIAN_POINT('Ctrl Pts',(-3.35946002969715,3.69749334286384,55.5172176337734));
#55272=CARTESIAN_POINT('Ctrl Pts',(-4.36178715915881,1.11193390546508,55.6107739979751));
#55273=CARTESIAN_POINT('Ctrl Pts',(-4.37203889039062,-0.0039907847152907,
55.6514101080949));
#55274=CARTESIAN_POINT('Ctrl Pts',(-4.37274842293649,-0.00394778047225635,
54.848589891905));
#55275=CARTESIAN_POINT('Ctrl Pts',(-4.37564665776889,-0.317799192266558,
54.8600234612052));
#55276=CARTESIAN_POINT('Ctrl Pts',(-4.20162062889501,-2.08112280559727,
54.9243772845874));
#55277=CARTESIAN_POINT('Ctrl Pts',(-1.80948281276126,-4.84022996603858,
55.0416513620516));
#55278=CARTESIAN_POINT('Ctrl Pts',(3.08498768485217,-4.1454680264268,55.2004121242973));
#55279=CARTESIAN_POINT('Ctrl Pts',(5.15598322111311,0.34335287594041,55.3591728865433));
#55280=CARTESIAN_POINT('Ctrl Pts',(2.50806542185317,4.51792673839683,55.5179336487891));
#55281=CARTESIAN_POINT('Ctrl Pts',(-2.43531046134262,4.55755604800332,55.6766944110351));
#55282=CARTESIAN_POINT('Ctrl Pts',(-4.31984022389642,1.68922674479917,55.7869131587403));
#55283=CARTESIAN_POINT('Ctrl Pts',(-4.37863264435646,0.121919394632788,
55.8442116523636));
#55284=CARTESIAN_POINT('Ctrl Pts',(-4.37792086111113,0.00210556704416347,
55.848589891905));
#55285=CARTESIAN_POINT('Origin',(0.,0.,24.1514101080949));
#55286=CARTESIAN_POINT('',(-4.37473956626258,0.00360433591460132,53.6514101080949));
#55287=CARTESIAN_POINT('',(-4.36486283016371,0.00035491530368581,53.848589891905));
#55288=CARTESIAN_POINT('',(-4.372,3.82579154166093E-12,24.1514101080949));
#55289=CARTESIAN_POINT('Ctrl Pts',(-4.37473956626258,0.00360433591460166,
53.6514101080949));
#55290=CARTESIAN_POINT('Ctrl Pts',(-4.36404265119134,-1.20025020685171,
53.6953178697402));
#55291=CARTESIAN_POINT('Ctrl Pts',(-3.22404333927935,-3.87285840602707,
53.7921458854674));
#55292=CARTESIAN_POINT('Ctrl Pts',(1.30029707219943,-5.00112796677752,53.9418941552766));
#55293=CARTESIAN_POINT('Ctrl Pts',(4.90686007449561,-1.62011654684958,54.1006549175225));
#55294=CARTESIAN_POINT('Ctrl Pts',(4.02251485462088,3.2436750238594,54.2594156797684));
#55295=CARTESIAN_POINT('Ctrl Pts',(-0.543358829519001,5.13875613338857,
54.4181764420142));
#55296=CARTESIAN_POINT('Ctrl Pts',(-3.89191662696183,2.82763508414209,54.5488412514565));
#55297=CARTESIAN_POINT('Ctrl Pts',(-4.3659797009454,0.685245008222085,54.6265858068167));
#55298=CARTESIAN_POINT('Ctrl Pts',(-4.36494997391578,0.000736207605459838,
54.651410108095));
#55299=CARTESIAN_POINT('Ctrl Pts',(-4.36486283016371,0.000354915303685741,
53.848589891905));
#55300=CARTESIAN_POINT('Ctrl Pts',(-4.36431860610875,-0.750950458311704,
53.8758352700467));
#55301=CARTESIAN_POINT('Ctrl Pts',(-3.82280092431587,-2.96229440941745,
53.9560009022705));
#55302=CARTESIAN_POINT('Ctrl Pts',(-0.308361083986154,-5.15819422043212,
54.0890867885761));
#55303=CARTESIAN_POINT('Ctrl Pts',(4.16630456733569,-3.05678923480409,54.2478475508221));
#55304=CARTESIAN_POINT('Ctrl Pts',(4.82784101720183,1.84228262935957,54.4066083130679));
#55305=CARTESIAN_POINT('Ctrl Pts',(1.07078989980086,5.0552411578777,54.5653690753139));
#55306=CARTESIAN_POINT('Ctrl Pts',(-3.3251283689399,3.74330363517374,54.7126962682595));
#55307=CARTESIAN_POINT('Ctrl Pts',(-4.36223218327779,1.13486147913407,54.8071032071232));
#55308=CARTESIAN_POINT('Ctrl Pts',(-4.37274842293649,-0.00394778047225635,
54.848589891905));
#55309=CARTESIAN_POINT('Origin',(0.,0.,24.1514101080949));
#55310=CARTESIAN_POINT('',(-4.37641405919053,-0.00301495007056918,52.6514101080949));
#55311=CARTESIAN_POINT('',(-4.37405090679819,0.00376197565890995,52.848589891905));
#55312=CARTESIAN_POINT('',(-4.372,3.82579154166093E-12,24.1514101080949));
#55313=CARTESIAN_POINT('Ctrl Pts',(-4.37641405919053,-0.00301495007056837,
52.651410108095));
#55314=CARTESIAN_POINT('Ctrl Pts',(-4.37788112208874,-0.189251796122769,
52.6582094244998));
#55315=CARTESIAN_POINT('Ctrl Pts',(-4.28250642368832,-1.82348881026957,
52.7179289949866));
#55316=CARTESIAN_POINT('Ctrl Pts',(-2.22485744252472,-4.66391067415503,
52.8305688195554));
#55317=CARTESIAN_POINT('Ctrl Pts',(2.71156366187259,-4.39880391966578,52.9893295818012));
#55318=CARTESIAN_POINT('Ctrl Pts',(5.16627887713359,-0.107777454683187,
53.1480903440472));
#55319=CARTESIAN_POINT('Ctrl Pts',(2.89265785799892,4.28189022893068,53.306851106293));
#55320=CARTESIAN_POINT('Ctrl Pts',(-2.02841199016113,4.75264118298715,53.4656118685389));
#55321=CARTESIAN_POINT('Ctrl Pts',(-4.24545291415805,1.94643078465362,53.5804648691395));
#55322=CARTESIAN_POINT('Ctrl Pts',(-4.37693521146432,0.250707115811383,
53.6423976156582));
#55323=CARTESIAN_POINT('Ctrl Pts',(-4.37473956626258,0.00360433591460166,
53.6514101080949));
#55324=CARTESIAN_POINT('Ctrl Pts',(-4.37405090679819,0.00376197565890985,
52.848589891905));
#55325=CARTESIAN_POINT('Ctrl Pts',(-4.36331136726339,-1.17725226132736,
52.8916470788883));
#55326=CARTESIAN_POINT('Ctrl Pts',(-3.26012737634599,-3.8274917595608,52.9876245199536));
#55327=CARTESIAN_POINT('Ctrl Pts',(1.21995054602492,-5.021331978576,53.1365222151008));
#55328=CARTESIAN_POINT('Ctrl Pts',(4.88025534693686,-1.69857643999627,53.2952829773467));
#55329=CARTESIAN_POINT('Ctrl Pts',(4.07400138499168,3.17876814016096,53.4540437395925));
#55330=CARTESIAN_POINT('Ctrl Pts',(-0.460903086490536,5.14680702170578,
53.6128045018385));
#55331=CARTESIAN_POINT('Ctrl Pts',(-3.86811921206171,2.87497489714133,53.7443198859426));
#55332=CARTESIAN_POINT('Ctrl Pts',(-4.365375683574,0.708352879597865,53.8229150159648));
#55333=CARTESIAN_POINT('Ctrl Pts',(-4.36486283016371,0.000354915303685741,
53.848589891905));
#55334=CARTESIAN_POINT('Origin',(0.,0.,24.1514101080949));
#55335=CARTESIAN_POINT('',(-4.36545824626946,-0.00168887658937792,51.651410108095));
#55336=CARTESIAN_POINT('',(-4.37699111974124,-0.00272425946348631,51.848589891905));
#55337=CARTESIAN_POINT('',(-4.372,3.82579154166093E-12,24.1514101080949));
#55338=CARTESIAN_POINT('Ctrl Pts',(-4.36545824626946,-0.00168887658937779,
51.651410108095));
#55339=CARTESIAN_POINT('Ctrl Pts',(-4.36762412827266,-0.624989998325019,
51.6740212333413));
#55340=CARTESIAN_POINT('Ctrl Pts',(-3.95142248851676,-2.70433810681889,
51.7495526126697));
#55341=CARTESIAN_POINT('Ctrl Pts',(-0.757199377814005,-5.111624254412,51.87800424608));
#55342=CARTESIAN_POINT('Ctrl Pts',(3.88373669535471,-3.40861301664037,52.0367650083259));
#55343=CARTESIAN_POINT('Ctrl Pts',(4.97015831465276,1.41406497140078,52.1955257705718));
#55344=CARTESIAN_POINT('Ctrl Pts',(1.50773922891819,4.94254750443899,52.3542865328176));
#55345=CARTESIAN_POINT('Ctrl Pts',(-3.12722350039883,3.99007665346195,52.5062479786588));
#55346=CARTESIAN_POINT('Ctrl Pts',(-4.36646271813384,1.26026174695854,52.6052891704178));
#55347=CARTESIAN_POINT('Ctrl Pts',(-4.37641405919053,-0.00301495007056837,
52.651410108095));
#55348=CARTESIAN_POINT('Ctrl Pts',(-4.37699111974124,-0.00272425946348602,
51.848589891905));
#55349=CARTESIAN_POINT('Ctrl Pts',(-4.37818018489292,-0.165607164620367,
51.8545386336479));
#55350=CARTESIAN_POINT('Ctrl Pts',(-4.29599872620153,-1.77629134844302,
51.9134076294728));
#55351=CARTESIAN_POINT('Ctrl Pts',(-2.2993445899923,-4.62764180012773,52.0251968793796));
#55352=CARTESIAN_POINT('Ctrl Pts',(2.64069239313623,-4.44171114083851,52.1839576416255));
#55353=CARTESIAN_POINT('Ctrl Pts',(5.16388703706709,-0.190590771620509,
52.3427184038713));
#55354=CARTESIAN_POINT('Ctrl Pts',(2.96093453169081,4.23496409345547,52.5014791661172));
#55355=CARTESIAN_POINT('Ctrl Pts',(-1.95195570001178,4.78455046153847,52.6602399283632));
#55356=CARTESIAN_POINT('Ctrl Pts',(-4.23045159262607,1.99372864599193,52.7759435036257));
#55357=CARTESIAN_POINT('Ctrl Pts',(-4.37651100246309,0.274295735060812,
52.8387268248063));
#55358=CARTESIAN_POINT('Ctrl Pts',(-4.37405090679819,0.00376197565890985,
52.848589891905));
#55359=CARTESIAN_POINT('Origin',(0.,0.,24.1514101080949));
#55360=CARTESIAN_POINT('',(-4.3702345064702,0.00391522497022664,50.651410108095));
#55361=CARTESIAN_POINT('',(-4.36575804463348,-0.0020306512688445,50.848589891905));
#55362=CARTESIAN_POINT('',(-4.372,3.82579154166093E-12,24.1514101080949));
#55363=CARTESIAN_POINT('Ctrl Pts',(-4.3702345064702,0.00391522497022637,
50.651410108095));
#55364=CARTESIAN_POINT('Ctrl Pts',(-4.36105392339508,-1.0523431449496,50.6898330421829));
#55365=CARTESIAN_POINT('Ctrl Pts',(-3.44595349118066,-3.57765592823792,
50.7811762303528));
#55366=CARTESIAN_POINT('Ctrl Pts',(0.777225141445664,-5.10861766973804,
50.9254396726047));
#55367=CARTESIAN_POINT('Ctrl Pts',(4.71345919711634,-2.11786586288516,51.0842004348506));
#55368=CARTESIAN_POINT('Ctrl Pts',(4.33579142110028,2.81122147273531,51.2429611970965));
#55369=CARTESIAN_POINT('Ctrl Pts',(-0.0101251019801382,5.16739304663044,
51.4017219593423));
#55370=CARTESIAN_POINT('Ctrl Pts',(-3.72913776533524,3.13220382459871,51.5378715963418));
#55371=CARTESIAN_POINT('Ctrl Pts',(-4.36255498533209,0.833816380056773,
51.6211009792594));
#55372=CARTESIAN_POINT('Ctrl Pts',(-4.36545824626946,-0.00168887658937779,
51.651410108095));
#55373=CARTESIAN_POINT('Ctrl Pts',(-4.36575804463348,-0.00203065126884408,
50.848589891905));
#55374=CARTESIAN_POINT('Ctrl Pts',(-4.36827427270984,-0.601781773597835,
50.8703504424894));
#55375=CARTESIAN_POINT('Ctrl Pts',(-3.97337829241374,-2.65691780935309,
50.9450312471558));
#55376=CARTESIAN_POINT('Ctrl Pts',(-0.839052999411725,-5.09882773174331,
51.0726323059043));
#55377=CARTESIAN_POINT('Ctrl Pts',(3.82858979556074,-3.47044008032763,51.2313930681501));
#55378=CARTESIAN_POINT('Ctrl Pts',(4.99219026383802,1.33420033857639,51.390153830396));
#55379=CARTESIAN_POINT('Ctrl Pts',(1.58678571421362,4.91773985393535,51.548914592642));
#55380=CARTESIAN_POINT('Ctrl Pts',(-3.08887708143298,4.03478571508497,51.7017266131449));
#55381=CARTESIAN_POINT('Ctrl Pts',(-4.36760221182464,1.28340593748707,51.8016183795659));
#55382=CARTESIAN_POINT('Ctrl Pts',(-4.37699111974124,-0.00272425946348602,
51.848589891905));
#55383=CARTESIAN_POINT('Origin',(0.,0.,24.1514101080949));
#55384=CARTESIAN_POINT('',(-4.3790496246733,-0.000667733410364872,49.651410108095));
#55385=CARTESIAN_POINT('',(-4.36957357182231,0.00381643768188569,49.848589891905));
#55386=CARTESIAN_POINT('',(-4.372,3.82579154166093E-12,24.1514101080949));
#55387=CARTESIAN_POINT('Ctrl Pts',(-4.3790496246733,-0.000667733410364751,
49.651410108095));
#55388=CARTESIAN_POINT('Ctrl Pts',(-4.37912616480055,-0.0366150338825652,
49.6527245969425));
#55389=CARTESIAN_POINT('Ctrl Pts',(-4.36244279655587,-1.51969860268292,
49.706959339872));
#55390=CARTESIAN_POINT('Ctrl Pts',(-2.69430468338317,-4.40939629531691,
49.8141143368835));
#55391=CARTESIAN_POINT('Ctrl Pts',(2.2431174238849,-4.6551560273227,49.9728750991294));
#55392=CARTESIAN_POINT('Ctrl Pts',(5.12756994789964,-0.640374769530455,
50.1316358613752));
#55393=CARTESIAN_POINT('Ctrl Pts',(3.31911383193326,3.96049703783808,50.2903966236212));
#55394=CARTESIAN_POINT('Ctrl Pts',(-1.52709664667054,4.93660098122003,50.4491573858669));
#55395=CARTESIAN_POINT('Ctrl Pts',(-4.14104743841719,2.25180987009099,50.569495214025));
#55396=CARTESIAN_POINT('Ctrl Pts',(-4.37369842336595,0.402451046051582,
50.636912788101));
#55397=CARTESIAN_POINT('Ctrl Pts',(-4.3702345064702,0.00391522497022637,
50.651410108095));
#55398=CARTESIAN_POINT('Ctrl Pts',(-4.36957357182231,0.00381643768188559,
49.848589891905));
#55399=CARTESIAN_POINT('Ctrl Pts',(-4.36092390126923,-1.02945575440987,
49.886162251331));
#55400=CARTESIAN_POINT('Ctrl Pts',(-3.47811671755736,-3.53137427358546,
49.976654864839));
#55401=CARTESIAN_POINT('Ctrl Pts',(0.695222531978707,-5.12042183856424,
50.1200677324289));
#55402=CARTESIAN_POINT('Ctrl Pts',(4.67889927324325,-2.19316113513354,50.2788284946747));
#55403=CARTESIAN_POINT('Ctrl Pts',(4.38030448079635,2.74134763015048,50.4375892569207));
#55404=CARTESIAN_POINT('Ctrl Pts',(0.0727212293821569,5.16689130876717,
50.5963500191666));
#55405=CARTESIAN_POINT('Ctrl Pts',(-3.70187703653703,3.1792474229629,50.733350230828));
#55406=CARTESIAN_POINT('Ctrl Pts',(-4.36215496848489,0.85677423381658,50.8174301884075));
#55407=CARTESIAN_POINT('Ctrl Pts',(-4.36575804463348,-0.00203065126884408,
50.848589891905));
#55408=CARTESIAN_POINT('Origin',(0.,0.,24.1514101080949));
#55409=CARTESIAN_POINT('',(-4.36828286829859,-0.0034930826256922,48.651410108095));
#55410=CARTESIAN_POINT('',(-4.37915940465982,-0.00023684953408154,48.848589891905));
#55411=CARTESIAN_POINT('',(-4.372,3.82579154166093E-12,24.1514101080949));
#55412=CARTESIAN_POINT('Ctrl Pts',(-4.36828286829859,-0.00349308262569223,
48.651410108095));
#55413=CARTESIAN_POINT('Ctrl Pts',(-4.37181608551705,-0.47483281190334,
48.6685364057841));
#55414=CARTESIAN_POINT('Ctrl Pts',(-4.08436231910608,-2.39841849396994,
48.7385829575551));
#55415=CARTESIAN_POINT('Ctrl Pts',(-1.2806885257803,-5.00618520592171,48.8615497634081));
#55416=CARTESIAN_POINT('Ctrl Pts',(3.51122164426531,-3.79122354667958,49.020310525654));
#55417=CARTESIAN_POINT('Ctrl Pts',(5.0895545138177,0.893581706914796,49.1790712878999));
#55418=CARTESIAN_POINT('Ctrl Pts',(2.00977162985725,4.76055368753214,49.3378320501457));
#55419=CARTESIAN_POINT('Ctrl Pts',(-2.86868632585708,4.274578831514,49.4952783235442));
#55420=CARTESIAN_POINT('Ctrl Pts',(-4.37604472140215,1.41059410609646,49.5998043428605));
#55421=CARTESIAN_POINT('Ctrl Pts',(-4.3790496246733,-0.000667733410364751,
49.651410108095));
#55422=CARTESIAN_POINT('Ctrl Pts',(-4.37915940465982,-0.000236849534081855,
48.848589891905));
#55423=CARTESIAN_POINT('Ctrl Pts',(-4.37916937864932,-0.0129226461636581,
48.8490538060906));
#55424=CARTESIAN_POINT('Ctrl Pts',(-4.37337449519616,-1.47271062880396,
48.9024379743582));
#55425=CARTESIAN_POINT('Ctrl Pts',(-2.76465105904324,-4.36563382517906,
49.0087423967076));
#55426=CARTESIAN_POINT('Ctrl Pts',(2.16819644989342,-4.69052004883103,49.1675031589536));
#55427=CARTESIAN_POINT('Ctrl Pts',(5.11664433946473,-0.72249904999246,49.3262639211995));
#55428=CARTESIAN_POINT('Ctrl Pts',(3.38218303962157,3.90677514842007,49.4850246834453));
#55429=CARTESIAN_POINT('Ctrl Pts',(-1.44775548820939,4.96044939699782,49.6437854456913));
#55430=CARTESIAN_POINT('Ctrl Pts',(-4.12319150304179,2.29923281750856,49.7649738485111));
#55431=CARTESIAN_POINT('Ctrl Pts',(-4.37310686689576,0.425896738132308,
49.833241997249));
#55432=CARTESIAN_POINT('Ctrl Pts',(-4.36957357182231,0.00381643768188559,
49.848589891905));
#55433=CARTESIAN_POINT('Origin',(0.,0.,24.1514101080949));
#55434=CARTESIAN_POINT('',(-4.36655943089002,0.00268207779483023,47.651410108095));
#55435=CARTESIAN_POINT('',(-4.36888289277856,-0.00366680700230215,47.848589891905));
#55436=CARTESIAN_POINT('',(-4.372,3.82579154166093E-12,24.1514101080949));
#55437=CARTESIAN_POINT('Ctrl Pts',(-4.36655943089002,0.00268207779483047,
47.651410108095));
#55438=CARTESIAN_POINT('Ctrl Pts',(-4.36147330371707,-0.90472081724388,
47.6843482146256));
#55439=CARTESIAN_POINT('Ctrl Pts',(-3.64307749349284,-3.2773877690834,47.7702065752383));
#55440=CARTESIAN_POINT('Ctrl Pts',(0.245853018125491,-5.16155109531365,
47.9089851899327));
#55441=CARTESIAN_POINT('Ctrl Pts',(4.46972204405066,-2.59299792999961,48.0677459521787));
#55442=CARTESIAN_POINT('Ctrl Pts',(4.60276492582317,2.34874614500311,48.2265067144246));
#55443=CARTESIAN_POINT('Ctrl Pts',(0.523216754197009,5.14084600471386,48.3852674766704));
#55444=CARTESIAN_POINT('Ctrl Pts',(-3.54345722553092,3.4342468351364,48.5269019412272));
#55445=CARTESIAN_POINT('Ctrl Pts',(-4.36089844550389,0.981606792564894,
48.6156161517021));
#55446=CARTESIAN_POINT('Ctrl Pts',(-4.36828286829859,-0.00349308262569223,
48.651410108095));
#55447=CARTESIAN_POINT('Ctrl Pts',(-4.36888289277856,-0.00366680700230278,
47.848589891905));
#55448=CARTESIAN_POINT('Ctrl Pts',(-4.37244155465394,-0.451442255901039,
47.8648656149322));
#55449=CARTESIAN_POINT('Ctrl Pts',(-4.10318789366455,-2.35097548418382,
47.9340615920413));
#55450=CARTESIAN_POINT('Ctrl Pts',(-1.36078444624568,-4.98500951500319,
48.0561778232324));
#55451=CARTESIAN_POINT('Ctrl Pts',(3.44998850215064,-3.84702917961962,48.2149385854782));
#55452=CARTESIAN_POINT('Ctrl Pts',(5.10322659210776,0.811869769988193,48.3736993477241));
#55453=CARTESIAN_POINT('Ctrl Pts',(2.08583582488191,4.72772070721777,48.53246010997));
#55454=CARTESIAN_POINT('Ctrl Pts',(-2.82618015492052,4.31781852687336,48.6907569580302));
#55455=CARTESIAN_POINT('Ctrl Pts',(-4.37803161206443,1.43418891395024,48.7961335520086));
#55456=CARTESIAN_POINT('Ctrl Pts',(-4.37915940465982,-0.000236849534081855,
48.848589891905));
#55457=CARTESIAN_POINT('Origin',(0.,0.,24.1514101080949));
#55458=CARTESIAN_POINT('',(-4.37802849378088,0.00201652107500087,46.651410108095));
#55459=CARTESIAN_POINT('',(-4.36614763918315,0.00238232933584437,46.848589891905));
#55460=CARTESIAN_POINT('',(-4.372,3.82579154166093E-12,24.1514101080949));
#55461=CARTESIAN_POINT('Ctrl Pts',(-4.37802849378088,0.00201652107500106,
46.651410108095));
#55462=CARTESIAN_POINT('Ctrl Pts',(-4.37038284048536,-1.33197484216078,
46.7001600234672));
#55463=CARTESIAN_POINT('Ctrl Pts',(-3.00664095593531,-4.12759897737828,
46.8018301929213));
#55464=CARTESIAN_POINT('Ctrl Pts',(1.75071634247466,-4.86179449424254,46.9564206164574));
#55465=CARTESIAN_POINT('Ctrl Pts',(5.03410234489664,-1.16613335307792,47.1151813787034));
#55466=CARTESIAN_POINT('Ctrl Pts',(3.71012411261097,3.59680865283067,47.2739421409492));
#55467=CARTESIAN_POINT('Ctrl Pts',(-1.00947303475291,5.06784151371782,47.4327029031951));
#55468=CARTESIAN_POINT('Ctrl Pts',(-4.01767618670528,2.55773240591479,47.5585255589103));
#55469=CARTESIAN_POINT('Ctrl Pts',(-4.36964496780575,0.553164799693178,
47.6314279605436));
#55470=CARTESIAN_POINT('Ctrl Pts',(-4.36655943089002,0.00268207779483047,
47.651410108095));
#55471=CARTESIAN_POINT('Ctrl Pts',(-4.36614763918315,0.00238232933584499,
46.848589891905));
#55472=CARTESIAN_POINT('Ctrl Pts',(-4.36177165814571,-0.881797305075611,
46.8806774237737));
#55473=CARTESIAN_POINT('Ctrl Pts',(-3.67150621186276,-3.23048848803606,
46.9656852097244));
#55474=CARTESIAN_POINT('Ctrl Pts',(0.163070052891163,-5.16482936133098,
47.103613249757));
#55475=CARTESIAN_POINT('Ctrl Pts',(4.42757599841828,-2.66432448325026,47.2623740120029));
#55476=CARTESIAN_POINT('Ctrl Pts',(4.63982914812316,2.27465154475207,47.4211347742487));
#55477=CARTESIAN_POINT('Ctrl Pts',(0.605568936039063,5.13179699886122,47.5798955364947));
#55478=CARTESIAN_POINT('Ctrl Pts',(-3.51252635231322,3.4807591641629,47.7223805757134));
#55479=CARTESIAN_POINT('Ctrl Pts',(-4.36087062227061,1.00449248124495,47.8119453608502));
#55480=CARTESIAN_POINT('Ctrl Pts',(-4.36888289277856,-0.00366680700230278,
47.848589891905));
#55481=CARTESIAN_POINT('Origin',(0.,0.,24.1514101080949));
#55482=CARTESIAN_POINT('',(-4.37257478030532,-0.00396203305634906,45.651410108095));
#55483=CARTESIAN_POINT('',(-4.37756404870526,0.00237073416934012,45.848589891905));
#55484=CARTESIAN_POINT('',(-4.372,3.82579154166093E-12,24.1514101080949));
#55485=CARTESIAN_POINT('Ctrl Pts',(-4.37257478030532,-0.00396203305634935,
45.651410108095));
#55486=CARTESIAN_POINT('Ctrl Pts',(-4.3755247754399,-0.323552849206446,
45.6630515782267));
#55487=CARTESIAN_POINT('Ctrl Pts',(-4.19769260696374,-2.0926975991144,45.7276133024405));
#55488=CARTESIAN_POINT('Ctrl Pts',(-1.79050086272392,-4.84728378338218,
45.8450952807362));
#55489=CARTESIAN_POINT('Ctrl Pts',(3.1012093298518,-4.13334659912459,46.0038560429821));
#55490=CARTESIAN_POINT('Ctrl Pts',(5.15459801607478,0.363555647367575,46.162616805228));
#55491=CARTESIAN_POINT('Ctrl Pts',(2.49034114873962,4.52772066043712,46.3213775674739));
#55492=CARTESIAN_POINT('Ctrl Pts',(-2.45315200638293,4.54797742404625,46.4801383297198));
#55493=CARTESIAN_POINT('Ctrl Pts',(-4.32289330486948,1.67770933141668,46.5901491765935));
#55494=CARTESIAN_POINT('Ctrl Pts',(-4.37868254545781,0.116133556522668,
46.6472397693852));
#55495=CARTESIAN_POINT('Ctrl Pts',(-4.37802849378088,0.00201652107500106,
46.651410108095));
#55496=CARTESIAN_POINT('Ctrl Pts',(-4.37756404870526,0.00237073416934035,
45.848589891905));
#55497=CARTESIAN_POINT('Ctrl Pts',(-4.36898434288233,-1.30871296070451,
45.8964892326153));
#55498=CARTESIAN_POINT('Ctrl Pts',(-3.04632193268225,-4.08332402648612,
45.9973088274075));
#55499=CARTESIAN_POINT('Ctrl Pts',(1.67254576409749,-4.88923765436041,46.1510486762816));
#55500=CARTESIAN_POINT('Ctrl Pts',(5.01475964555148,-1.2466915701828,46.3098094385276));
#55501=CARTESIAN_POINT('Ctrl Pts',(3.76731232156889,3.53686471971598,46.4685702007735));
#55502=CARTESIAN_POINT('Ctrl Pts',(-0.928094313166731,5.08337438319113,
46.6273309630193));
#55503=CARTESIAN_POINT('Ctrl Pts',(-3.99675882839479,2.60517577302872,46.7540041933965));
#55504=CARTESIAN_POINT('Ctrl Pts',(-4.36898873016318,0.576432985076398,
46.8277571696918));
#55505=CARTESIAN_POINT('Ctrl Pts',(-4.36614763918315,0.00238232933584499,
46.848589891905));
#55506=CARTESIAN_POINT('Origin',(0.,0.,24.1514101080949));
#55507=CARTESIAN_POINT('',(-4.36487844624636,0.000448538275869127,44.651410108095));
#55508=CARTESIAN_POINT('',(-4.37328422903404,-0.00388840045026428,44.848589891905));
#55509=CARTESIAN_POINT('',(-4.372,3.82579154166093E-12,24.1514101080949));
#55510=CARTESIAN_POINT('Ctrl Pts',(-4.36487844624636,0.00044853827586927,
44.651410108095));
#55511=CARTESIAN_POINT('Ctrl Pts',(-4.36418527448618,-0.756583014477848,
44.6788633870683));
#55512=CARTESIAN_POINT('Ctrl Pts',(-3.8166662948363,-2.9738437257919,44.7592369201236));
#55513=CARTESIAN_POINT('Ctrl Pts',(-0.288144634510089,-5.15936295347187,
44.8925307072609));
#55514=CARTESIAN_POINT('Ctrl Pts',(4.17825154873217,-3.04043868735616,45.0512914695067));
#55515=CARTESIAN_POINT('Ctrl Pts',(4.8205842882194,1.86118793683688,45.2100522317526));
#55516=CARTESIAN_POINT('Ctrl Pts',(1.05097104046387,5.05939851051103,45.3688129939986));
#55517=CARTESIAN_POINT('Ctrl Pts',(-3.33357615425217,3.73211986818334,45.5159322861126));
#55518=CARTESIAN_POINT('Ctrl Pts',(-4.36211457120495,1.12925568798617,45.6101313241448));
#55519=CARTESIAN_POINT('Ctrl Pts',(-4.37257478030532,-0.00396203305634935,
45.651410108095));
#55520=CARTESIAN_POINT('Ctrl Pts',(-4.37328422903404,-0.00388840045026397,
44.848589891905));
#55521=CARTESIAN_POINT('Ctrl Pts',(-4.37601255181714,-0.300005218706897,
44.8593807873749));
#55522=CARTESIAN_POINT('Ctrl Pts',(-4.21359764945945,-2.04535030654532,
44.9230919369267));
#55523=CARTESIAN_POINT('Ctrl Pts',(-1.8679837165673,-4.81795506501003,45.0397233405604));
#55524=CARTESIAN_POINT('Ctrl Pts',(3.03454387031403,-4.18253483822383,45.1984841028063));
#55525=CARTESIAN_POINT('Ctrl Pts',(5.15976421573454,0.280869029694986,45.3572448650522));
#55526=CARTESIAN_POINT('Ctrl Pts',(2.56261074386464,4.4872129823807,45.5160056272982));
#55527=CARTESIAN_POINT('Ctrl Pts',(-2.37992235675453,4.58672254988638,45.6747663895439));
#55528=CARTESIAN_POINT('Ctrl Pts',(-4.31025055648257,1.72484198053187,45.7856278110796));
#55529=CARTESIAN_POINT('Ctrl Pts',(-4.37846339218375,0.139801386813307,
45.8435689785333));
#55530=CARTESIAN_POINT('Ctrl Pts',(-4.37756404870526,0.00237073416934035,
45.848589891905));
#55531=CARTESIAN_POINT('Origin',(0.,0.,24.1514101080949));
#55532=CARTESIAN_POINT('',(-4.37422072754471,0.00372710199133062,43.651410108095));
#55533=CARTESIAN_POINT('',(-4.36483752583336,6.45211600033835E-5,43.848589891905));
#55534=CARTESIAN_POINT('',(-4.372,3.82579154166093E-12,24.1514101080949));
#55535=CARTESIAN_POINT('Ctrl Pts',(-4.37422072754471,0.00372710199133028,
43.651410108095));
#55536=CARTESIAN_POINT('Ctrl Pts',(-4.36348027804383,-1.18287063932153,
43.6946751959099));
#55537=CARTESIAN_POINT('Ctrl Pts',(-3.25136487986307,-3.83859580238497,
43.7908605378067));
#55538=CARTESIAN_POINT('Ctrl Pts',(1.23961889884326,-5.01651257365967,43.9399661337855));
#55539=CARTESIAN_POINT('Ctrl Pts',(4.88687423334376,-1.67943849054845,44.0987268960314));
#55540=CARTESIAN_POINT('Ctrl Pts',(4.06151299797099,3.19470899822934,44.2574876582773));
#55541=CARTESIAN_POINT('Ctrl Pts',(-0.481068993674721,5.1449612281707,44.4162484205232));
#55542=CARTESIAN_POINT('Ctrl Pts',(-3.87398394218857,2.8634067002645,44.5475559037957));
#55543=CARTESIAN_POINT('Ctrl Pts',(-4.36552146553668,0.702707227634927,
44.6259431329863));
#55544=CARTESIAN_POINT('Ctrl Pts',(-4.36487844624636,0.00044853827586927,
44.651410108095));
#55545=CARTESIAN_POINT('Ctrl Pts',(-4.36483752583336,6.45211600032447E-5,
43.848589891905));
#55546=CARTESIAN_POINT('Ctrl Pts',(-4.36474095456816,-0.733529397636361,
43.8751925962164));
#55547=CARTESIAN_POINT('Ctrl Pts',(-3.84156354313547,-2.92657717231582,
43.9547155546098));
#55548=CARTESIAN_POINT('Ctrl Pts',(-0.370823894361365,-5.15408030721166,
44.0871587670851));
#55549=CARTESIAN_POINT('Ctrl Pts',(4.12896947009338,-3.10703480650815,44.245919529331));
#55550=CARTESIAN_POINT('Ctrl Pts',(4.84980385450403,1.78366385472551,44.4046802915768));
#55551=CARTESIAN_POINT('Ctrl Pts',(1.13194961208497,5.04189887339256,44.5634410538228));
#55552=CARTESIAN_POINT('Ctrl Pts',(-3.29878256966109,3.77781872906067,44.7114109205989));
#55553=CARTESIAN_POINT('Ctrl Pts',(-4.36263242638615,1.15219838236422,44.8064605332929));
#55554=CARTESIAN_POINT('Ctrl Pts',(-4.37328422903404,-0.00388840045026397,
44.848589891905));
#55555=CARTESIAN_POINT('Origin',(0.,0.,24.1514101080949));
#55556=CARTESIAN_POINT('',(-4.37685426135052,-0.00279837449763291,42.651410108095));
#55557=CARTESIAN_POINT('',(-4.37352103895722,0.00385464862035001,42.848589891905));
#55558=CARTESIAN_POINT('',(-4.372,3.82579154166093E-12,24.1514101080949));
#55559=CARTESIAN_POINT('Ctrl Pts',(-4.37685426135052,-0.00279837449763325,
42.651410108095));
#55560=CARTESIAN_POINT('Ctrl Pts',(-4.37811047462212,-0.171387646022154,
42.6575667506695));
#55561=CARTESIAN_POINT('Ctrl Pts',(-4.29273874071207,-1.78782473877565,
42.7166436473259));
#55562=CARTESIAN_POINT('Ctrl Pts',(-2.28119196804685,-4.63661693705371,
42.8286407980642));
#55563=CARTESIAN_POINT('Ctrl Pts',(2.65807838191241,-4.43132855153674,42.9874015603103));
#55564=CARTESIAN_POINT('Ctrl Pts',(5.1645942046841,-0.170352918960309,43.146162322556));
#55565=CARTESIAN_POINT('Ctrl Pts',(2.94431565674484,4.24653490854626,43.304923084802));
#55566=CARTESIAN_POINT('Ctrl Pts',(-1.97069051554003,4.77686427565358,43.4636838470478));
#55567=CARTESIAN_POINT('Ctrl Pts',(-4.23415771881522,1.98216556151801,43.5791795214788));
#55568=CARTESIAN_POINT('Ctrl Pts',(-4.37661759834636,0.26853179933828,43.6417549418279));
#55569=CARTESIAN_POINT('Ctrl Pts',(-4.37422072754471,0.00372710199133028,
43.651410108095));
#55570=CARTESIAN_POINT('Ctrl Pts',(-4.37352103895722,0.00385464862035015,
42.848589891905));
#55571=CARTESIAN_POINT('Ctrl Pts',(-4.36282818723577,-1.15989502481933,
42.891004405058));
#55572=CARTESIAN_POINT('Ctrl Pts',(-3.28698059005484,-3.79310505340026,
42.9863391722929));
#55573=CARTESIAN_POINT('Ctrl Pts',(1.15903352033341,-5.0357417996319,43.1345941936098));
#55574=CARTESIAN_POINT('Ctrl Pts',(4.85932100888344,-1.75757034181863,43.2933549558556));
#55575=CARTESIAN_POINT('Ctrl Pts',(4.11220948021047,3.12918317851219,43.4521157181016));
#55576=CARTESIAN_POINT('Ctrl Pts',(-0.398521773825228,5.15201267172389,
43.6108764803474));
#55577=CARTESIAN_POINT('Ctrl Pts',(-3.84979170382512,2.91072243457703,43.7430345382819));
#55578=CARTESIAN_POINT('Ctrl Pts',(-4.36493306195062,0.725795042513237,
43.8222723421345));
#55579=CARTESIAN_POINT('Ctrl Pts',(-4.36483752583336,6.45211600032447E-5,
43.848589891905));
#55580=CARTESIAN_POINT('Origin',(0.,0.,24.1514101080949));
#55581=CARTESIAN_POINT('',(-4.36567955402809,-0.00194869704108157,41.651410108095));
#55582=CARTESIAN_POINT('',(-4.37739485101806,-0.00248321819134589,41.848589891905));
#55583=CARTESIAN_POINT('',(-4.372,3.82579154166093E-12,24.1514101080949));
#55584=CARTESIAN_POINT('Ctrl Pts',(-4.3656795540281,-0.00194869704108112,
41.651410108095));
#55585=CARTESIAN_POINT('Ctrl Pts',(-4.36811474531132,-0.607457052316279,
41.673378559511));
#55586=CARTESIAN_POINT('Ctrl Pts',(-3.96805804018506,-2.66850978845469,
41.748267265009));
#55587=CARTESIAN_POINT('Ctrl Pts',(-0.819065114488867,-5.10207661195736,
41.8760762245889));
#55588=CARTESIAN_POINT('Ctrl Pts',(3.8421604015636,-3.45540979692878,42.0348369868349));
#55589=CARTESIAN_POINT('Ctrl Pts',(4.98692335778749,1.35375361111553,42.1935977490807));
#55590=CARTESIAN_POINT('Ctrl Pts',(1.56750172940691,4.92392036332446,42.3523585113267));
#55591=CARTESIAN_POINT('Ctrl Pts',(-3.09830846639719,4.02387607629251,42.504962630998));
#55592=CARTESIAN_POINT('Ctrl Pts',(-4.36731252351321,1.27774424309386,42.6046464965875));
#55593=CARTESIAN_POINT('Ctrl Pts',(-4.37685426135052,-0.00279837449763325,
42.651410108095));
#55594=CARTESIAN_POINT('Ctrl Pts',(-4.37739485101806,-0.00248321819134518,
41.8485898919051));
#55595=CARTESIAN_POINT('Ctrl Pts',(-4.37838119777137,-0.1477338083412,41.8538959598176));
#55596=CARTESIAN_POINT('Ctrl Pts',(-4.30592187837124,-1.74065025431473,
41.9121222818121));
#55597=CARTESIAN_POINT('Ctrl Pts',(-2.35523429540729,-4.59944840035779,
42.0232688578885));
#55598=CARTESIAN_POINT('Ctrl Pts',(2.58669254300161,-4.47337410259821,42.1820296201345));
#55599=CARTESIAN_POINT('Ctrl Pts',(5.16119935450289,-0.253131185149624,
42.3407903823802));
#55600=CARTESIAN_POINT('Ctrl Pts',(3.01201886587614,4.19878512494061,42.4995511446263));
#55601=CARTESIAN_POINT('Ctrl Pts',(-1.89385329211466,4.80784503512363,42.6583119068721));
#55602=CARTESIAN_POINT('Ctrl Pts',(-4.21883224032928,2.02948215439444,42.774658155965));
#55603=CARTESIAN_POINT('Ctrl Pts',(-4.37616957413132,0.292106279171763,
42.838084150976));
#55604=CARTESIAN_POINT('Ctrl Pts',(-4.37352103895722,0.00385464862035015,
42.848589891905));
#55605=CARTESIAN_POINT('Origin',(0.,0.,24.1514101080949));
#55606=CARTESIAN_POINT('',(-4.36973282931957,0.00384403733829788,40.651410108095));
#55607=CARTESIAN_POINT('',(-4.36602112377814,-0.00227682230535847,40.848589891905));
#55608=CARTESIAN_POINT('',(-4.372,3.82579154166093E-12,24.1514101080949));
#55609=CARTESIAN_POINT('Ctrl Pts',(-4.36973282931958,0.00384403733829777,
40.651410108095));
#55610=CARTESIAN_POINT('Ctrl Pts',(-4.36094828703741,-1.03504959539527,
40.6891903683526));
#55611=CARTESIAN_POINT('Ctrl Pts',(-3.47031004267523,-3.54269738683393,
40.7798908826921));
#55612=CARTESIAN_POINT('Ctrl Pts',(0.715283237582617,-5.11765799033974,
40.9235116511136));
#55613=CARTESIAN_POINT('Ctrl Pts',(4.6874579011302,-2.17480846080452,41.0822724133595));
#55614=CARTESIAN_POINT('Ctrl Pts',(4.36952791329752,2.75849220244841,41.2410331756054));
#55615=CARTESIAN_POINT('Ctrl Pts',(0.052472510246957,5.16713654277911,41.3997939378513));
#55616=CARTESIAN_POINT('Ctrl Pts',(-3.70859131189293,3.16775466245737,41.5365862486812));
#55617=CARTESIAN_POINT('Ctrl Pts',(-4.36224856298441,0.851164468294318,
41.620458305429));
#55618=CARTESIAN_POINT('Ctrl Pts',(-4.3656795540281,-0.00194869704108112,
41.651410108095));
#55619=CARTESIAN_POINT('Ctrl Pts',(-4.36602112377814,-0.00227682230535861,
40.848589891905));
#55620=CARTESIAN_POINT('Ctrl Pts',(-4.36876880712171,-0.584227201261346,
40.8697077686591));
#55621=CARTESIAN_POINT('Ctrl Pts',(-3.98963601281,-2.62107929020566,40.9437458994952));
#55622=CARTESIAN_POINT('Ctrl Pts',(-0.90075771530386,-5.08828946819429,
41.0707042844132));
#55623=CARTESIAN_POINT('Ctrl Pts',(3.78626858625262,-3.51656428443629,41.2294650466591));
#55624=CARTESIAN_POINT('Ctrl Pts',(5.00798622459088,1.27362794729248,41.3882258089049));
#55625=CARTESIAN_POINT('Ctrl Pts',(1.64624189925253,4.89815697818699,41.5469865711509));
#55626=CARTESIAN_POINT('Ctrl Pts',(-3.0594815075565,4.0684328488748,41.7004412654842));
#55627=CARTESIAN_POINT('Ctrl Pts',(-4.36854383389695,1.30092803749072,41.8009757057356));
#55628=CARTESIAN_POINT('Ctrl Pts',(-4.37739485101806,-0.00248321819134518,
41.8485898919051));
#55629=CARTESIAN_POINT('Origin',(0.,0.,24.1514101080949));
#55630=CARTESIAN_POINT('',(-4.37914188721017,-0.000342719191574727,39.651410108095));
#55631=CARTESIAN_POINT('',(-4.36909141260198,0.00371732487008336,39.848589891905));
#55632=CARTESIAN_POINT('',(-4.372,3.82579154166093E-12,24.1514101080949));
#55633=CARTESIAN_POINT('Ctrl Pts',(-4.37914188721017,-0.000342719191574457,
39.651410108095));
#55634=CARTESIAN_POINT('Ctrl Pts',(-4.37916257714185,-0.0187137896541573,
39.6520819231122));
#55635=CARTESIAN_POINT('Ctrl Pts',(-4.37073789868075,-1.48419245149001,
39.7056739922113));
#55636=CARTESIAN_POINT('Ctrl Pts',(-2.74752162183386,-4.3764344338297,39.8121863153924));
#55637=CARTESIAN_POINT('Ctrl Pts',(2.18656111288008,-4.68198717594309,39.9709470776383));
#55638=CARTESIAN_POINT('Ctrl Pts',(5.11943632770732,-0.702442241472902,
40.1297078398842));
#55639=CARTESIAN_POINT('Ctrl Pts',(3.36684704019806,3.9199992887709,40.2884686021301));
#55640=CARTESIAN_POINT('Ctrl Pts',(-1.46718350018236,4.95473773199425,40.4472293643759));
#55641=CARTESIAN_POINT('Ctrl Pts',(-4.12759825135317,2.28764036559584,40.5682098663642));
#55642=CARTESIAN_POINT('Ctrl Pts',(-4.37325313105903,0.420168410874277,
40.6362701142706));
#55643=CARTESIAN_POINT('Ctrl Pts',(-4.36973282931958,0.00384403733829777,
40.651410108095));
#55644=CARTESIAN_POINT('Ctrl Pts',(-4.36909141260198,0.0037173248700835,
39.848589891905));
#55645=CARTESIAN_POINT('Ctrl Pts',(-4.36087746473157,-1.01216450930882,
39.8855195775007));
#55646=CARTESIAN_POINT('Ctrl Pts',(-3.50202565789313,-3.49632888214117,
39.9753695171783));
#55647=CARTESIAN_POINT('Ctrl Pts',(0.6331436514814,-5.12846792818335,40.1181397109379));
#55648=CARTESIAN_POINT('Ctrl Pts',(4.65198839971611,-2.2496795555641,40.2769004731838));
#55649=CARTESIAN_POINT('Ctrl Pts',(4.41319126769477,2.68808426366416,40.4356612354296));
#55650=CARTESIAN_POINT('Ctrl Pts',(0.135306684796697,5.16563125618407,40.5944219976755));
#55651=CARTESIAN_POINT('Ctrl Pts',(-3.68091103301737,3.21474907678104,40.7320648831673));
#55652=CARTESIAN_POINT('Ctrl Pts',(-4.36188326164895,0.874108893605594,
40.8167875145772));
#55653=CARTESIAN_POINT('Ctrl Pts',(-4.36602112377814,-0.00227682230535861,
40.848589891905));
#55654=CARTESIAN_POINT('Origin',(0.,0.,24.1514101080949));
#55655=CARTESIAN_POINT('',(-4.36873305544013,-0.00362749675167218,38.651410108095));
#55656=CARTESIAN_POINT('',(-4.37917310725098,9.13219796030052E-5,38.848589891905));
#55657=CARTESIAN_POINT('',(-4.372,3.82579154166093E-12,24.1514101080949));
#55658=CARTESIAN_POINT('Ctrl Pts',(-4.36873305544013,-0.00362749675167234,
38.651410108095));
#55659=CARTESIAN_POINT('Ctrl Pts',(-4.37228988643661,-0.457161961038693,
38.6678937319537));
#55660=CARTESIAN_POINT('Ctrl Pts',(-4.0986296928328,-2.36257101965516,38.7372976098944));
#55661=CARTESIAN_POINT('Ctrl Pts',(-1.34123858177823,-4.99030384674165,
38.8596217419171));
#55662=CARTESIAN_POINT('Ctrl Pts',(3.46503780867414,-3.83347967263602,39.0183825041629));
#55663=CARTESIAN_POINT('Ctrl Pts',(5.10000575566994,0.831862193027325,39.1771432664089));
#55664=CARTESIAN_POINT('Ctrl Pts',(2.06729265337245,4.73585837007054,39.3359040286547));
#55665=CARTESIAN_POINT('Ctrl Pts',(-2.83663011433148,4.30727362250648,39.4939929758834));
#55666=CARTESIAN_POINT('Ctrl Pts',(-4.37753278856417,1.42841330898948,39.5991616690302));
#55667=CARTESIAN_POINT('Ctrl Pts',(-4.37914188721017,-0.000342719191574457,
39.651410108095));
#55668=CARTESIAN_POINT('Ctrl Pts',(-4.37917310725098,9.13219796029981E-5,
38.848589891905));
#55669=CARTESIAN_POINT('Ctrl Pts',(-4.37872965626048,-1.44211984317019,
38.9013313863422));
#55670=CARTESIAN_POINT('Ctrl Pts',(-2.81178331229755,-4.33225607926283,
39.0069931348614));
#55671=CARTESIAN_POINT('Ctrl Pts',(2.11121724282438,-4.71644102342194,39.1655751374625));
#55672=CARTESIAN_POINT('Ctrl Pts',(5.10751668218689,-0.784428145210908,
39.3243358997084));
#55673=CARTESIAN_POINT('Ctrl Pts',(3.42926084288352,3.86551733216684,39.4830966619543));
#55674=CARTESIAN_POINT('Ctrl Pts',(-1.38755926796319,4.97762327338117,39.6418574242002));
#55675=CARTESIAN_POINT('Ctrl Pts',(-4.1093944849834,2.33507192947434,39.7636885008504));
#55676=CARTESIAN_POINT('Ctrl Pts',(-4.37264805528242,0.443594561337992,
39.8325993234187));
#55677=CARTESIAN_POINT('Ctrl Pts',(-4.36909141260198,0.0037173248700835,
39.848589891905));
#55678=CARTESIAN_POINT('Origin',(0.,0.,24.1514101080949));
#55679=CARTESIAN_POINT('',(-4.36624352627694,0.00245771687439172,37.651410108095));
#55680=CARTESIAN_POINT('',(-4.36935764006,-0.00377501215838794,37.848589891905));
#55681=CARTESIAN_POINT('',(-4.372,3.82579154166093E-12,24.1514101080949));
#55682=CARTESIAN_POINT('Ctrl Pts',(-4.36624352627694,0.00245771687439181,
37.651410108095));
#55683=CARTESIAN_POINT('Ctrl Pts',(-4.36169382655995,-0.887401680305794,
37.6837055407953));
#55684=CARTESIAN_POINT('Ctrl Pts',(-3.66460952904662,-3.24195865307006,
37.7689212275775));
#55685=CARTESIAN_POINT('Ctrl Pts',(0.183308877707052,-5.16415058566349,
37.9070571684418));
#55686=CARTESIAN_POINT('Ctrl Pts',(4.43798296793759,-2.64695307709652,38.0658179306876));
#55687=CARTESIAN_POINT('Ctrl Pts',(4.63087948595682,2.29281673986369,38.2245786929335));
#55688=CARTESIAN_POINT('Ctrl Pts',(0.585453646372677,5.13413064150142,38.3833394551794));
#55689=CARTESIAN_POINT('Ctrl Pts',(-3.52014057613125,3.46939996827985,38.5256165935665));
#55690=CARTESIAN_POINT('Ctrl Pts',(-4.36087077121817,0.99889887186349,38.6149734778717));
#55691=CARTESIAN_POINT('Ctrl Pts',(-4.36873305544013,-0.00362749675167234,
38.651410108095));
#55692=CARTESIAN_POINT('Ctrl Pts',(-4.36935764006,-0.00377501215838787,
37.848589891905));
#55693=CARTESIAN_POINT('Ctrl Pts',(-4.37290446571934,-0.43375111631892,
37.8642229411018));
#55694=CARTESIAN_POINT('Ctrl Pts',(-4.11710236903147,-2.31513392579321,
37.9327762443806));
#55695=CARTESIAN_POINT('Ctrl Pts',(-1.42107210669624,-4.96815944202542,
38.0542498017413));
#55696=CARTESIAN_POINT('Ctrl Pts',(3.40313314014881,-3.88853944357485,38.2130105639872));
#55697=CARTESIAN_POINT('Ctrl Pts',(5.11268698707437,0.749990630619295,38.3717713262331));
#55698=CARTESIAN_POINT('Ctrl Pts',(2.14295353437204,4.70210637090854,38.5305320884789));
#55699=CARTESIAN_POINT('Ctrl Pts',(-2.78807645035559,4.35071073283309,38.6892928507248));
#55700=CARTESIAN_POINT('Ctrl Pts',(-4.37695363416618,1.45696557727882,38.7953121185335));
#55701=CARTESIAN_POINT('Ctrl Pts',(-4.37917461026378,0.0049794875180062,
38.8484111322603));
#55702=CARTESIAN_POINT('Ctrl Pts',(-4.37917310725098,9.13219796029981E-5,
38.848589891905));
#55703=CARTESIAN_POINT('Origin',(0.,0.,24.1514101080949));
#55704=CARTESIAN_POINT('',(-4.37768323182342,0.00228667983145002,36.651410108095));
#55705=CARTESIAN_POINT('',(-4.36587095680509,0.00214125659340675,36.848589891905));
#55706=CARTESIAN_POINT('',(-4.372,3.82579154166093E-12,24.1514101080949));
#55707=CARTESIAN_POINT('Ctrl Pts',(-4.37768323182342,0.00228667983144982,
36.651410108095));
#55708=CARTESIAN_POINT('Ctrl Pts',(-4.36931436006514,-1.31439298482965,
36.6995173496368));
#55709=CARTESIAN_POINT('Ctrl Pts',(-3.03668215072675,-4.09416581339981,
36.8005448452606));
#55710=CARTESIAN_POINT('Ctrl Pts',(1.69169298020808,-4.88264562268956,36.9544925949664));
#55711=CARTESIAN_POINT('Ctrl Pts',(5.01960663803976,-1.22702999775959,37.1132533572123));
#55712=CARTESIAN_POINT('Ctrl Pts',(3.75342297485632,3.55160096123927,37.2720141194582));
#55713=CARTESIAN_POINT('Ctrl Pts',(-0.94800804471325,5.07969823544803,37.430774881704));
#55714=CARTESIAN_POINT('Ctrl Pts',(-4.00191688963235,2.59358013793749,37.5572402112497));
#55715=CARTESIAN_POINT('Ctrl Pts',(-4.36914909948521,0.570748326013101,
37.6307852867133));
#55716=CARTESIAN_POINT('Ctrl Pts',(-4.36624352627694,0.00245771687439181,
37.651410108095));
#55717=CARTESIAN_POINT('Ctrl Pts',(-4.36587095680509,0.00214125659340626,
36.848589891905));
#55718=CARTESIAN_POINT('Ctrl Pts',(-4.36203103509102,-0.864466812036311,
36.8800347499434));
#55719=CARTESIAN_POINT('Ctrl Pts',(-3.6926137083843,-3.19500429871341,36.9643998620637));
#55720=CARTESIAN_POINT('Ctrl Pts',(0.100492274349119,-5.16642579319712,
37.101685228266));
#55721=CARTESIAN_POINT('Ctrl Pts',(4.39497597774354,-2.71776384714963,37.2604459905118));
#55722=CARTESIAN_POINT('Ctrl Pts',(4.66704342001788,2.21827858698683,37.4192067527577));
#55723=CARTESIAN_POINT('Ctrl Pts',(0.66769016759438,5.12408470011126,37.5779675150036));
#55724=CARTESIAN_POINT('Ctrl Pts',(-3.48876670478196,3.51583248140767,37.7210952280527));
#55725=CARTESIAN_POINT('Ctrl Pts',(-4.36089792030941,1.02178352666142,37.8113026870198));
#55726=CARTESIAN_POINT('Ctrl Pts',(-4.36935764006,-0.00377501215838787,
37.848589891905));
#55727=CARTESIAN_POINT('Origin',(0.,0.,24.1514101080949));
#55728=CARTESIAN_POINT('',(-4.37311107145795,-0.00391014173522758,35.651410108095));
#55729=CARTESIAN_POINT('',(-4.3771739373938,0.00261949572194539,35.848589891905));
#55730=CARTESIAN_POINT('',(-4.372,3.82579154166093E-12,24.1514101080949));
#55731=CARTESIAN_POINT('Ctrl Pts',(-4.37311107145795,-0.00391014173522778,
35.651410108095));
#55732=CARTESIAN_POINT('Ctrl Pts',(-4.3758959220056,-0.305762745961795,
35.6624089043964));
#55733=CARTESIAN_POINT('Ctrl Pts',(-4.20975035875682,-2.05692106559916,
35.7263279547798));
#55734=CARTESIAN_POINT('Ctrl Pts',(-1.84908860800444,-4.8252383087059,35.8431672592452));
#55735=CARTESIAN_POINT('Ctrl Pts',(3.05091116183891,-4.17061080641931,36.0019280214911));
#55736=CARTESIAN_POINT('Ctrl Pts',(5.15862384507246,0.301087098868051,36.1606887837369));
#55737=CARTESIAN_POINT('Ctrl Pts',(2.54500641307862,4.49722089444621,36.3194495459828));
#55738=CARTESIAN_POINT('Ctrl Pts',(-2.39787862639785,4.5773607580263,36.4782103082287));
#55739=CARTESIAN_POINT('Ctrl Pts',(-4.31337783157312,1.71331867151843,36.5888638289328));
#55740=CARTESIAN_POINT('Ctrl Pts',(-4.37852051709334,0.134017278681583,
36.6465970955549));
#55741=CARTESIAN_POINT('Ctrl Pts',(-4.37768323182342,0.00228667983144982,
36.651410108095));
#55742=CARTESIAN_POINT('Ctrl Pts',(-4.3771739373938,0.00261949572194524,
35.848589891905));
#55743=CARTESIAN_POINT('Ctrl Pts',(-4.36801132265503,-1.29117660831409,
35.8958465587849));
#55744=CARTESIAN_POINT('Ctrl Pts',(-3.07587918570516,-4.04972946385307,
35.9960234797468));
#55745=CARTESIAN_POINT('Ctrl Pts',(1.61319569609569,-4.90913982484862,36.1491206547906));
#55746=CARTESIAN_POINT('Ctrl Pts',(4.99928949022287,-1.30734798992603,36.3078814170365));
#55747=CARTESIAN_POINT('Ctrl Pts',(3.80988083761225,3.49096865884117,36.4666421792824));
#55748=CARTESIAN_POINT('Ctrl Pts',(-0.866447131906533,5.09424415801081,
36.6254029415283));
#55749=CARTESIAN_POINT('Ctrl Pts',(-3.9806269029927,2.64101706972627,36.7527188457358));
#55750=CARTESIAN_POINT('Ctrl Pts',(-4.36849344724489,0.59399482660225,36.8271144958614));
#55751=CARTESIAN_POINT('Ctrl Pts',(-4.36587095680509,0.00214125659340626,
36.848589891905));
#55752=CARTESIAN_POINT('Origin',(0.,0.,24.1514101080949));
#55753=CARTESIAN_POINT('',(-4.36484181559087,0.000158569877717519,34.651410108095));
#55754=CARTESIAN_POINT('',(-4.37381658707025,-0.00380592486605935,34.848589891905));
#55755=CARTESIAN_POINT('',(-4.372,3.82579154166093E-12,24.1514101080949));
#55756=CARTESIAN_POINT('Ctrl Pts',(-4.36484181559087,0.000158569877717965,
34.651410108095));
#55757=CARTESIAN_POINT('Ctrl Pts',(-4.36460260997581,-0.739166555623858,
34.6782207132379));
#55758=CARTESIAN_POINT('Ctrl Pts',(-3.83552704168218,-2.93813387262851,
34.7579515724629));
#55759=CARTESIAN_POINT('Ctrl Pts',(-0.350623086089188,-5.15549385292585,
34.8906026857698));
#55760=CARTESIAN_POINT('Ctrl Pts',(4.14111364246891,-3.09083018236409,35.0493634480157));
#55761=CARTESIAN_POINT('Ctrl Pts',(4.84277667347619,1.80265568173448,35.2081242102616));
#55762=CARTESIAN_POINT('Ctrl Pts',(1.11218256837853,5.0462960030749,35.3668849725075));
#55763=CARTESIAN_POINT('Ctrl Pts',(-3.30734354987895,3.76666274637145,35.5146469384519));
#55764=CARTESIAN_POINT('Ctrl Pts',(-4.36249672862818,1.14658859078299,35.6094886503144));
#55765=CARTESIAN_POINT('Ctrl Pts',(-4.37311107145795,-0.00391014173522778,
35.651410108095));
#55766=CARTESIAN_POINT('Ctrl Pts',(-4.37381658707025,-0.00380592486605963,
34.848589891905));
#55767=CARTESIAN_POINT('Ctrl Pts',(-4.37636167316891,-0.282199643018631,
34.8587381135445));
#55768=CARTESIAN_POINT('Ctrl Pts',(-4.22532647145104,-2.00959079533273,
34.921806589266));
#55769=CARTESIAN_POINT('Ctrl Pts',(-1.92621049372714,-4.7949731289833,35.0377953190694));
#55770=CARTESIAN_POINT('Ctrl Pts',(2.98365473640471,-4.21898786295316,35.1965560813153));
#55771=CARTESIAN_POINT('Ctrl Pts',(5.16278801485838,0.21834396591395,35.3553168435612));
#55772=CARTESIAN_POINT('Ctrl Pts',(2.61678000270041,4.45584072777334,35.514077605807));
#55773=CARTESIAN_POINT('Ctrl Pts',(-2.32418499851494,4.61521595014736,35.672838368053));
#55774=CARTESIAN_POINT('Ctrl Pts',(-4.30043031041834,1.76047520998047,35.7843424634189));
#55775=CARTESIAN_POINT('Ctrl Pts',(-4.37827205266511,0.157677555053939,
35.842926304703));
#55776=CARTESIAN_POINT('Ctrl Pts',(-4.3771739373938,0.00261949572194524,
35.848589891905));
#55777=CARTESIAN_POINT('Origin',(0.,0.,24.1514101080949));
#55778=CARTESIAN_POINT('',(-4.37369305382679,0.00382718076316987,33.651410108095));
#55779=CARTESIAN_POINT('',(-4.36484727915486,-0.000226203520788115,33.848589891905));
#55780=CARTESIAN_POINT('',(-4.372,3.82579154166093E-12,24.1514101080949));
#55781=CARTESIAN_POINT('Ctrl Pts',(-4.37369305382679,0.00382718076316957,
33.651410108095));
#55782=CARTESIAN_POINT('Ctrl Pts',(-4.36297801900768,-1.16550827733193,
33.6940325220795));
#55783=CARTESIAN_POINT('Ctrl Pts',(-3.27833228748252,-3.80423885928109,
33.789575190146));
#55784=CARTESIAN_POINT('Ctrl Pts',(1.17875881138994,-5.0311610072254,33.9380381122944));
#55785=CARTESIAN_POINT('Ctrl Pts',(4.86617124330449,-1.73851397661661,34.0967988745404));
#55786=CARTESIAN_POINT('Ctrl Pts',(4.09991511421076,3.14527414899259,34.2555596367862));
#55787=CARTESIAN_POINT('Ctrl Pts',(-0.418708560946466,5.15041129979394,
34.4143203990322));
#55788=CARTESIAN_POINT('Ctrl Pts',(-3.85575329743435,2.89916044399897,34.5462705561351));
#55789=CARTESIAN_POINT('Ctrl Pts',(-4.36507476723817,0.720154234863851,
34.625300459156));
#55790=CARTESIAN_POINT('Ctrl Pts',(-4.36484181559087,0.000158569877717965,
34.651410108095));
#55791=CARTESIAN_POINT('Ctrl Pts',(-4.36484727915486,-0.000226203520787838,
33.848589891905));
#55792=CARTESIAN_POINT('Ctrl Pts',(-4.36517770844991,-0.716093813355663,
33.8745499223861));
#55793=CARTESIAN_POINT('Ctrl Pts',(-3.86002428520416,-2.89083849180258,
33.9534302069491));
#55794=CARTESIAN_POINT('Ctrl Pts',(-0.433232286323001,-5.1492100326073,
34.085230745594));
#55795=CARTESIAN_POINT('Ctrl Pts',(4.0910284465022,-3.15682442079478,34.24399150784));
#55796=CARTESIAN_POINT('Ctrl Pts',(4.87105498299758,1.72478332738662,34.4027522700858));
#55797=CARTESIAN_POINT('Ctrl Pts',(1.1929432107418,5.02781669015105,34.5615130323318));
#55798=CARTESIAN_POINT('Ctrl Pts',(-3.27208568972255,3.81224566198089,34.7101255729381));
#55799=CARTESIAN_POINT('Ctrl Pts',(-4.36308973176021,1.16954893154173,34.8058178594626));
#55800=CARTESIAN_POINT('Ctrl Pts',(-4.37381658707025,-0.00380592486605963,
34.848589891905));
#55801=CARTESIAN_POINT('Origin',(0.,0.,24.1514101080949));
#55802=CARTESIAN_POINT('',(-4.37726747931578,-0.00256312102853162,32.651410108095));
#55803=CARTESIAN_POINT('',(-4.37298639645094,0.00392429018828133,32.848589891905));
#55804=CARTESIAN_POINT('',(-4.372,3.82579154166093E-12,24.1514101080949));
#55805=CARTESIAN_POINT('Ctrl Pts',(-4.37726747931578,-0.0025631210285324,
32.651410108095));
#55806=CARTESIAN_POINT('Ctrl Pts',(-4.37831848753371,-0.153516427525766,
32.6569240768391));
#55807=CARTESIAN_POINT('Ctrl Pts',(-4.30273715326605,-1.7521779604483,32.7153582996652));
#55808=CARTESIAN_POINT('Ctrl Pts',(-2.33719172860392,-4.60864277632799,
32.8267127765732));
#55809=CARTESIAN_POINT('Ctrl Pts',(2.60420302889879,-4.4632028858578,32.9854735388192));
#55810=CARTESIAN_POINT('Ctrl Pts',(5.16215162793603,-0.232903383943239,
33.144234301065));
#55811=CARTESIAN_POINT('Ctrl Pts',(2.99554137711165,4.21055640908263,33.302995063311));
#55812=CARTESIAN_POINT('Ctrl Pts',(-1.91267984204806,4.80038636339596,33.4617558255568));
#55813=CARTESIAN_POINT('Ctrl Pts',(-4.22261792613804,2.01791460332865,33.5778941738182));
#55814=CARTESIAN_POINT('Ctrl Pts',(-4.37628187282812,0.286345894322504,
33.6411122679975));
#55815=CARTESIAN_POINT('Ctrl Pts',(-4.37369305382679,0.00382718076316957,
33.651410108095));
#55816=CARTESIAN_POINT('Ctrl Pts',(-4.37298639645094,0.00392429018828126,
32.848589891905));
#55817=CARTESIAN_POINT('Ctrl Pts',(-4.36240284050621,-1.14255230782506,
32.8903617312276));
#55818=CARTESIAN_POINT('Ctrl Pts',(-3.31348194711132,-3.75862865123049,
32.9850538246322));
#55819=CARTESIAN_POINT('Ctrl Pts',(1.09794640645064,-5.04941262548215,33.1326661721187));
#55820=CARTESIAN_POINT('Ctrl Pts',(4.83767356537879,-1.81630632015957,33.2914269343646));
#55821=CARTESIAN_POINT('Ctrl Pts',(4.14981410860918,3.07913900917197,33.4501876966104));
#55822=CARTESIAN_POINT('Ctrl Pts',(-0.336081978081961,5.15646226378366,
33.6089484588564));
#55823=CARTESIAN_POINT('Ctrl Pts',(-3.83116330074657,2.94644944182165,33.7417491906212));
#55824=CARTESIAN_POINT('Ctrl Pts',(-4.36450411901545,0.743222493270702,
33.8216296683041));
#55825=CARTESIAN_POINT('Ctrl Pts',(-4.36484727915486,-0.000226203520787838,
33.848589891905));
#55826=CARTESIAN_POINT('Origin',(0.,0.,24.1514101080949));
#55827=CARTESIAN_POINT('',(-4.36593258301536,-0.00219842154078257,31.651410108095));
#55828=CARTESIAN_POINT('',(-4.37776688532802,-0.00222515354369623,31.848589891905));
#55829=CARTESIAN_POINT('',(-4.372,3.82579154166093E-12,24.1514101080949));
#55830=CARTESIAN_POINT('Ctrl Pts',(-4.36593258301536,-0.00219842154078276,
31.651410108095));
#55831=CARTESIAN_POINT('Ctrl Pts',(-4.36860855649085,-0.589907775928666,
31.6727358856806));
#55832=CARTESIAN_POINT('Ctrl Pts',(-3.98440775127391,-2.63267349583233,
31.7469819173483));
#55833=CARTESIAN_POINT('Ctrl Pts',(-0.880810653343035,-5.09178023966167,
31.8741482030979));
#55834=CARTESIAN_POINT('Ctrl Pts',(3.80002027066033,-3.5016994957634,32.0329089653438));
#55835=CARTESIAN_POINT('Ctrl Pts',(5.00295656982363,1.29324358746212,32.1916697275897));
#55836=CARTESIAN_POINT('Ctrl Pts',(1.62703419898677,4.90457063680218,32.3504304898356));
#55837=CARTESIAN_POINT('Ctrl Pts',(-3.06903058869073,4.05756105615878,32.5036772833373));
#55838=CARTESIAN_POINT('Ctrl Pts',(-4.36823144777778,1.29525626325957,32.6040038227571));
#55839=CARTESIAN_POINT('Ctrl Pts',(-4.37726747931578,-0.0025631210285324,
32.651410108095));
#55840=CARTESIAN_POINT('Ctrl Pts',(-4.37776688532802,-0.00222515354369674,
31.848589891905));
#55841=CARTESIAN_POINT('Ctrl Pts',(-4.37856029699079,-0.129854311945594,
31.8532532859872));
#55842=CARTESIAN_POINT('Ctrl Pts',(-4.31561362407578,-1.70502699061033,
31.9108369341514));
#55843=CARTESIAN_POINT('Ctrl Pts',(-2.41077837014428,-4.57058003144683,
32.0213408363975));
#55844=CARTESIAN_POINT('Ctrl Pts',(2.53231309568674,-4.50438059662262,32.1801015986434));
#55845=CARTESIAN_POINT('Ctrl Pts',(5.15775426583447,-0.31563445167244,32.3388623608893));
#55846=CARTESIAN_POINT('Ctrl Pts',(3.06266118623515,4.16198998462816,32.4976231231351));
#55847=CARTESIAN_POINT('Ctrl Pts',(-1.83547296121064,4.83043405735769,32.6563838853811));
#55848=CARTESIAN_POINT('Ctrl Pts',(-4.20696559908301,2.06524898522119,32.7733728083043));
#55849=CARTESIAN_POINT('Ctrl Pts',(-4.37581102359723,0.309905468748449,
32.8374414771457));
#55850=CARTESIAN_POINT('Ctrl Pts',(-4.37298639645094,0.00392429018828126,
32.848589891905));
#55851=CARTESIAN_POINT('Origin',(0.,0.,24.1514101080949));
#55852=CARTESIAN_POINT('',(-4.36924553642194,0.00375164274966603,30.651410108095));
#55853=CARTESIAN_POINT('',(-4.36631454878401,-0.00251114173366096,30.848589891905));
#55854=CARTESIAN_POINT('',(-4.372,3.82579154166093E-12,24.1514101080949));
#55855=CARTESIAN_POINT('Ctrl Pts',(-4.36924553642194,0.00375164274966585,
30.651410108095));
#55856=CARTESIAN_POINT('Ctrl Pts',(-4.36088767272676,-1.01775802631581,
30.6885476945222));
#55857=CARTESIAN_POINT('Ctrl Pts',(-3.49432807348169,-3.50767273053874,
30.7786055350314));
#55858=CARTESIAN_POINT('Ctrl Pts',(0.653236365857992,-5.12594729451212,
30.9215836296226));
#55859=CARTESIAN_POINT('Ctrl Pts',(4.6607687206244,-2.23143190555148,31.0803443918685));
#55860=CARTESIAN_POINT('Ctrl Pts',(4.4026231771807,2.70535812338375,31.2391051541143));
#55861=CARTESIAN_POINT('Ctrl Pts',(0.115062422136807,5.16612176153803,31.3978659163603));
#55862=CARTESIAN_POINT('Ctrl Pts',(-3.68772820349694,3.20326873769824,31.5353009010205));
#55863=CARTESIAN_POINT('Ctrl Pts',(-4.36196808602404,0.868502274330174,
31.6198156315987));
#55864=CARTESIAN_POINT('Ctrl Pts',(-4.36593258301536,-0.00219842154078276,
31.651410108095));
#55865=CARTESIAN_POINT('Ctrl Pts',(-4.36631454878401,-0.0025111417336611,
30.848589891905));
#55866=CARTESIAN_POINT('Ctrl Pts',(-4.36926463444175,-0.566656242129838,
30.8690650948288));
#55867=CARTESIAN_POINT('Ctrl Pts',(-4.00561083840711,-2.58523495481153,
30.9424605518345));
#55868=CARTESIAN_POINT('Ctrl Pts',(-0.962330244988123,-5.07700449806455,
31.0687762629221));
#55869=CARTESIAN_POINT('Ctrl Pts',(3.74339174195905,-3.56217243267071,31.2275370251681));
#55870=CARTESIAN_POINT('Ctrl Pts',(5.02304726326813,1.21286865108392,31.3862977874139));
#55871=CARTESIAN_POINT('Ctrl Pts',(1.70545649826175,4.87785529780762,31.5450585496599));
#55872=CARTESIAN_POINT('Ctrl Pts',(-3.02972114369421,4.10196041210765,31.6991559178235));
#55873=CARTESIAN_POINT('Ctrl Pts',(-4.36955665156738,1.31848296597982,31.8003330319052));
#55874=CARTESIAN_POINT('Ctrl Pts',(-4.37776688532802,-0.00222515354369674,
31.848589891905));
#55875=CARTESIAN_POINT('Origin',(0.,0.,24.1514101080949));
#55876=CARTESIAN_POINT('',(-4.37917542201394,-1.48878467067329E-5,29.651410108095));
#55877=CARTESIAN_POINT('',(-4.36862654983539,0.00359793095617206,29.848589891905));
#55878=CARTESIAN_POINT('',(-4.372,3.82579154166093E-12,24.1514101080949));
#55879=CARTESIAN_POINT('Ctrl Pts',(-4.3791753974872,-1.48877958181532E-5,
29.651410108095));
#55880=CARTESIAN_POINT('Ctrl Pts',(-4.37917543773958,-0.000811749618496727,
29.6514392492818));
#55881=CARTESIAN_POINT('Ctrl Pts',(-4.37881439934298,-1.44870578249893,
29.7043886445506));
#55882=CARTESIAN_POINT('Ctrl Pts',(-2.80033535833003,-4.34283033250174,
29.8102582939013));
#55883=CARTESIAN_POINT('Ctrl Pts',(2.12968392236957,-4.70813124181331,29.9690190561473));
#55884=CARTESIAN_POINT('Ctrl Pts',(5.11055143098187,-0.764406630547101,
30.1277798183931));
#55885=CARTESIAN_POINT('Ctrl Pts',(3.41408616315334,3.87892628001712,30.286540580639));
#55886=CARTESIAN_POINT('Ctrl Pts',(-1.4070550442568,4.97214737476293,30.4453013428849));
#55887=CARTESIAN_POINT('Ctrl Pts',(-4.11388660080008,2.32347755138503,30.5669245187036));
#55888=CARTESIAN_POINT('Ctrl Pts',(-4.37279744697119,0.437871066329566,
30.6356274404402));
#55889=CARTESIAN_POINT('Ctrl Pts',(-4.36924553642194,0.00375164274966585,
30.651410108095));
#55890=CARTESIAN_POINT('Ctrl Pts',(-4.36862654983539,0.0035979309561724,
29.848589891905));
#55891=CARTESIAN_POINT('Ctrl Pts',(-4.36087365922317,-0.994873321808196,
29.8848769036703));
#55892=CARTESIAN_POINT('Ctrl Pts',(-3.52559867611562,-3.46122138486278,
29.9740841695176));
#55893=CARTESIAN_POINT('Ctrl Pts',(0.570971856938151,-5.13576141485164,
30.1162116894468));
#55894=CARTESIAN_POINT('Ctrl Pts',(4.62439484690811,-2.30586783557282,30.2749724516927));
#55895=CARTESIAN_POINT('Ctrl Pts',(4.44543041863472,2.63442642081081,30.4337332139386));
#55896=CARTESIAN_POINT('Ctrl Pts',(0.1978722839815,5.16361314708889,30.5924939761844));
#55897=CARTESIAN_POINT('Ctrl Pts',(-3.65962554388572,3.25021066517935,30.7307795355066));
#55898=CARTESIAN_POINT('Ctrl Pts',(-4.361639836624,0.891434413344724,30.8161448407468));
#55899=CARTESIAN_POINT('Ctrl Pts',(-4.36631454878401,-0.0025111417336611,
30.848589891905));
#55900=CARTESIAN_POINT('Origin',(0.,0.,24.1514101080949));
#55901=CARTESIAN_POINT('',(-4.36920210772109,-0.00374225457618444,28.651410108095));
#55902=CARTESIAN_POINT('',(-4.379125585284,0.000418740495046069,28.848589891905));
#55903=CARTESIAN_POINT('',(-4.372,3.82579154166093E-12,24.1514101080949));
#55904=CARTESIAN_POINT('Ctrl Pts',(-4.36920210772109,-0.00374225457618473,
28.651410108095));
#55905=CARTESIAN_POINT('Ctrl Pts',(-4.37275566211042,-0.439475723050513,
28.6672510581234));
#55906=CARTESIAN_POINT('Ctrl Pts',(-4.11263026215736,-2.3267277008933,28.7360122622337));
#55907=CARTESIAN_POINT('Ctrl Pts',(-1.40159165779937,-4.9736902589037,28.857693720426));
#55908=CARTESIAN_POINT('Ctrl Pts',(3.41834539873403,-3.87517318393326,29.0164544826719));
#55909=CARTESIAN_POINT('Ctrl Pts',(5.10970861334159,0.770020576487015,29.1752152449178));
#55910=CARTESIAN_POINT('Ctrl Pts',(2.12451027984608,4.71046807932676,29.3339760071637));
#55911=CARTESIAN_POINT('Ctrl Pts',(-2.80419982800075,4.33981931003669,29.4927076282227));
#55912=CARTESIAN_POINT('Ctrl Pts',(-4.37910233962271,1.44628545901738,29.5985189951998));
#55913=CARTESIAN_POINT('Ctrl Pts',(-4.3791753974872,-1.48877958181532E-5,
29.651410108095));
#55914=CARTESIAN_POINT('Ctrl Pts',(-4.379125585284,0.000418740495045835,
28.848589891905));
#55915=CARTESIAN_POINT('Ctrl Pts',(-4.37717920749743,-1.42426027511931,
28.9006887125119));
#55916=CARTESIAN_POINT('Ctrl Pts',(-2.84412638479826,-4.2996753084771,29.0057077872007));
#55917=CARTESIAN_POINT('Ctrl Pts',(2.05392820456428,-4.74166985111631,29.1636471159715));
#55918=CARTESIAN_POINT('Ctrl Pts',(5.09763950196961,-0.846242130327758,
29.3224078782173));
#55919=CARTESIAN_POINT('Ctrl Pts',(3.47583539931961,3.82369225364773,29.4811686404633));
#55920=CARTESIAN_POINT('Ctrl Pts',(-1.32715942194175,4.9940666821606,29.6399294027091));
#55921=CARTESIAN_POINT('Ctrl Pts',(-4.09533214146315,2.37091623060187,29.7624031531897));
#55922=CARTESIAN_POINT('Ctrl Pts',(-4.37218032023241,0.461277235079317,
29.8319566495884));
#55923=CARTESIAN_POINT('Ctrl Pts',(-4.36862654983539,0.0035979309561724,
29.848589891905));
#55924=CARTESIAN_POINT('Origin',(0.,0.,24.1514101080949));
#55925=CARTESIAN_POINT('',(-4.36594998909341,0.00221597220681413,27.651410108095));
#55926=CARTESIAN_POINT('',(-4.36984836444492,-0.00386263586949487,27.848589891905));
#55927=CARTESIAN_POINT('',(-4.372,3.82579154166093E-12,24.1514101080949));
#55928=CARTESIAN_POINT('Ctrl Pts',(-4.36594998909341,0.00221597220681394,
27.651410108095));
#55929=CARTESIAN_POINT('Ctrl Pts',(-4.36193991209169,-0.870076739562532,
27.6830628669649));
#55930=CARTESIAN_POINT('Ctrl Pts',(-3.68583197785541,-3.20648009630763,
27.7676358799168));
#55931=CARTESIAN_POINT('Ctrl Pts',(0.12074539761077,-5.16599709979471,27.9051291469506));
#55932=CARTESIAN_POINT('Ctrl Pts',(4.40558866999103,-2.70051724468854,28.0638899091966));
#55933=CARTESIAN_POINT('Ctrl Pts',(4.65831652566081,2.23654953809766,28.2226506714425));
#55934=CARTESIAN_POINT('Ctrl Pts',(0.647603546994949,5.12666253671564,28.3814114336883));
#55935=CARTESIAN_POINT('Ctrl Pts',(-3.49648913171247,3.50449301705117,28.5243312459059));
#55936=CARTESIAN_POINT('Ctrl Pts',(-4.36088421495349,1.0161898665986,28.6143308040414));
#55937=CARTESIAN_POINT('Ctrl Pts',(-4.36920210772109,-0.00374225457618473,
28.651410108095));
#55938=CARTESIAN_POINT('Ctrl Pts',(-4.36984836444492,-0.00386263586949508,
27.848589891905));
#55939=CARTESIAN_POINT('Ctrl Pts',(-4.37335795381477,-0.41604489030568,
27.8635802672715));
#55940=CARTESIAN_POINT('Ctrl Pts',(-4.13075387899131,-2.27929715120676,
27.9314908967199));
#55941=CARTESIAN_POINT('Ctrl Pts',(-1.48115027726835,-4.95058115072351,
28.0523217802503));
#55942=CARTESIAN_POINT('Ctrl Pts',(3.35577787359124,-3.92947861571792,28.2110825424961));
#55943=CARTESIAN_POINT('Ctrl Pts',(5.12139735341277,0.688001195909337,28.369843304742));
#55944=CARTESIAN_POINT('Ctrl Pts',(2.1997566305386,4.67580212267651,28.5286040669879));
#55945=CARTESIAN_POINT('Ctrl Pts',(-2.7351680780718,4.38416569184913,28.6873648292338));
#55946=CARTESIAN_POINT('Ctrl Pts',(-4.36882639464741,1.49245678983841,28.7940267708728));
#55947=CARTESIAN_POINT('Ctrl Pts',(-4.37915627350017,0.0228814185571984,
28.8477684584299));
#55948=CARTESIAN_POINT('Ctrl Pts',(-4.379125585284,0.000418740495045835,
28.848589891905));
#55949=CARTESIAN_POINT('Origin',(0.,0.,24.1514101080949));
#55950=CARTESIAN_POINT('',(-4.37688026104952,0.00226901643694793,26.651410108095));
#55951=CARTESIAN_POINT('',(-4.36558297706963,0.00185075076461538,26.848589891905));
#55952=CARTESIAN_POINT('',(-4.372,3.82579154166093E-12,24.1514101080949));
#55953=CARTESIAN_POINT('Ctrl Pts',(-4.37688026104952,0.00226901643694839,
26.651410108095));
#55954=CARTESIAN_POINT('Ctrl Pts',(-4.36778028862692,-1.29719233300268,
26.6988746758065));
#55955=CARTESIAN_POINT('Ctrl Pts',(-3.06703503858937,-4.06017418671544,
26.7992594975999));
#55956=CARTESIAN_POINT('Ctrl Pts',(1.63279456941769,-4.90302026906412,26.9525645734753));
#55957=CARTESIAN_POINT('Ctrl Pts',(5.00417945325775,-1.28762125191842,27.1113253357213));
#55958=CARTESIAN_POINT('Ctrl Pts',(3.79627275763131,3.50580663842047,27.2700860979671));
#55959=CARTESIAN_POINT('Ctrl Pts',(-0.886457053099411,5.09084367591115,
27.428846860213));
#55960=CARTESIAN_POINT('Ctrl Pts',(-3.98586478860146,2.62941579049566,27.5559548635889));
#55961=CARTESIAN_POINT('Ctrl Pts',(-4.3686443606578,0.588309625125352,27.6301426128829));
#55962=CARTESIAN_POINT('Ctrl Pts',(-4.36594998909341,0.00221597220681394,
27.651410108095));
#55963=CARTESIAN_POINT('Ctrl Pts',(-4.36558297706963,0.00185075076461511,
26.848589891905));
#55964=CARTESIAN_POINT('Ctrl Pts',(-4.36229437398082,-0.847147845875526,
26.879392076113));
#55965=CARTESIAN_POINT('Ctrl Pts',(-3.7134735047561,-3.15941742864277,26.963114514403));
#55966=CARTESIAN_POINT('Ctrl Pts',(0.037946527963305,-5.16730646950401,
27.0997572067749));
#55967=CARTESIAN_POINT('Ctrl Pts',(4.36170657063856,-2.77078223288025,27.2585179690208));
#55968=CARTESIAN_POINT('Ctrl Pts',(4.69358555482947,2.16156853417802,27.4172787312667));
#55969=CARTESIAN_POINT('Ctrl Pts',(0.729706757950081,5.11562647870316,27.5760394935125));
#55970=CARTESIAN_POINT('Ctrl Pts',(-3.46466751885718,3.55083973542589,27.719809880392));
#55971=CARTESIAN_POINT('Ctrl Pts',(-4.36096811322469,1.03907475143884,27.8106600131895));
#55972=CARTESIAN_POINT('Ctrl Pts',(-4.36984836444492,-0.00386263586949508,
27.848589891905));
#55973=CARTESIAN_POINT('Ctrl Pts',(-1.91898364243938,3.92834389788497,25.6709103465619));
#55974=CARTESIAN_POINT('Ctrl Pts',(-2.57208606313318,3.60930541889036,25.6973704736029));
#55975=CARTESIAN_POINT('Ctrl Pts',(-3.70615701990389,2.63929385761509,25.7502907276849));
#55976=CARTESIAN_POINT('Ctrl Pts',(-4.81803798679934,-0.15958129715831,
25.8561312358487));
#55977=CARTESIAN_POINT('Ctrl Pts',(-3.30234769881301,-3.97407004593024,
25.9884318710537));
#55978=CARTESIAN_POINT('Ctrl Pts',(1.55593458522165,-4.93043777696371,26.1471926332996));
#55979=CARTESIAN_POINT('Ctrl Pts',(4.98187809541805,-1.36671674862893,26.3059533955455));
#55980=CARTESIAN_POINT('Ctrl Pts',(3.85252000415521,3.44398917781397,26.4647141577913));
#55981=CARTESIAN_POINT('Ctrl Pts',(-0.805001512196143,5.10466442465425,
26.6234749200372));
#55982=CARTESIAN_POINT('Ctrl Pts',(-4.72460311480109,2.09234479401288,26.7822356822831));
#55983=CARTESIAN_POINT('Ctrl Pts',(-4.32070810303542,-2.83440458431113,
26.940996444529));
#55984=CARTESIAN_POINT('Ctrl Pts',(0.037946527963305,-5.16730646950401,
27.0997572067749));
#55985=CARTESIAN_POINT('Ctrl Pts',(4.36170657063856,-2.77078223288025,27.2585179690208));
#55986=CARTESIAN_POINT('Ctrl Pts',(4.69358555482947,2.16156853417802,27.4172787312667));
#55987=CARTESIAN_POINT('Ctrl Pts',(0.729706757950081,5.11562647870316,27.5760394935125));
#55988=CARTESIAN_POINT('Ctrl Pts',(-3.90199850336257,3.38768554797952,27.7348002557585));
#55989=CARTESIAN_POINT('Ctrl Pts',(-4.96248778940575,-1.44075757294651,
27.8935610180043));
#55990=CARTESIAN_POINT('Ctrl Pts',(-1.48115027726835,-4.95058115072351,
28.0523217802503));
#55991=CARTESIAN_POINT('Ctrl Pts',(3.35577787359124,-3.92947861571792,28.2110825424961));
#55992=CARTESIAN_POINT('Ctrl Pts',(5.12139735341277,0.688001195909337,28.369843304742));
#55993=CARTESIAN_POINT('Ctrl Pts',(2.1997566305386,4.67580212267651,28.5286040669879));
#55994=CARTESIAN_POINT('Ctrl Pts',(-2.7351680780718,4.38416569184913,28.6873648292338));
#55995=CARTESIAN_POINT('Ctrl Pts',(-5.16678366281907,0.0800071286185968,
28.8461255914797));
#55996=CARTESIAN_POINT('Ctrl Pts',(-2.86960088841888,-4.29737651997417,
29.0048863537256));
#55997=CARTESIAN_POINT('Ctrl Pts',(2.05392820456428,-4.74166985111631,29.1636471159715));
#55998=CARTESIAN_POINT('Ctrl Pts',(5.09763950196961,-0.846242130327758,
29.3224078782173));
#55999=CARTESIAN_POINT('Ctrl Pts',(3.47583539931961,3.82369225364773,29.4811686404633));
#56000=CARTESIAN_POINT('Ctrl Pts',(-1.32715942194175,4.9940666821606,29.6399294027091));
#56001=CARTESIAN_POINT('Ctrl Pts',(-4.9154974066526,1.59371874196162,29.798690164955));
#56002=CARTESIAN_POINT('Ctrl Pts',(-4.00502201634919,-3.26524927403143,
29.9574509272009));
#56003=CARTESIAN_POINT('Ctrl Pts',(0.570971856938151,-5.13576141485164,
30.1162116894468));
#56004=CARTESIAN_POINT('Ctrl Pts',(4.62439484690811,-2.30586783557282,30.2749724516927));
#56005=CARTESIAN_POINT('Ctrl Pts',(4.44543041863472,2.63442642081081,30.4337332139386));
#56006=CARTESIAN_POINT('Ctrl Pts',(0.1978722839815,5.16361314708889,30.5924939761844));
#56007=CARTESIAN_POINT('Ctrl Pts',(-4.23078460916092,2.96690339662622,30.7512547384304));
#56008=CARTESIAN_POINT('Ctrl Pts',(-4.7872981969476,-1.94520696772118,30.9100155006763));
#56009=CARTESIAN_POINT('Ctrl Pts',(-0.962330244988123,-5.07700449806455,
31.0687762629221));
#56010=CARTESIAN_POINT('Ctrl Pts',(3.74339174195905,-3.56217243267071,31.2275370251681));
#56011=CARTESIAN_POINT('Ctrl Pts',(5.02304726326813,1.21286865108392,31.3862977874139));
#56012=CARTESIAN_POINT('Ctrl Pts',(1.70545649826175,4.87785529780762,31.5450585496599));
#56013=CARTESIAN_POINT('Ctrl Pts',(-3.17302014780288,4.07847977994959,31.7038193119056));
#56014=CARTESIAN_POINT('Ctrl Pts',(-5.14745183343486,-0.453645011306304,
31.8625800741516));
#56015=CARTESIAN_POINT('Ctrl Pts',(-2.41077837014428,-4.57058003144683,
32.0213408363975));
#56016=CARTESIAN_POINT('Ctrl Pts',(2.53231309568674,-4.50438059662262,32.1801015986434));
#56017=CARTESIAN_POINT('Ctrl Pts',(5.15775426583447,-0.31563445167244,32.3388623608893));
#56018=CARTESIAN_POINT('Ctrl Pts',(3.06266118623515,4.16198998462816,32.4976231231351));
#56019=CARTESIAN_POINT('Ctrl Pts',(-1.83547296121064,4.83043405735769,32.6563838853811));
#56020=CARTESIAN_POINT('Ctrl Pts',(-5.05372618930481,1.07791733326401,32.8151446476269));
#56021=CARTESIAN_POINT('Ctrl Pts',(-3.64665484087083,-3.66114225964655,
32.9739054098729));
#56022=CARTESIAN_POINT('Ctrl Pts',(1.09794640645064,-5.04941262548215,33.1326661721187));
#56023=CARTESIAN_POINT('Ctrl Pts',(4.83767356537879,-1.81630632015957,33.2914269343646));
#56024=CARTESIAN_POINT('Ctrl Pts',(4.14981410860918,3.07913900917197,33.4501876966104));
#56025=CARTESIAN_POINT('Ctrl Pts',(-0.336081978081961,5.15646226378366,
33.6089484588564));
#56026=CARTESIAN_POINT('Ctrl Pts',(-4.51438557267483,2.51443374838985,33.7677092211023));
#56027=CARTESIAN_POINT('Ctrl Pts',(-4.56098559745287,-2.42888133790924,
33.9264699833482));
#56028=CARTESIAN_POINT('Ctrl Pts',(-0.433232286323001,-5.1492100326073,
34.085230745594));
#56029=CARTESIAN_POINT('Ctrl Pts',(4.0910284465022,-3.15682442079478,34.24399150784));
#56030=CARTESIAN_POINT('Ctrl Pts',(4.87105498299758,1.72478332738662,34.4027522700858));
#56031=CARTESIAN_POINT('Ctrl Pts',(1.1929432107418,5.02781669015105,34.5615130323318));
#56032=CARTESIAN_POINT('Ctrl Pts',(-3.5769866269097,3.72923864142877,34.7202737945776));
#56033=CARTESIAN_POINT('Ctrl Pts',(-5.07314904313429,-0.982452523006609,
34.8790345568235));
#56034=CARTESIAN_POINT('Ctrl Pts',(-1.92621049372714,-4.7949731289833,35.0377953190694));
#56035=CARTESIAN_POINT('Ctrl Pts',(2.98365473640471,-4.21898786295316,35.1965560813153));
#56036=CARTESIAN_POINT('Ctrl Pts',(5.16278801485838,0.21834396591395,35.3553168435612));
#56037=CARTESIAN_POINT('Ctrl Pts',(2.61678000270041,4.45584072777334,35.514077605807));
#56038=CARTESIAN_POINT('Ctrl Pts',(-2.32418499851494,4.61521595014736,35.672838368053));
#56039=CARTESIAN_POINT('Ctrl Pts',(-5.13798489593422,0.55060456133973,35.8315991302988));
#56040=CARTESIAN_POINT('Ctrl Pts',(-3.24934407480239,-4.01793694044132,
35.9903598925447));
#56041=CARTESIAN_POINT('Ctrl Pts',(1.61319569609569,-4.90913982484862,36.1491206547906));
#56042=CARTESIAN_POINT('Ctrl Pts',(4.99928949022287,-1.30734798992603,36.3078814170365));
#56043=CARTESIAN_POINT('Ctrl Pts',(3.80988083761225,3.49096865884117,36.4666421792824));
#56044=CARTESIAN_POINT('Ctrl Pts',(-0.866447131906533,5.09424415801081,
36.6254029415283));
#56045=CARTESIAN_POINT('Ctrl Pts',(-4.74977622033223,2.03511179805508,36.7841637037742));
#56046=CARTESIAN_POINT('Ctrl Pts',(-4.28596502810612,-2.88661704277997,
36.94292446602));
#56047=CARTESIAN_POINT('Ctrl Pts',(0.100492274349119,-5.16642579319712,
37.101685228266));
#56048=CARTESIAN_POINT('Ctrl Pts',(4.39497597774354,-2.71776384714963,37.2604459905118));
#56049=CARTESIAN_POINT('Ctrl Pts',(4.66704342001788,2.21827858698683,37.4192067527577));
#56050=CARTESIAN_POINT('Ctrl Pts',(0.66769016759438,5.12408470011126,37.5779675150036));
#56051=CARTESIAN_POINT('Ctrl Pts',(-3.9427535210732,3.34017197848871,37.7367282772495));
#56052=CARTESIAN_POINT('Ctrl Pts',(-4.94466875428017,-1.50076816472822,
37.8954890394954));
#56053=CARTESIAN_POINT('Ctrl Pts',(-1.42107210669624,-4.96815944202542,
38.0542498017413));
#56054=CARTESIAN_POINT('Ctrl Pts',(3.40313314014881,-3.88853944357485,38.2130105639872));
#56055=CARTESIAN_POINT('Ctrl Pts',(5.11268698707437,0.749990630619295,38.3717713262331));
#56056=CARTESIAN_POINT('Ctrl Pts',(2.14295353437204,4.70210637090854,38.5305320884789));
#56057=CARTESIAN_POINT('Ctrl Pts',(-2.78807645035559,4.35071073283309,38.6892928507248));
#56058=CARTESIAN_POINT('Ctrl Pts',(-5.16737370481374,0.0174117378790549,
38.8480536129707));
#56059=CARTESIAN_POINT('Ctrl Pts',(-2.81733270514135,-4.33182301143032,
39.0068143752166));
#56060=CARTESIAN_POINT('Ctrl Pts',(2.11121724282438,-4.71644102342194,39.1655751374625));
#56061=CARTESIAN_POINT('Ctrl Pts',(5.10751668218689,-0.784428145210908,
39.3243358997084));
#56062=CARTESIAN_POINT('Ctrl Pts',(3.42926084288352,3.86551733216684,39.4830966619543));
#56063=CARTESIAN_POINT('Ctrl Pts',(-1.38755926796319,4.97762327338117,39.6418574242002));
#56064=CARTESIAN_POINT('Ctrl Pts',(-4.93444275322028,1.53405635131447,39.8006181864461));
#56065=CARTESIAN_POINT('Ctrl Pts',(-3.96517350621375,-3.31352580183661,
39.959378948692));
#56066=CARTESIAN_POINT('Ctrl Pts',(0.6331436514814,-5.12846792818335,40.1181397109379));
#56067=CARTESIAN_POINT('Ctrl Pts',(4.65198839971611,-2.2496795555641,40.2769004731838));
#56068=CARTESIAN_POINT('Ctrl Pts',(4.41319126769477,2.68808426366416,40.4356612354296));
#56069=CARTESIAN_POINT('Ctrl Pts',(0.135306684796697,5.16563125618407,40.5944219976755));
#56070=CARTESIAN_POINT('Ctrl Pts',(-4.26641470902384,2.91543473678309,40.7531827599214));
#56071=CARTESIAN_POINT('Ctrl Pts',(-4.7633830418116,-2.00305670683536,40.9119435221673));
#56072=CARTESIAN_POINT('Ctrl Pts',(-0.90075771530386,-5.08828946819429,
41.0707042844132));
#56073=CARTESIAN_POINT('Ctrl Pts',(3.78626858625262,-3.51656428443629,41.2294650466591));
#56074=CARTESIAN_POINT('Ctrl Pts',(5.00798622459088,1.27362794729248,41.3882258089049));
#56075=CARTESIAN_POINT('Ctrl Pts',(1.64624189925253,4.89815697818699,41.5469865711509));
#56076=CARTESIAN_POINT('Ctrl Pts',(-3.22219329739529,4.03974312649174,41.7057473333967));
#56077=CARTESIAN_POINT('Ctrl Pts',(-5.14157876509112,-0.515967030129218,
41.8645080956427));
#56078=CARTESIAN_POINT('Ctrl Pts',(-2.35523429540729,-4.59944840035779,
42.0232688578885));
#56079=CARTESIAN_POINT('Ctrl Pts',(2.58669254300161,-4.47337410259821,42.1820296201345));
#56080=CARTESIAN_POINT('Ctrl Pts',(5.16119935450289,-0.253131185149624,
42.3407903823802));
#56081=CARTESIAN_POINT('Ctrl Pts',(3.01201886587614,4.19878512494061,42.4995511446263));
#56082=CARTESIAN_POINT('Ctrl Pts',(-1.89385329211466,4.80784503512363,42.6583119068721));
#56083=CARTESIAN_POINT('Ctrl Pts',(-5.0664130686601,1.01661831162269,42.817072669118));
#56084=CARTESIAN_POINT('Ctrl Pts',(-3.6020368491656,-3.70504854368597,42.9758334313639));
#56085=CARTESIAN_POINT('Ctrl Pts',(1.15903352033341,-5.0357417996319,43.1345941936098));
#56086=CARTESIAN_POINT('Ctrl Pts',(4.85932100888344,-1.75757034181863,43.2933549558556));
#56087=CARTESIAN_POINT('Ctrl Pts',(4.11220948021047,3.12918317851219,43.4521157181016));
#56088=CARTESIAN_POINT('Ctrl Pts',(-0.398521773825228,5.15201267172389,
43.6108764803474));
#56089=CARTESIAN_POINT('Ctrl Pts',(-4.54451372744996,2.45956279749778,43.7696372425933));
#56090=CARTESIAN_POINT('Ctrl Pts',(-4.53122790373328,-2.48395407732217,
43.9283980048393));
#56091=CARTESIAN_POINT('Ctrl Pts',(-0.370823894361365,-5.15408030721166,
44.0871587670851));
#56092=CARTESIAN_POINT('Ctrl Pts',(4.12896947009338,-3.10703480650815,44.245919529331));
#56093=CARTESIAN_POINT('Ctrl Pts',(4.84980385450403,1.78366385472551,44.4046802915768));
#56094=CARTESIAN_POINT('Ctrl Pts',(1.13194961208497,5.04189887339256,44.5634410538228));
#56095=CARTESIAN_POINT('Ctrl Pts',(-3.62189949116538,3.68563403632435,44.7222018160687));
#56096=CARTESIAN_POINT('Ctrl Pts',(-5.06087554774066,-1.0438356499454,44.8809625783145));
#56097=CARTESIAN_POINT('Ctrl Pts',(-1.8679837165673,-4.81795506501003,45.0397233405604));
#56098=CARTESIAN_POINT('Ctrl Pts',(3.03454387031403,-4.18253483822383,45.1984841028063));
#56099=CARTESIAN_POINT('Ctrl Pts',(5.15976421573454,0.280869029694986,45.3572448650522));
#56100=CARTESIAN_POINT('Ctrl Pts',(2.56261074386464,4.4872129823807,45.5160056272982));
#56101=CARTESIAN_POINT('Ctrl Pts',(-2.37992235675453,4.58672254988638,45.6747663895439));
#56102=CARTESIAN_POINT('Ctrl Pts',(-5.14427782079704,0.488323536471552,
45.8335271517899));
#56103=CARTESIAN_POINT('Ctrl Pts',(-3.20043308923407,-4.05700409355871,
45.9922879140358));
#56104=CARTESIAN_POINT('Ctrl Pts',(1.67254576409749,-4.88923765436041,46.1510486762816));
#56105=CARTESIAN_POINT('Ctrl Pts',(5.01475964555148,-1.2466915701828,46.3098094385276));
#56106=CARTESIAN_POINT('Ctrl Pts',(3.76731232156889,3.53686471971598,46.4685702007735));
#56107=CARTESIAN_POINT('Ctrl Pts',(-0.928094313166731,5.08337438319113,
46.6273309630193));
#56108=CARTESIAN_POINT('Ctrl Pts',(-4.77408068348225,1.97742453747749,46.7860917252652));
#56109=CARTESIAN_POINT('Ctrl Pts',(-4.25068258608159,-2.93832464615453,
46.9448524875111));
#56110=CARTESIAN_POINT('Ctrl Pts',(0.163070052891163,-5.16482936133098,
47.103613249757));
#56111=CARTESIAN_POINT('Ctrl Pts',(4.42757599841828,-2.66432448325026,47.2623740120029));
#56112=CARTESIAN_POINT('Ctrl Pts',(4.63982914812316,2.27465154475207,47.4211347742487));
#56113=CARTESIAN_POINT('Ctrl Pts',(0.605568936039063,5.13179699886122,47.5798955364947));
#56114=CARTESIAN_POINT('Ctrl Pts',(-3.982926463652,3.29216508683222,47.7386562987406));
#56115=CARTESIAN_POINT('Ctrl Pts',(-4.92612590373581,-1.56055687315755,
47.8974170609864));
#56116=CARTESIAN_POINT('Ctrl Pts',(-1.36078444624568,-4.98500951500319,
48.0561778232324));
#56117=CARTESIAN_POINT('Ctrl Pts',(3.44998850215064,-3.84702917961962,48.2149385854782));
#56118=CARTESIAN_POINT('Ctrl Pts',(5.10322659210776,0.811869769988193,48.3736993477241));
#56119=CARTESIAN_POINT('Ctrl Pts',(2.08583582488191,4.72772070721777,48.53246010997));
#56120=CARTESIAN_POINT('Ctrl Pts',(-2.8405756019607,4.31661724309231,48.6912208722158));
#56121=CARTESIAN_POINT('Ctrl Pts',(-5.16720547137737,-0.0451861747017031,
48.8499816344618));
#56122=CARTESIAN_POINT('Ctrl Pts',(-2.76465105904324,-4.36563382517906,
49.0087423967076));
#56123=CARTESIAN_POINT('Ctrl Pts',(2.16819644989342,-4.69052004883103,49.1675031589536));
#56124=CARTESIAN_POINT('Ctrl Pts',(5.11664433946473,-0.72249904999246,49.3262639211995));
#56125=CARTESIAN_POINT('Ctrl Pts',(3.38218303962157,3.90677514842007,49.4850246834453));
#56126=CARTESIAN_POINT('Ctrl Pts',(-1.44775548820939,4.96044939699782,49.6437854456913));
#56127=CARTESIAN_POINT('Ctrl Pts',(-4.95266397096391,1.47416883854343,49.8025462079371));
#56128=CARTESIAN_POINT('Ctrl Pts',(-3.92474310640146,-3.36131607001936,
49.961306970183));
#56129=CARTESIAN_POINT('Ctrl Pts',(0.695222531978707,-5.12042183856424,
50.1200677324289));
#56130=CARTESIAN_POINT('Ctrl Pts',(4.67889927324325,-2.19316113513354,50.2788284946747));
#56131=CARTESIAN_POINT('Ctrl Pts',(4.38030448079635,2.74134763015048,50.4375892569207));
#56132=CARTESIAN_POINT('Ctrl Pts',(0.0727212293821569,5.16689130876717,
50.5963500191666));
#56133=CARTESIAN_POINT('Ctrl Pts',(-4.30141871246148,2.86353823685011,50.7551107814125));
#56134=CARTESIAN_POINT('Ctrl Pts',(-4.73876886011502,-2.06061249734653,
50.9138715436583));
#56135=CARTESIAN_POINT('Ctrl Pts',(-0.839052999411725,-5.09882773174331,
51.0726323059043));
#56136=CARTESIAN_POINT('Ctrl Pts',(3.82858979556074,-3.47044008032763,51.2313930681501));
#56137=CARTESIAN_POINT('Ctrl Pts',(4.99219026383802,1.33420033857639,51.390153830396));
#56138=CARTESIAN_POINT('Ctrl Pts',(1.58678571421362,4.91773985393535,51.548914592642));
#56139=CARTESIAN_POINT('Ctrl Pts',(-3.27089359005984,4.00041364065291,51.7076753548878));
#56140=CARTESIAN_POINT('Ctrl Pts',(-5.1349511699649,-0.578213330780779,
51.8664361171337));
#56141=CARTESIAN_POINT('Ctrl Pts',(-2.2993445899923,-4.62764180012773,52.0251968793796));
#56142=CARTESIAN_POINT('Ctrl Pts',(2.64069239313623,-4.44171114083851,52.1839576416255));
#56143=CARTESIAN_POINT('Ctrl Pts',(5.16388703706709,-0.190590771620509,
52.3427184038713));
#56144=CARTESIAN_POINT('Ctrl Pts',(2.96093453169081,4.23496409345547,52.5014791661172));
#56145=CARTESIAN_POINT('Ctrl Pts',(-1.95195570001178,4.78455046153847,52.6602399283632));
#56146=CARTESIAN_POINT('Ctrl Pts',(-5.07835645180041,0.955170101224678,
52.819000690609));
#56147=CARTESIAN_POINT('Ctrl Pts',(-3.5568902584837,-3.7484111117806,52.9777614528549));
#56148=CARTESIAN_POINT('Ctrl Pts',(1.21995054602492,-5.021331978576,53.1365222151008));
#56149=CARTESIAN_POINT('Ctrl Pts',(4.88025534693686,-1.69857643999627,53.2952829773467));
#56150=CARTESIAN_POINT('Ctrl Pts',(4.07400138499168,3.17876814016096,53.4540437395925));
#56151=CARTESIAN_POINT('Ctrl Pts',(-0.460903086490536,5.14680702170578,
53.6128045018385));
#56152=CARTESIAN_POINT('Ctrl Pts',(-4.57397497474849,2.404330905718,53.7715652640843));
#56153=CARTESIAN_POINT('Ctrl Pts',(-4.5008052522319,-2.53866229642665,53.9303260263303));
#56154=CARTESIAN_POINT('Ctrl Pts',(-0.308361083986154,-5.15819422043212,
54.0890867885761));
#56155=CARTESIAN_POINT('Ctrl Pts',(4.16630456733569,-3.05678923480409,54.2478475508221));
#56156=CARTESIAN_POINT('Ctrl Pts',(4.82784101720183,1.84228262935957,54.4066083130679));
#56157=CARTESIAN_POINT('Ctrl Pts',(1.07078989980086,5.0552411578777,54.5653690753139));
#56158=CARTESIAN_POINT('Ctrl Pts',(-3.66628084160122,3.64148856435446,54.7241298375597));
#56159=CARTESIAN_POINT('Ctrl Pts',(-5.04785936876341,-1.10506559398251,
54.8828905998056));
#56160=CARTESIAN_POINT('Ctrl Pts',(-1.80948281276126,-4.84022996603858,
55.0416513620516));
#56161=CARTESIAN_POINT('Ctrl Pts',(3.08498768485217,-4.1454680264268,55.2004121242973));
#56162=CARTESIAN_POINT('Ctrl Pts',(5.15598322111311,0.34335287594041,55.3591728865433));
#56163=CARTESIAN_POINT('Ctrl Pts',(2.50806542185317,4.51792673839683,55.5179336487891));
#56164=CARTESIAN_POINT('Ctrl Pts',(-2.43531046134262,4.55755604800332,55.6766944110351));
#56165=CARTESIAN_POINT('Ctrl Pts',(-5.14981582279099,0.425970850115064,
55.8354551732808));
#56166=CARTESIAN_POINT('Ctrl Pts',(-3.15105244004859,-4.09547588124754,
55.9942159355269));
#56167=CARTESIAN_POINT('Ctrl Pts',(1.73165038597632,-4.86861798815274,56.1529766977727));
#56168=CARTESIAN_POINT('Ctrl Pts',(5.02949388480597,-1.18585219842773,56.3117374600186));
#56169=CARTESIAN_POINT('Ctrl Pts',(3.72419095237009,3.58224174562538,56.4704982222645));
#56170=CARTESIAN_POINT('Ctrl Pts',(-0.989605296568694,5.07175862308326,
56.6292589845104));
#56171=CARTESIAN_POINT('Ctrl Pts',(-4.79768455020047,1.91944708981109,56.7880197467563));
#56172=CARTESIAN_POINT('Ctrl Pts',(-4.21477635630603,-2.98960105033098,
56.9467805090022));
#56173=CARTESIAN_POINT('Ctrl Pts',(0.225623900899773,-5.162474990657,57.1055412712481));
#56174=CARTESIAN_POINT('Ctrl Pts',(4.45952627223033,-2.61049412968195,57.2643020334939));
#56175=CARTESIAN_POINT('Ctrl Pts',(4.61193398121205,2.33069069735948,57.4230627957398));
#56176=CARTESIAN_POINT('Ctrl Pts',(0.543358837230748,5.13875620630321,57.5818235579857));
#56177=CARTESIAN_POINT('Ctrl Pts',(-4.02251491169591,3.24367506988608,57.7405843202316));
#56178=CARTESIAN_POINT('Ctrl Pts',(-4.90686014412063,-1.62011656983585,
57.8993450824775));
#56179=CARTESIAN_POINT('Ctrl Pts',(-1.30029709065152,-5.00112803773905,
58.0581058447233));
#56180=CARTESIAN_POINT('Ctrl Pts',(3.49633757827368,-3.80495436405849,58.2168666069693));
#56181=CARTESIAN_POINT('Ctrl Pts',(5.09301729854088,0.873629767452735,58.3756273692151));
#56182=CARTESIAN_POINT('Ctrl Pts',(2.02841201894453,4.75264125042254,58.5343881314611));
#56183=CARTESIAN_POINT('Ctrl Pts',(-2.89265789904175,4.2818902896884,58.6931488937069));
#56184=CARTESIAN_POINT('Ctrl Pts',(-5.16627895043901,-0.107777456210482,
58.8519096559528));
#56185=CARTESIAN_POINT('Ctrl Pts',(-2.71156370034918,-4.39880398208026,
59.0106704181988));
#56186=CARTESIAN_POINT('Ctrl Pts',(2.22485747409188,-4.66391074033302,59.1694311804446));
#56187=CARTESIAN_POINT('Ctrl Pts',(5.12502112908765,-0.660463928024547,
59.3281919426906));
#56188=CARTESIAN_POINT('Ctrl Pts',(3.33460890093368,3.94745964534539,59.4869527049363));
#56189=CARTESIAN_POINT('Ctrl Pts',(-1.5077392503099,4.94254757457034,59.6457134671823));
#56190=CARTESIAN_POINT('Ctrl Pts',(-4.97015838517481,1.41406499146713,59.8044742294282));
#56191=CARTESIAN_POINT('Ctrl Pts',(-3.88373675046313,-3.40861306500439,
59.963234991674));
#56192=CARTESIAN_POINT('Ctrl Pts',(0.757199388556149,-5.11162432694214,
60.12199575392));
#56193=CARTESIAN_POINT('Ctrl Pts',(4.70512351821232,-2.13632086826434,60.2807565161658));
#56194=CARTESIAN_POINT('Ctrl Pts',(4.34677488413138,2.79420870381954,60.4395172784118));
#56195=CARTESIAN_POINT('Ctrl Pts',(0.0101251021257834,5.16739311995163,
60.5982780406576));
#56196=CARTESIAN_POINT('Ctrl Pts',(-4.33579148262063,2.81122151262594,60.7570388029036));
#56197=CARTESIAN_POINT('Ctrl Pts',(-4.71345926399734,-2.11786589293417,
60.9157995651493));
#56198=CARTESIAN_POINT('Ctrl Pts',(-0.777225152475865,-5.10861774222493,
61.0745603273954));
#56199=CARTESIAN_POINT('Ctrl Pts',(3.87034915924295,-3.42380658907068,61.2333210896411));
#56200=CARTESIAN_POINT('Ctrl Pts',(4.97566169906822,1.39457693593507,61.3920818518871));
#56201=CARTESIAN_POINT('Ctrl Pts',(1.52709666834069,4.93660105126586,61.550842614133));
#56202=CARTESIAN_POINT('Ctrl Pts',(-3.3191138790273,3.96049709403562,61.7096033763789));
#56203=CARTESIAN_POINT('Ctrl Pts',(-5.12757002065602,-0.640374778614905,
61.8683641386248));
#56204=CARTESIAN_POINT('Ctrl Pts',(-2.24311745571471,-4.65515609337478,
62.0271249008706));
#56205=CARTESIAN_POINT('Ctrl Pts',(2.69430472161155,-4.40939635788372,62.1858856631165));
#56206=CARTESIAN_POINT('Ctrl Pts',(5.16581691910958,-0.128022388891978,
62.3446464253625));
#56207=CARTESIAN_POINT('Ctrl Pts',(2.90941568030617,4.27052158090844,62.5034071876082));
#56208=CARTESIAN_POINT('Ctrl Pts',(-2.00977165837252,4.76055375508134,62.6621679498542));
#56209=CARTESIAN_POINT('Ctrl Pts',(-5.08955458603407,0.893581719595941,
62.8209287121001));
#56210=CARTESIAN_POINT('Ctrl Pts',(-3.51122169408817,-3.79122360047265,
62.9796894743459));
#56211=CARTESIAN_POINT('Ctrl Pts',(1.28068854395033,-5.00618527695598,63.1384502365919));
#56212=CARTESIAN_POINT('Ctrl Pts',(4.90047350742458,-1.63933327204883,63.2972109988377));
#56213=CARTESIAN_POINT('Ctrl Pts',(4.03519542999152,3.22788661752423,63.4559717610837));
#56214=CARTESIAN_POINT('Ctrl Pts',(-0.523216761619089,5.14084607765855,
63.6147325233295));
#56215=CARTESIAN_POINT('Ctrl Pts',(-4.60276499113179,2.34874617833169,63.7734932855755));
#56216=CARTESIAN_POINT('Ctrl Pts',(-4.46972210747346,-2.59299796679048,
63.9322540478212));
#56217=CARTESIAN_POINT('Ctrl Pts',(-0.245853021615901,-5.16155116855183,
64.0910148100673));
#56218=CARTESIAN_POINT('Ctrl Pts',(4.20302825930282,-3.00609507922124,64.249775572313));
#56219=CARTESIAN_POINT('Ctrl Pts',(4.80516969413782,1.90063104898239,64.408536334559));
#56220=CARTESIAN_POINT('Ctrl Pts',(1.00947304907845,5.06784158562605,64.5672970968048));
#56221=CARTESIAN_POINT('Ctrl Pts',(-3.71012416525332,3.59680870386789,64.7260578590508));
#56222=CARTESIAN_POINT('Ctrl Pts',(-5.03410241632698,-1.16613336962256,
64.8848186212966));
#56223=CARTESIAN_POINT('Ctrl Pts',(-1.75071636731768,-4.86179456322688,
65.0435793835425));
#56224=CARTESIAN_POINT('Ctrl Pts',(3.1349787773885,-4.10779286711735,65.2023401457884));
#56225=CARTESIAN_POINT('Ctrl Pts',(5.15144558585509,0.405786335144852,65.3611009080343));
#56226=CARTESIAN_POINT('Ctrl Pts',(2.45315204119292,4.54797748857745,65.5198616702802));
#56227=CARTESIAN_POINT('Ctrl Pts',(-2.49034118407384,4.52772072468283,65.6786224325261));
#56228=CARTESIAN_POINT('Ctrl Pts',(-5.15459808921429,0.363555652528053,
65.837383194772));
#56229=CARTESIAN_POINT('Ctrl Pts',(-3.10120937385697,-4.13334665777235,
65.9961439570178));
#56230=CARTESIAN_POINT('Ctrl Pts',(1.79050088812788,-4.84728385216189,66.1549047192638));
#56231=CARTESIAN_POINT('Ctrl Pts',(5.04349004573647,-1.12483880283976,66.3136654815096));
#56232=CARTESIAN_POINT('Ctrl Pts',(3.68052305807757,3.62709307749002,66.4724262437556));
#56233=CARTESIAN_POINT('Ctrl Pts',(-1.05097105537457,5.05939858230018,66.6311870060014));
#56234=CARTESIAN_POINT('Ctrl Pts',(-4.82058435661895,1.86118796324735,66.7899477682473));
#56235=CARTESIAN_POINT('Ctrl Pts',(-4.17825160801934,-3.04043873049599,
66.9487085304932));
#56236=CARTESIAN_POINT('Ctrl Pts',(0.288144638596748,-5.15936302667923,
67.1074692927391));
#56237=CARTESIAN_POINT('Ctrl Pts',(4.49082211047655,-2.55628068604989,67.266230054985));
#56238=CARTESIAN_POINT('Ctrl Pts',(4.58336201290063,2.38638782106256,67.4249908172308));
#56239=CARTESIAN_POINT('Ctrl Pts',(0.481069000502546,5.14496130117338,67.5837515794768));
#56240=CARTESIAN_POINT('Ctrl Pts',(-4.06151305559941,3.19470904356121,67.7425123417227));
#56241=CARTESIAN_POINT('Ctrl Pts',(-4.88687430268524,-1.67943851437657,
67.9012731039685));
#56242=CARTESIAN_POINT('Ctrl Pts',(-1.23961891643423,-5.01651264483955,
68.0600338662145));
#56243=CARTESIAN_POINT('Ctrl Pts',(3.54217356679019,-3.76232117137135,68.2187946284603));
#56244=CARTESIAN_POINT('Ctrl Pts',(5.08206060458778,0.935261559732356,68.3775553907062));
#56245=CARTESIAN_POINT('Ctrl Pts',(1.97069054350433,4.77686434343271,68.5363161529522));
#56246=CARTESIAN_POINT('Ctrl Pts',(-2.9443156985208,4.2465349688023,68.695076915198));
#56247=CARTESIAN_POINT('Ctrl Pts',(-5.16459427796565,-0.170352921375672,
68.8538376774439));
#56248=CARTESIAN_POINT('Ctrl Pts',(-2.65807841962993,-4.43132861441282,
69.0125984396897));
#56249=CARTESIAN_POINT('Ctrl Pts',(2.2811920004135,-4.63661700284439,69.1713592019357));
#56250=CARTESIAN_POINT('Ctrl Pts',(5.1326458217616,-0.598331882962418,69.3301199641815));
#56251=CARTESIAN_POINT('Ctrl Pts',(3.28654540832559,3.98756485249208,69.4888807264275));
#56252=CARTESIAN_POINT('Ctrl Pts',(-1.56750175164667,4.92392043319156,69.6476414886732));
#56253=CARTESIAN_POINT('Ctrl Pts',(-4.98692342854749,1.35375363032602,69.8064022509193));
#56254=CARTESIAN_POINT('Ctrl Pts',(-3.84216045608199,-3.45540984595692,
69.965163013165));
#56255=CARTESIAN_POINT('Ctrl Pts',(0.819065126108891,-5.102076684352,70.1239237754111));
#56256=CARTESIAN_POINT('Ctrl Pts',(4.73065728621489,-2.07916709626671,70.2826845376568));
#56257=CARTESIAN_POINT('Ctrl Pts',(4.31260739816882,2.84665972730784,70.4414452999028));
#56258=CARTESIAN_POINT('Ctrl Pts',(-0.0524725109896868,5.16713661609669,
70.6002060621488));
#56259=CARTESIAN_POINT('Ctrl Pts',(-4.36952797529665,2.75849224159072,70.7589668243945));
#56260=CARTESIAN_POINT('Ctrl Pts',(-4.68745796764224,-2.17480849166161,
70.9177275866405));
#56261=CARTESIAN_POINT('Ctrl Pts',(-0.715283247733823,-5.11765806295492,
71.0764883488864));
#56262=CARTESIAN_POINT('Ctrl Pts',(3.91154054911197,-3.37667065413102,71.2352491111322));
#56263=CARTESIAN_POINT('Ctrl Pts',(4.95840295584866,1.45474887910182,71.3940098733782));
#56264=CARTESIAN_POINT('Ctrl Pts',(1.46718352100222,4.95473780229749,71.552770635624));
#56265=CARTESIAN_POINT('Ctrl Pts',(-3.36684708796952,3.91999934439373,71.7115313978699));
#56266=CARTESIAN_POINT('Ctrl Pts',(-5.11943640034826,-0.702442251438138,
71.8702921601158));
#56267=CARTESIAN_POINT('Ctrl Pts',(-2.18656114390733,-4.68198724237597,
72.0290529223616));
#56268=CARTESIAN_POINT('Ctrl Pts',(2.74752166081747,-4.3764344959288,72.1878136846077));
#56269=CARTESIAN_POINT('Ctrl Pts',(5.16698871742013,-0.0654352188752399,
72.3465744468534));
#56270=CARTESIAN_POINT('Ctrl Pts',(2.85746987211454,4.30545236923763,72.5053352090995));
#56271=CARTESIAN_POINT('Ctrl Pts',(-2.06729268270395,4.73585843726931,72.6640959713451));
#56272=CARTESIAN_POINT('Ctrl Pts',(-5.10000582803462,0.831862204832684,
72.8228567335913));
#56273=CARTESIAN_POINT('Ctrl Pts',(-3.46503785784167,-3.83347972702879,
72.9816174958369));
#56274=CARTESIAN_POINT('Ctrl Pts',(1.34123860080759,-4.99030391755056,73.140378258083));
#56275=CARTESIAN_POINT('Ctrl Pts',(4.91997252333115,-1.57984953191204,73.2991390203287));
#56276=CARTESIAN_POINT('Ctrl Pts',(3.99579730998455,3.27653140246455,73.4578997825747));
#56277=CARTESIAN_POINT('Ctrl Pts',(-0.585453654677876,5.13413071435083,
73.6166605448206));
#56278=CARTESIAN_POINT('Ctrl Pts',(-4.63087955166449,2.29281677239862,73.7754213070665));
#56279=CARTESIAN_POINT('Ctrl Pts',(-4.43798303090997,-2.64695311465312,
73.9341820693124));
#56280=CARTESIAN_POINT('Ctrl Pts',(-0.183308880309829,-5.16415065893858,
74.0929428315583));
#56281=CARTESIAN_POINT('Ctrl Pts',(4.23913515679244,-2.95495977912772,74.2517035938041));
#56282=CARTESIAN_POINT('Ctrl Pts',(4.78179321232898,1.95870055096247,74.4104643560501));
#56283=CARTESIAN_POINT('Ctrl Pts',(0.948008058166557,5.07969830752458,74.5692251182959));
#56284=CARTESIAN_POINT('Ctrl Pts',(-3.75342302811316,3.55160101163497,74.7279858805418));
#56285=CARTESIAN_POINT('Ctrl Pts',(-5.01960670926438,-1.22703001516843,
74.8867466427878));
#56286=CARTESIAN_POINT('Ctrl Pts',(-1.69169300421356,-4.88264569196979,
75.0455074050335));
#56287=CARTESIAN_POINT('Ctrl Pts',(3.18450981172911,-4.06951488912588,75.2042681672795));
#56288=CARTESIAN_POINT('Ctrl Pts',(5.14615197585861,0.468160245196775,75.3630289295254));
#56289=CARTESIAN_POINT('Ctrl Pts',(2.39787866042351,4.57736082297456,75.5217896917712));
#56290=CARTESIAN_POINT('Ctrl Pts',(-2.54500644918866,4.49722095825909,75.6805504540172));
#56291=CARTESIAN_POINT('Ctrl Pts',(-5.15862391826907,0.301087103142032,
75.839311216263));
#56292=CARTESIAN_POINT('Ctrl Pts',(-3.05091120513038,-4.17061086559584,
75.9980719785089));
#56293=CARTESIAN_POINT('Ctrl Pts',(1.84908863423975,-4.82523837717284,76.1568327407549));
#56294=CARTESIAN_POINT('Ctrl Pts',(5.05674607440601,-1.06366033713594,76.3155935030006));
#56295=CARTESIAN_POINT('Ctrl Pts',(3.63631504695578,3.6714121333759,76.4743542652466));
#56296=CARTESIAN_POINT('Ctrl Pts',(-1.11218258415778,5.04629607467818,76.6331150274925));
#56297=CARTESIAN_POINT('Ctrl Pts',(-4.84277674219067,1.80265570731443,76.7918757897383));
#56298=CARTESIAN_POINT('Ctrl Pts',(-4.1411137012291,-3.09083022621898,76.9506365519843));
#56299=CARTESIAN_POINT('Ctrl Pts',(0.350623091062388,-5.15549392607834,
77.1093973142301));
#56300=CARTESIAN_POINT('Ctrl Pts',(4.52145892049186,-2.50169210817825,77.268158076476));
#56301=CARTESIAN_POINT('Ctrl Pts',(4.55411743612604,2.44173474230699,77.4269188387219));
#56302=CARTESIAN_POINT('Ctrl Pts',(0.4187085668894,5.15041137287398,77.5856796009678));
#56303=CARTESIAN_POINT('Ctrl Pts',(-4.09991517238411,3.14527419362299,77.7444403632137));
#56304=CARTESIAN_POINT('Ctrl Pts',(-4.86617131235222,-1.738514001283,77.9032011254596));
#56305=CARTESIAN_POINT('Ctrl Pts',(-1.17875882811733,-5.03116107861318,
78.0619618877055));
#56306=CARTESIAN_POINT('Ctrl Pts',(3.58748974126774,-3.71913585798031,78.2207226499514));
#56307=CARTESIAN_POINT('Ctrl Pts',(5.07035811814355,0.996756102360001,78.3794834121972));
#56308=CARTESIAN_POINT('Ctrl Pts',(1.91267986918918,4.80038643150889,78.5382441744432));
#56309=CARTESIAN_POINT('Ctrl Pts',(-2.99554141961442,4.21055646882815,78.697004936689));
#56310=CARTESIAN_POINT('Ctrl Pts',(-5.16215170118294,-0.232903387246084,
78.855765698935));
#56311=CARTESIAN_POINT('Ctrl Pts',(-2.60420306585193,-4.46320294918618,
79.0145264611808));
#56312=CARTESIAN_POINT('Ctrl Pts',(2.33719176176521,-4.60864284172174,79.1732872234268));
#56313=CARTESIAN_POINT('Ctrl Pts',(5.13951729856278,-0.536112032685121,
79.3320479856725));
#56314=CARTESIAN_POINT('Ctrl Pts',(3.23799961511593,4.02708488442023,79.4908087479186));
#56315=CARTESIAN_POINT('Ctrl Pts',(-1.62703422207133,4.90457070639472,79.6495695101643));
#56316=CARTESIAN_POINT('Ctrl Pts',(-5.00295664081116,1.29324360581397,79.8083302724103));
#56317=CARTESIAN_POINT('Ctrl Pts',(-3.80002032458076,-3.5016995454484,79.9670910346561));
#56318=CARTESIAN_POINT('Ctrl Pts',(0.880810665839244,-5.09178031191025,
80.125851796902));
#56319=CARTESIAN_POINT('Ctrl Pts',(4.75549683016874,-2.02170820645871,80.2846125591479));
#56320=CARTESIAN_POINT('Ctrl Pts',(4.27780703699033,2.89869300342805,80.4433733213939));
#56321=CARTESIAN_POINT('Ctrl Pts',(-0.11506242376767,5.16612183484124,80.6021340836397));
#56322=CARTESIAN_POINT('Ctrl Pts',(-4.40262323964949,2.70535816177208,80.7608948458856));
#56323=CARTESIAN_POINT('Ctrl Pts',(-4.66076878675771,-2.23143193721207,
80.9196556081315));
#56324=CARTESIAN_POINT('Ctrl Pts',(-0.653236375128765,-5.12594736724498,
81.0784163703773));
#56325=CARTESIAN_POINT('Ctrl Pts',(3.95215792026738,-3.32903919274863,81.2371771326234));
#56326=CARTESIAN_POINT('Ctrl Pts',(4.94041656702063,1.51470733791976,81.3959378948691));
#56327=CARTESIAN_POINT('Ctrl Pts',(1.40705506422376,4.97214744531344,81.5546986571151));
#56328=CARTESIAN_POINT('Ctrl Pts',(-3.41408621159557,3.87892633505682,81.713459419361));
#56329=CARTESIAN_POINT('Ctrl Pts',(-5.11055150349599,-0.76440664139103,
81.8722201816067));
#56330=CARTESIAN_POINT('Ctrl Pts',(-2.12968395259116,-4.7081313086182,82.0309809438528));
#56331=CARTESIAN_POINT('Ctrl Pts',(2.80033539806548,-4.3428303941221,82.1897417060986));
#56332=CARTESIAN_POINT('Ctrl Pts',(5.16740226597732,-0.00283844241944707,
82.3485024683445));
#56333=CARTESIAN_POINT('Ctrl Pts',(2.80510471878759,4.33975132503298,82.5072632305904));
#56334=CARTESIAN_POINT('Ctrl Pts',(-2.12451031000386,4.71046814615349,82.6660239928362));
#56335=CARTESIAN_POINT('Ctrl Pts',(-5.10970868581842,0.770020587436124,
82.8247847550823));
#56336=CARTESIAN_POINT('Ctrl Pts',(-3.41834544728425,-3.87517323895607,
82.983545517328));
#56337=CARTESIAN_POINT('Ctrl Pts',(1.40159167776471,-4.9736903294079,83.142306279574));
#56338=CARTESIAN_POINT('Ctrl Pts',(4.93874982643145,-1.52013376024582,83.3010670418199));
#56339=CARTESIAN_POINT('Ctrl Pts',(3.95581224496304,3.32469499516411,83.4598278040656));
#56340=CARTESIAN_POINT('Ctrl Pts',(-0.647603556591826,5.12666260907039,
83.6185885663118));
#56341=CARTESIAN_POINT('Ctrl Pts',(-4.65831659106839,2.23654957051732,83.7773493285574));
#56342=CARTESIAN_POINT('Ctrl Pts',(-4.40558873364168,-2.70051728419629,
83.9361100908035));
#56343=CARTESIAN_POINT('Ctrl Pts',(-0.120745397495975,-5.1659971710397,
84.0948708530492));
#56344=CARTESIAN_POINT('Ctrl Pts',(4.27463443926266,-2.90338152834273,84.2536316152952));
#56345=CARTESIAN_POINT('Ctrl Pts',(4.75768727179541,2.01646478129229,84.412392377541));
#56346=CARTESIAN_POINT('Ctrl Pts',(0.886457060193665,5.09084373843816,84.571153139787));
#56347=CARTESIAN_POINT('Ctrl Pts',(-3.79627280569434,3.50580670373394,84.7299139020329));
#56348=CARTESIAN_POINT('Ctrl Pts',(-5.00417952636703,-1.28762129421282,
84.8886746642788));
#56349=CARTESIAN_POINT('Ctrl Pts',(-1.63279460579437,-4.90302030367583,
85.0474354265246));
#56350=CARTESIAN_POINT('Ctrl Pts',(3.23428855022947,-4.03017982392474,85.2061961887705));
#56351=CARTESIAN_POINT('Ctrl Pts',(5.13873193725801,0.529582954402255,85.3649569510164));
#56352=CARTESIAN_POINT('Ctrl Pts',(2.34489518331184,4.6077777382683,85.5237177132623));
#56353=CARTESIAN_POINT('Ctrl Pts',(-2.60449736313211,4.46265913321349,85.6824784755082));
#56354=CARTESIAN_POINT('Ctrl Pts',(-4.72633661207834,0.94905134843793,85.8147791107131));
#56355=CARTESIAN_POINT('Ctrl Pts',(-4.08944266318188,-1.99447502555823,
85.9206196188771));
#56356=CARTESIAN_POINT('Ctrl Pts',(-3.130164636136,-3.13763950664809,85.973539872959));
#56357=CARTESIAN_POINT('Ctrl Pts',(-2.53835875722777,-3.5596515025498,86.));
#56358=CARTESIAN_POINT('Ctrl Pts',(-2.00237954638818,4.09906332620103,25.7806068977079));
#56359=CARTESIAN_POINT('Ctrl Pts',(-2.68386473467845,3.76615995447791,25.8070670247489));
#56360=CARTESIAN_POINT('Ctrl Pts',(-3.86722056834447,2.75399327045732,25.8599872788309));
#56361=CARTESIAN_POINT('Ctrl Pts',(-5.02742207131257,-0.166516440447624,
25.9658277869948));
#56362=CARTESIAN_POINT('Ctrl Pts',(-3.44586235178049,-4.14677665817345,
26.0981284221997));
#56363=CARTESIAN_POINT('Ctrl Pts',(1.62355296838563,-5.14470657330929,26.2568891844456));
#56364=CARTESIAN_POINT('Ctrl Pts',(5.19838240423087,-1.42611203276403,26.4156499466915));
#56365=CARTESIAN_POINT('Ctrl Pts',(4.01994424953236,3.59365933878956,26.5744107089374));
#56366=CARTESIAN_POINT('Ctrl Pts',(-0.839985566934964,5.3265048273725,26.7331714711833));
#56367=CARTESIAN_POINT('Ctrl Pts',(-4.92992667194028,2.18327469128225,26.8919322334291));
#56368=CARTESIAN_POINT('Ctrl Pts',(-4.50847904072441,-2.95758319158922,
27.050692995675));
#56369=CARTESIAN_POINT('Ctrl Pts',(0.0395956222711487,-5.39186919347605,
27.2094537579209));
#56370=CARTESIAN_POINT('Ctrl Pts',(4.55125923496193,-2.89119591637671,27.3682145201668));
#56371=CARTESIAN_POINT('Ctrl Pts',(4.89756113932563,2.25550678246132,27.5269752824127));
#56372=CARTESIAN_POINT('Ctrl Pts',(0.761418625289898,5.33794327443822,27.6857360446586));
#56373=CARTESIAN_POINT('Ctrl Pts',(-4.07157300373756,3.53490884489523,27.8444968069045));
#56374=CARTESIAN_POINT('Ctrl Pts',(-5.17814942709716,-1.503370550728,28.0032575691504));
#56375=CARTESIAN_POINT('Ctrl Pts',(-1.54551865619794,-5.1657253452884,28.1620183313962));
#56376=CARTESIAN_POINT('Ctrl Pts',(3.50161451494142,-4.10024735702302,28.3207790936422));
#56377=CARTESIAN_POINT('Ctrl Pts',(5.34396494196453,0.717900607442646,28.479539855888));
#56378=CARTESIAN_POINT('Ctrl Pts',(2.29535447129834,4.8790048681726,28.6383006181339));
#56379=CARTESIAN_POINT('Ctrl Pts',(-2.85403402839988,4.57469439300441,28.7970613803798));
#56380=CARTESIAN_POINT('Ctrl Pts',(-5.391323666464,0.0834841081329312,28.9558221426257));
#56381=CARTESIAN_POINT('Ctrl Pts',(-2.99430906975439,-4.48413350506007,
29.1145829048716));
#56382=CARTESIAN_POINT('Ctrl Pts',(2.14318857941972,-4.94773510082165,29.2733436671175));
#56383=CARTESIAN_POINT('Ctrl Pts',(5.31917461298845,-0.88301843516797,29.4321044293634));
#56384=CARTESIAN_POINT('Ctrl Pts',(3.62688954521853,3.98986369193538,29.5908651916093));
#56385=CARTESIAN_POINT('Ctrl Pts',(-1.3848356090803,5.21110068710349,29.7496259538552));
#56386=CARTESIAN_POINT('Ctrl Pts',(-5.12911691883564,1.66297916304394,29.9083867161011));
#56387=CARTESIAN_POINT('Ctrl Pts',(-4.17907375081987,-3.40715168987467,
30.0671474783469));
#56388=CARTESIAN_POINT('Ctrl Pts',(0.595785363987352,-5.35895324212101,
30.2259082405928));
#56389=CARTESIAN_POINT('Ctrl Pts',(4.82536351591838,-2.40607709649645,30.3846690028387));
#56390=CARTESIAN_POINT('Ctrl Pts',(4.63862158504372,2.74891430277669,30.5434297650846));
#56391=CARTESIAN_POINT('Ctrl Pts',(0.206471491199163,5.38801536528353,30.7021905273305));
#56392=CARTESIAN_POINT('Ctrl Pts',(-4.41464761825083,3.09584018650688,30.8609512895764));
#56393=CARTESIAN_POINT('Ctrl Pts',(-4.99534638025495,-2.02974249468088,
31.0197120518223));
#56394=CARTESIAN_POINT('Ctrl Pts',(-1.00415155023673,-5.29764284541871,
31.1784728140681));
#56395=CARTESIAN_POINT('Ctrl Pts',(3.90607345078174,-3.71697864543531,31.3372335763141));
#56396=CARTESIAN_POINT('Ctrl Pts',(5.24134071706976,1.26557794744869,31.4959943385599));
#56397=CARTESIAN_POINT('Ctrl Pts',(1.77957286026287,5.08983894524214,31.6547551008058));
#56398=CARTESIAN_POINT('Ctrl Pts',(-3.31091443601954,4.25572386919705,31.8135158630518));
#56399=CARTESIAN_POINT('Ctrl Pts',(-5.37115170725749,-0.473359684716424,
31.9722766252976));
#56400=CARTESIAN_POINT('Ctrl Pts',(-2.51554687204882,-4.76920999621703,
32.1310373875435));
#56401=CARTESIAN_POINT('Ctrl Pts',(2.6423632988389,-4.70013364176394,32.2897981497894));
#56402=CARTESIAN_POINT('Ctrl Pts',(5.38190186659124,-0.329351410916935,
32.4485589120353));
#56403=CARTESIAN_POINT('Ctrl Pts',(3.19575945370633,4.34286329137105,32.6073196742812));
#56404=CARTESIAN_POINT('Ctrl Pts',(-1.91523962695419,5.04035685490976,32.7660804365271));
#56405=CARTESIAN_POINT('Ctrl Pts',(-5.27335289927007,1.12476186513028,32.9248411987729));
#56406=CARTESIAN_POINT('Ctrl Pts',(-3.80513252151237,-3.82024953991496,
33.0836019610189));
#56407=CARTESIAN_POINT('Ctrl Pts',(1.14566136921973,-5.26885187498842,33.2423627232647));
#56408=CARTESIAN_POINT('Ctrl Pts',(5.04791098015974,-1.89524003489642,33.4011234855106));
#56409=CARTESIAN_POINT('Ctrl Pts',(4.330158271609,3.21295337599341,33.5598842477565));
#56410=CARTESIAN_POINT('Ctrl Pts',(-0.350687553524876,5.38055371623537,
33.7186450100024));
#56411=CARTESIAN_POINT('Ctrl Pts',(-4.71057341778202,2.62370694422547,33.8774057722483));
#56412=CARTESIAN_POINT('Ctrl Pts',(-4.75919860374648,-2.53443656531169,
34.0361665344942));
#56413=CARTESIAN_POINT('Ctrl Pts',(-0.452059855948003,-5.3729863149027,
34.19492729674));
#56414=CARTESIAN_POINT('Ctrl Pts',(4.2688178803622,-3.29401486909083,34.353688058986));
#56415=CARTESIAN_POINT('Ctrl Pts',(5.08274309982495,1.79973960190727,34.5124488212318));
#56416=CARTESIAN_POINT('Ctrl Pts',(1.2447865799184,5.24631741547787,34.6712095834778));
#56417=CARTESIAN_POINT('Ctrl Pts',(-3.73243664043062,3.89130527955111,34.8299703457236));
#56418=CARTESIAN_POINT('Ctrl Pts',(-5.2936198386959,-1.02514830968824,34.9887311079695));
#56419=CARTESIAN_POINT('Ctrl Pts',(-2.00992046486332,-5.00335485233809,
35.1474918702154));
#56420=CARTESIAN_POINT('Ctrl Pts',(3.11331951223216,-4.40233820466419,35.3062526324613));
#56421=CARTESIAN_POINT('Ctrl Pts',(5.38715437415002,0.227832839089729,35.4650133947072));
#56422=CARTESIAN_POINT('Ctrl Pts',(2.73050100007286,4.64948430926405,35.6237741569531));
#56423=CARTESIAN_POINT('Ctrl Pts',(-2.42519029351004,4.81578571925249,35.782534919199));
#56424=CARTESIAN_POINT('Ctrl Pts',(-5.36127335207045,0.574532938890892,
35.9412956814449));
#56425=CARTESIAN_POINT('Ctrl Pts',(-3.39055527658917,-4.19254993648074,
36.1000564436907));
#56426=CARTESIAN_POINT('Ctrl Pts',(1.68330255388594,-5.12248304687996,36.2588172059367));
#56427=CARTESIAN_POINT('Ctrl Pts',(5.21655046989866,-1.36416320449261,36.4175779681825));
#56428=CARTESIAN_POINT('Ctrl Pts',(3.97545205425126,3.64268047155399,36.5763387304284));
#56429=CARTESIAN_POINT('Ctrl Pts',(-0.904101513210989,5.31563171291061,
36.7350994926743));
#56430=CARTESIAN_POINT('Ctrl Pts',(-4.95619375964226,2.12355444252664,36.8938602549202));
#56431=CARTESIAN_POINT('Ctrl Pts',(-4.47222608833935,-3.01206471847277,
37.0526210171661));
#56432=CARTESIAN_POINT('Ctrl Pts',(0.10485950493631,-5.39095024441108,37.211381779412));
#56433=CARTESIAN_POINT('Ctrl Pts',(4.58597447631896,-2.83587343794507,37.3701425416579));
#56434=CARTESIAN_POINT('Ctrl Pts',(4.8698655265602,2.31468136181031,37.5289033039037));
#56435=CARTESIAN_POINT('Ctrl Pts',(0.696706894914159,5.34676907637412,37.6876640661497));
#56436=CARTESIAN_POINT('Ctrl Pts',(-4.1140991681465,3.48533041305234,37.8464248283955));
#56437=CARTESIAN_POINT('Ctrl Pts',(-5.15955600572413,-1.56598910509857,
38.0051855906414));
#56438=CARTESIAN_POINT('Ctrl Pts',(-1.48282958617279,-5.18406756050325,
38.1639463528873));
#56439=CARTESIAN_POINT('Ctrl Pts',(3.55102776426338,-4.05752903512989,38.3227071151332));
#56440=CARTESIAN_POINT('Ctrl Pts',(5.33487603729029,0.782584002032494,38.4814678773791));
#56441=CARTESIAN_POINT('Ctrl Pts',(2.23608280507879,4.90645225619513,38.640228639625));
#56442=CARTESIAN_POINT('Ctrl Pts',(-2.90924171237944,4.53978553595244,38.7989894018709));
#56443=CARTESIAN_POINT('Ctrl Pts',(-5.39193935072285,0.0181684236512802,
38.9577501641167));
#56444=CARTESIAN_POINT('Ctrl Pts',(-2.93976939635272,-4.52007698493724,
39.1165109263627));
#56445=CARTESIAN_POINT('Ctrl Pts',(2.20296730598482,-4.92140986936197,39.2752716886085));
#56446=CARTESIAN_POINT('Ctrl Pts',(5.32948103937253,-0.818518114924823,
39.4340324508545));
#56447=CARTESIAN_POINT('Ctrl Pts',(3.5782909344085,4.03350642025291,39.5927932131003));
#56448=CARTESIAN_POINT('Ctrl Pts',(-1.44786033404595,5.19394267455733,39.7515539753462));
#56449=CARTESIAN_POINT('Ctrl Pts',(-5.14888559931178,1.60072394206216,39.9103147375921));
#56450=CARTESIAN_POINT('Ctrl Pts',(-4.13749348932905,-3.45752623695775,
40.069075499838));
#56451=CARTESIAN_POINT('Ctrl Pts',(0.660659043471872,-5.3513427923999,40.2278362620838));
#56452=CARTESIAN_POINT('Ctrl Pts',(4.85415623959407,-2.3474469653437,40.3865970243298));
#56453=CARTESIAN_POINT('Ctrl Pts',(4.60498137310684,2.80490402809622,40.5453577865757));
#56454=CARTESIAN_POINT('Ctrl Pts',(0.141186892964701,5.39012117811339,40.7041185488216));
#56455=CARTESIAN_POINT('Ctrl Pts',(-4.45182614422856,3.04213478252601,40.8628793110674));
#56456=CARTESIAN_POINT('Ctrl Pts',(-4.97039191142365,-2.09010628924604,
41.0216400733134));
#56457=CARTESIAN_POINT('Ctrl Pts',(-0.939903178686041,-5.30941824197221,
41.1804008355592));
#56458=CARTESIAN_POINT('Ctrl Pts',(3.95081365290143,-3.66938844135355,41.3391615978052));
#56459=CARTESIAN_POINT('Ctrl Pts',(5.22562515017917,1.32897774372121,41.497922360051));
#56460=CARTESIAN_POINT('Ctrl Pts',(1.71778489121437,5.11102290358859,41.6566831222969));
#56461=CARTESIAN_POINT('Ctrl Pts',(-3.36222457061253,4.21530378386431,41.8154438845428));
#56462=CARTESIAN_POINT('Ctrl Pts',(-5.36502340492809,-0.538390116983158,
41.9742046467887));
#56463=CARTESIAN_POINT('Ctrl Pts',(-2.4575889422798,-4.7993329374274,42.1329654090346));
#56464=CARTESIAN_POINT('Ctrl Pts',(2.69910598837468,-4.66777965600471,42.2917261712804));
#56465=CARTESIAN_POINT('Ctrl Pts',(5.38549667320271,-0.26413185422043,42.4504869335264));
#56466=CARTESIAN_POINT('Ctrl Pts',(3.14291630057783,4.38125748855891,42.6092476957722));
#56467=CARTESIAN_POINT('Ctrl Pts',(-1.97615707196429,5.01678615055665,42.7680084580181));
#56468=CARTESIAN_POINT('Ctrl Pts',(-5.28659112974097,1.06079888783667,42.926769220264));
#56469=CARTESIAN_POINT('Ctrl Pts',(-3.75857550455005,-3.86606391955536,
43.0855299825098));
#56470=CARTESIAN_POINT('Ctrl Pts',(1.20940322958872,-5.25458693731027,43.2442907447559));
#56471=CARTESIAN_POINT('Ctrl Pts',(5.07049918630525,-1.83395148659098,43.4030515070016));
#56472=CARTESIAN_POINT('Ctrl Pts',(4.29091940730092,3.26517238343396,43.5618122692476));
#56473=CARTESIAN_POINT('Ctrl Pts',(-0.41584088110511,5.37591075215103,43.7205730314935));
#56474=CARTESIAN_POINT('Ctrl Pts',(-4.74201089309862,2.56645139116746,43.8793337937394));
#56475=CARTESIAN_POINT('Ctrl Pts',(-4.72814768911957,-2.59190267629106,
44.0380945559852));
#56476=CARTESIAN_POINT('Ctrl Pts',(-0.386939296906612,-5.3780682437099,
44.1968553182311));
#56477=CARTESIAN_POINT('Ctrl Pts',(4.30840775904998,-3.24206147925195,44.3556160804771));
#56478=CARTESIAN_POINT('Ctrl Pts',(5.06056843189549,1.86117898107469,44.5143768427229));
#56479=CARTESIAN_POINT('Ctrl Pts',(1.18114229879479,5.26101158746959,44.6731376049688));
#56480=CARTESIAN_POINT('Ctrl Pts',(-3.77930134462421,3.84580568932092,44.8318983672147));
#56481=CARTESIAN_POINT('Ctrl Pts',(-5.2808129571804,-1.08919904735859,44.9906591294605));
#56482=CARTESIAN_POINT('Ctrl Pts',(-1.94916324679306,-5.02733554587743,
45.1494198917065));
#56483=CARTESIAN_POINT('Ctrl Pts',(3.16642020502591,-4.36430099084551,45.3081806539524));
#56484=CARTESIAN_POINT('Ctrl Pts',(5.38399916564066,0.293075140317788,45.4669414161982));
#56485=CARTESIAN_POINT('Ctrl Pts',(2.67397763346517,4.68221995096551,45.6257021784443));
#56486=CARTESIAN_POINT('Ctrl Pts',(-2.48334990656791,4.78605404221895,45.7844629406899));
#56487=CARTESIAN_POINT('Ctrl Pts',(-5.3678397571995,0.509545282109415,45.9432237029359));
#56488=CARTESIAN_POINT('Ctrl Pts',(-3.3395186992418,-4.23331488444999,46.1019844651818));
#56489=CARTESIAN_POINT('Ctrl Pts',(1.74523187918884,-5.10171596047391,46.2607452274276));
#56490=CARTESIAN_POINT('Ctrl Pts',(5.232692932984,-1.30087075552908,46.4195059896737));
#56491=CARTESIAN_POINT('Ctrl Pts',(3.93103357982541,3.69057110049061,46.5782667519194));
#56492=CARTESIAN_POINT('Ctrl Pts',(-0.96842778057353,5.30428955537918,46.7370275141654));
#56493=CARTESIAN_POINT('Ctrl Pts',(-4.98155445517987,2.06336018755066,46.8957882764112));
#56494=CARTESIAN_POINT('Ctrl Pts',(-4.43541032884349,-3.06601945008181,
47.0545490386572));
#56495=CARTESIAN_POINT('Ctrl Pts',(0.170156811823045,-5.3892844342159,47.213309800903));
#56496=CARTESIAN_POINT('Ctrl Pts',(4.61999124080161,-2.78011168631907,47.3720705631489));
#56497=CARTESIAN_POINT('Ctrl Pts',(4.8414685667286,2.37350419651411,47.5308313253948));
#56498=CARTESIAN_POINT('Ctrl Pts',(0.631885975802691,5.35481653906792,47.6895920876407));
#56499=CARTESIAN_POINT('Ctrl Pts',(-4.15601796138632,3.43523722006585,47.8483528498866));
#56500=CARTESIAN_POINT('Ctrl Pts',(-5.14020731309298,-1.62837613342762,
48.0071136121325));
#56501=CARTESIAN_POINT('Ctrl Pts',(-1.41992192218023,-5.20164991021152,
48.1658743743783));
#56502=CARTESIAN_POINT('Ctrl Pts',(3.59991938399174,-4.01421480270452,48.3246351366243));
#56503=CARTESIAN_POINT('Ctrl Pts',(5.32500450896511,0.847152308025391,48.4833958988701));
#56504=CARTESIAN_POINT('Ctrl Pts',(2.17648285295299,4.93317974984624,48.642156661116));
#56505=CARTESIAN_POINT('Ctrl Pts',(-2.96402239161607,4.50421039867032,48.800917423362));
#56506=CARTESIAN_POINT('Ctrl Pts',(-5.39176380613531,-0.0471498922667038,
48.9596781856078));
#56507=CARTESIAN_POINT('Ctrl Pts',(-2.88479829170963,-4.55535716158905,
49.1184389478537));
#56508=CARTESIAN_POINT('Ctrl Pts',(2.26242273659985,-4.89436241142882,49.2771997100995));
#56509=CARTESIAN_POINT('Ctrl Pts',(5.33900536977086,-0.753897682082513,
49.4359604723455));
#56510=CARTESIAN_POINT('Ctrl Pts',(3.52916720648512,4.07655723401027,49.5947212345913));
#56511=CARTESIAN_POINT('Ctrl Pts',(-1.51067258399179,5.1760224494748,49.7534819968373));
#56512=CARTESIAN_POINT('Ctrl Pts',(-5.16789868150448,1.53823381551562,49.9122427590831));
#56513=CARTESIAN_POINT('Ctrl Pts',(-4.09530605018365,-3.5073933923671,50.0710035213291));
#56514=CARTESIAN_POINT('Ctrl Pts',(0.72543577101732,-5.34294703282935,50.2297642835748));
#56515=CARTESIAN_POINT('Ctrl Pts',(4.88223661585912,-2.28847234640404,50.3885250458209));
#56516=CARTESIAN_POINT('Ctrl Pts',(4.57066538000743,2.86048213374822,50.5472858080667));
#56517=CARTESIAN_POINT('Ctrl Pts',(0.0758815755810925,5.39143599052969,
50.7060465703126));
#56518=CARTESIAN_POINT('Ctrl Pts',(-4.48835136464999,2.98798294522175,50.8648073325585));
#56519=CARTESIAN_POINT('Ctrl Pts',(-4.94470803747584,-2.15016336068061,
51.0235680948044));
#56520=CARTESIAN_POINT('Ctrl Pts',(-0.875516876330153,-5.32041448129303,
51.1823288570502));
#56521=CARTESIAN_POINT('Ctrl Pts',(3.99497407304406,-3.62125975444968,51.3410896192962));
#56522=CARTESIAN_POINT('Ctrl Pts',(5.20914272269644,1.39218251248544,51.499850381542));
#56523=CARTESIAN_POINT('Ctrl Pts',(1.65574483720076,5.13145681922537,51.658611143788));
#56524=CARTESIAN_POINT('Ctrl Pts',(-3.41304129868565,4.17426510262078,51.8173719060338));
#56525=CARTESIAN_POINT('Ctrl Pts',(-5.35810778531101,-0.603341540490118,
51.9761326682797));
#56526=CARTESIAN_POINT('Ctrl Pts',(-2.39927036128639,-4.82875157643711,
52.1348934305256));
#56527=CARTESIAN_POINT('Ctrl Pts',(2.75545258405494,-4.6347406734915,52.2936541927715));
#56528=CARTESIAN_POINT('Ctrl Pts',(5.38830115807414,-0.198873536169234,
52.4524149550174));
#56529=CARTESIAN_POINT('Ctrl Pts',(3.08961192442195,4.41900873612634,52.6111757172633));
#56530=CARTESIAN_POINT('Ctrl Pts',(-2.03678451588621,4.99247923273975,52.7699364795092));
#56531=CARTESIAN_POINT('Ctrl Pts',(-5.29905355286222,0.996680238285941,
52.928697241755));
#56532=CARTESIAN_POINT('Ctrl Pts',(-3.71146691656038,-3.91131095424147,
53.087458004001));
#56533=CARTESIAN_POINT('Ctrl Pts',(1.27296761001063,-5.23955088889833,53.2462187662468));
#56534=CARTESIAN_POINT('Ctrl Pts',(5.09234329659795,-1.77239380586966,53.4049795284928));
#56535=CARTESIAN_POINT('Ctrl Pts',(4.25105085048754,3.31691222676463,53.5637402907385));
#56536=CARTESIAN_POINT('Ctrl Pts',(-0.48093318402806,5.37047887306077,53.7225010529846));
#56537=CARTESIAN_POINT('Ctrl Pts',(-4.77275247822576,2.50881921131856,53.8812618152303));
#56538=CARTESIAN_POINT('Ctrl Pts',(-4.69640291872861,-2.64898842550301,
54.0400225774763));
#56539=CARTESIAN_POINT('Ctrl Pts',(-0.321761954516003,-5.38236094089921,
54.1987833397221));
#56540=CARTESIAN_POINT('Ctrl Pts',(4.34736537881655,-3.18963231682882,54.3575441019682));
#56541=CARTESIAN_POINT('Ctrl Pts',(5.03765112545161,1.92234523219103,54.5163048642139));
#56542=CARTESIAN_POINT('Ctrl Pts',(1.11732468501616,5.27493370590994,54.6750656264599));
#56543=CARTESIAN_POINT('Ctrl Pts',(-3.82561143627296,3.79974172703212,54.8338263887057));
#56544=CARTESIAN_POINT('Ctrl Pts',(-5.26723111626224,-1.15308994504782,
54.9925871509516));
#56545=CARTESIAN_POINT('Ctrl Pts',(-1.88811998897897,-5.05057847782898,
55.1513479131975));
#56546=CARTESIAN_POINT('Ctrl Pts',(3.21905622559384,-4.32562331577277,55.3101086754434));
#56547=CARTESIAN_POINT('Ctrl Pts',(5.38005385515049,0.358274432763269,55.4688694376893));
#56548=CARTESIAN_POINT('Ctrl Pts',(2.61706186058861,4.71426847679935,55.6276301999351));
#56549=CARTESIAN_POINT('Ctrl Pts',(-2.54114508797937,4.75562001166302,55.7863909621812));
#56550=CARTESIAN_POINT('Ctrl Pts',(-5.37361843174121,0.444482849548049,
55.9451517244269));
#56551=CARTESIAN_POINT('Ctrl Pts',(-3.28799204746135,-4.27345859337873,
56.1039124866729));
#56552=CARTESIAN_POINT('Ctrl Pts',(1.80690509167997,-5.08020019715291,56.2626732489186));
#56553=CARTESIAN_POINT('Ctrl Pts',(5.24806749828111,-1.23738740375719,56.4214340111647));
#56554=CARTESIAN_POINT('Ctrl Pts',(3.88603822614634,3.73792013804749,56.5801947734104));
#56555=CARTESIAN_POINT('Ctrl Pts',(-1.03261193114073,5.2921689932538,56.7389555356565));
#56556=CARTESIAN_POINT('Ctrl Pts',(-5.00618410750568,2.00286313442759,56.8977162979023));
#56557=CARTESIAN_POINT('Ctrl Pts',(-4.3979436727968,-3.11952424327782,57.0564770601482));
#56558=CARTESIAN_POINT('Ctrl Pts',(0.235429148194338,-5.38682774642662,
57.2152378223941));
#56559=CARTESIAN_POINT('Ctrl Pts',(4.65333002148106,-2.72394195324985,57.37399858464));
#56560=CARTESIAN_POINT('Ctrl Pts',(4.81236112129208,2.43197871943155,57.5327593468858));
#56561=CARTESIAN_POINT('Ctrl Pts',(0.566972327412124,5.36207818233195,57.6915201091318));
#56562=CARTESIAN_POINT('Ctrl Pts',(-4.19732685891063,3.38463990595143,57.8502808713776));
#56563=CARTESIAN_POINT('Ctrl Pts',(-5.12010429494008,-1.6905241975279,58.0090416336235));
#56564=CARTESIAN_POINT('Ctrl Pts',(-1.35680588461835,-5.21846891769574,
58.1678023958695));
#56565=CARTESIAN_POINT('Ctrl Pts',(3.64828271548151,-3.97031148417985,58.3265631581153));
#56566=CARTESIAN_POINT('Ctrl Pts',(5.31435153612611,0.911596294400786,58.4853239203612));
#56567=CARTESIAN_POINT('Ctrl Pts',(2.11656350192684,4.95918329927446,58.6440846826071));
#56568=CARTESIAN_POINT('Ctrl Pts',(-3.01836810050987,4.46797426842589,58.8028454448529));
#56569=CARTESIAN_POINT('Ctrl Pts',(-5.39079702010585,-0.112461288937121,
58.9616062070989));
#56570=CARTESIAN_POINT('Ctrl Pts',(-2.8294038428619,-4.58996883949007,59.1203669693448));
#56571=CARTESIAN_POINT('Ctrl Pts',(2.32154615663493,-4.86659670571795,59.2791277315906));
#56572=CARTESIAN_POINT('Ctrl Pts',(5.34774620102881,-0.689166614740877,
59.4378884938366));
#56573=CARTESIAN_POINT('Ctrl Pts',(3.47952557320649,4.11900981291542,59.5966492560824));
#56574=CARTESIAN_POINT('Ctrl Pts',(-1.5732631427069,5.15734264299855,59.7554100183284));
#56575=CARTESIAN_POINT('Ctrl Pts',(-5.18615337446655,1.47551795312722,59.9141707805741));
#56576=CARTESIAN_POINT('Ctrl Pts',(-4.05251762479693,-3.55674583772888,
60.0729315428202));
#56577=CARTESIAN_POINT('Ctrl Pts',(0.790106040849496,-5.33376719567931,
60.2316923050659));
#56578=CARTESIAN_POINT('Ctrl Pts',(4.90960052380718,-2.22916189410365,60.3904530673119));
#56579=CARTESIAN_POINT('Ctrl Pts',(4.53567864167587,2.91564046359228,60.5492138295578));
#56580=CARTESIAN_POINT('Ctrl Pts',(0.0105651225747838,5.39195960961101,
60.7079745918036));
#56581=CARTESIAN_POINT('Ctrl Pts',(-4.52421791942263,2.93339262136295,60.8667353540496));
#56582=CARTESIAN_POINT('Ctrl Pts',(-4.91829852752871,-2.20990489560075,
61.0254961162954));
#56583=CARTESIAN_POINT('Ctrl Pts',(-0.811002091855911,-5.3306299496867,
61.1842568785414));
#56584=CARTESIAN_POINT('Ctrl Pts',(4.03854823066489,-3.57259964760746,61.3430176407872));
#56585=CARTESIAN_POINT('Ctrl Pts',(5.19189585341926,1.4551829784393,61.5017784030331));
#56586=CARTESIAN_POINT('Ctrl Pts',(1.5934618026005,5.15113769347555,61.660539165279));
#56587=CARTESIAN_POINT('Ctrl Pts',(-3.4633571628827,4.1326138478934,61.8192999275249));
#56588=CARTESIAN_POINT('Ctrl Pts',(-5.35040586327371,-0.668204423614378,
61.9780606897707));
#56589=CARTESIAN_POINT('Ctrl Pts',(-2.34059968732153,-4.85746159606041,
62.1368214520167));
#56590=CARTESIAN_POINT('Ctrl Pts',(2.81139481701569,-4.60102154269558,62.2955822142625));
#56591=CARTESIAN_POINT('Ctrl Pts',(5.39031490964729,-0.133586033422769,
62.4543429765085));
#56592=CARTESIAN_POINT('Ctrl Pts',(3.03585414765692,4.45611149407704,62.6131037387543));
#56593=CARTESIAN_POINT('Ctrl Pts',(-2.09711306164141,4.96743966849971,62.7718645010003));
#56594=CARTESIAN_POINT('Ctrl Pts',(-5.310738339773,0.932415325891086,62.930625263246));
#56595=CARTESIAN_POINT('Ctrl Pts',(-3.66381367072956,-3.95598400396999,
63.089386025492));
#56596=CARTESIAN_POINT('Ctrl Pts',(1.33634518241131,-5.223745936293,63.2481467877379));
#56597=CARTESIAN_POINT('Ctrl Pts',(5.11344010541426,-1.71057602632341,63.4069075499838));
#56598=CARTESIAN_POINT('Ctrl Pts',(4.21055845188033,3.36816531316245,63.5656683122297));
#56599=CARTESIAN_POINT('Ctrl Pts',(-0.545954909997053,5.36425887609291,
63.7244290744756));
#56600=CARTESIAN_POINT('Ctrl Pts',(-4.80279366183524,2.45081886220229,63.8831898367214));
#56601=CARTESIAN_POINT('Ctrl Pts',(-4.66396895111927,-2.70568543561274,
64.0419505989674));
#56602=CARTESIAN_POINT('Ctrl Pts',(-0.256537393552353,-5.38586377651727,
64.2007113612132));
#56603=CARTESIAN_POINT('Ctrl Pts',(4.38568502263036,-3.13673507580205,64.3594721234591));
#56604=CARTESIAN_POINT('Ctrl Pts',(5.01399454360851,1.98322937910761,64.5182328857051));
#56605=CARTESIAN_POINT('Ctrl Pts',(1.05334310381863,5.28808172772786,64.6769936479507));
#56606=CARTESIAN_POINT('Ctrl Pts',(-3.87136011937014,3.75312015257198,64.8357544101969));
#56607=CARTESIAN_POINT('Ctrl Pts',(-5.25287630907674,-1.21681162676554,
64.9945151724425));
#56608=CARTESIAN_POINT('Ctrl Pts',(-1.82679964952023,-5.07308023729216,
65.1532759346887));
#56609=CARTESIAN_POINT('Ctrl Pts',(3.27121984959904,-4.28631085539543,65.3120366969344));
#56610=CARTESIAN_POINT('Ctrl Pts',(5.3753190216539,0.423421148429019,65.4707974591804));
#56611=CARTESIAN_POINT('Ctrl Pts',(2.55976203383379,4.7456251836438,65.6295582214262));
#56612=CARTESIAN_POINT('Ctrl Pts',(-2.59856735630046,4.7244880937792,65.7883189836722));
#56613=CARTESIAN_POINT('Ctrl Pts',(-5.37860852767513,0.379355189119878,
65.947079745918));
#56614=CARTESIAN_POINT('Ctrl Pts',(-3.23598288278473,-4.31297517217702,
66.1058405081639));
#56615=CARTESIAN_POINT('Ctrl Pts',(1.86831314081432,-5.05793891435551,66.2646012704098));
#56616=CARTESIAN_POINT('Ctrl Pts',(5.26267190957225,-1.17372246536004,66.4233620326557));
#56617=CARTESIAN_POINT('Ctrl Pts',(3.84047259628301,3.78472063575253,66.5821227949015));
#56618=CARTESIAN_POINT('Ctrl Pts',(-1.09664454588739,5.27927180522719,66.7408835571475));
#56619=CARTESIAN_POINT('Ctrl Pts',(-5.03007910221774,1.94207216110101,66.8996443193933));
#56620=CARTESIAN_POINT('Ctrl Pts',(-4.35983161843177,-3.17257124623133,
67.0584050816393));
#56621=CARTESIAN_POINT('Ctrl Pts',(0.300666935333765,-5.38358054156236,
67.2171658438851));
#56622=CARTESIAN_POINT('Ctrl Pts',(4.68598592589077,-2.66737248164657,67.375926606131));
#56623=CARTESIAN_POINT('Ctrl Pts',(4.78254746176859,2.49009634942548,67.534687368377));
#56624=CARTESIAN_POINT('Ctrl Pts',(0.50197547582154,5.3685529405199,67.6934481306227));
#56625=CARTESIAN_POINT('Ctrl Pts',(-4.23801979863793,3.33354589586587,67.8522088928688));
#56626=CARTESIAN_POINT('Ctrl Pts',(-5.09924990138375,-1.75242417716988,
68.0109696551145));
#56627=CARTESIAN_POINT('Ctrl Pts',(-1.29349073576672,-5.2345221147663,68.1697304173606));
#56628=CARTESIAN_POINT('Ctrl Pts',(3.69611066141296,-3.92582552236859,68.3284911796063));
#56629=CARTESIAN_POINT('Ctrl Pts',(5.30291868209728,0.975906504002708,68.4872519418522));
#56630=CARTESIAN_POINT('Ctrl Pts',(2.05633354516605,4.98445908845845,68.6460127040982));
#56631=CARTESIAN_POINT('Ctrl Pts',(-3.07227086382722,4.43108246287181,68.804773466344));
#56632=CARTESIAN_POINT('Ctrl Pts',(-5.38903913451035,-0.177756181911403,
68.96353422859));
#56633=CARTESIAN_POINT('Ctrl Pts',(-2.77359417894579,-4.62390693937597,
69.1222949908358));
#56634=CARTESIAN_POINT('Ctrl Pts',(2.38032888972716,-4.83811682684714,69.2810557530817));
#56635=CARTESIAN_POINT('Ctrl Pts',(5.35570225042921,-0.624334412185203,
69.4398165153275));
#56636=CARTESIAN_POINT('Ctrl Pts',(3.42937331948324,4.16085792705156,69.5985772775736));
#56637=CARTESIAN_POINT('Ctrl Pts',(-1.63562282502583,5.13790599639058,69.7573380398193));
#56638=CARTESIAN_POINT('Ctrl Pts',(-5.20364699932156,1.4125855584507,69.9160988020653));
#56639=CARTESIAN_POINT('Ctrl Pts',(-4.00913449237088,-3.60557633057093,
70.0748595643111));
#56640=CARTESIAN_POINT('Ctrl Pts',(0.854660362605124,-5.32380462809097,
70.233620326557));
#56641=CARTESIAN_POINT('Ctrl Pts',(4.93624394778424,-2.1695243122525,70.392381088803));
#56642=CARTESIAN_POINT('Ctrl Pts',(4.50002629241666,2.97037092314251,70.5511418510488));
#56643=CARTESIAN_POINT('Ctrl Pts',(-0.0547528808636342,5.39169195851627,
70.7099026132947));
#56644=CARTESIAN_POINT('Ctrl Pts',(-4.55942054512895,2.87837182208054,70.8686633755406));
#56645=CARTESIAN_POINT('Ctrl Pts',(-4.89116725717831,-2.26932212693528,
71.0274241377865));
#56646=CARTESIAN_POINT('Ctrl Pts',(-0.746368292808977,-5.34006314803305,
71.1861849000323));
#56647=CARTESIAN_POINT('Ctrl Pts',(4.08152973125557,-3.52341526169831,71.3449456622782));
#56648=CARTESIAN_POINT('Ctrl Pts',(5.17388707332602,1.51796989626334,71.5037064245242));
#56649=CARTESIAN_POINT('Ctrl Pts',(1.53094492744998,5.1700626381705,71.66246718677));
#56650=CARTESIAN_POINT('Ctrl Pts',(-3.51316477934987,4.09035613200449,71.8212279490159));
#56651=CARTESIAN_POINT('Ctrl Pts',(-5.34191876907334,-0.732969247726808,
71.9799887112618));
#56652=CARTESIAN_POINT('Ctrl Pts',(-2.28158553030752,-4.88545878310146,
72.1387494735077));
#56653=CARTESIAN_POINT('Ctrl Pts',(2.86692447773331,-4.56662721189998,72.2975102357536));
#56654=CARTESIAN_POINT('Ctrl Pts',(5.39153763240408,-0.0682789269231456,
72.4562709979995));
#56655=CARTESIAN_POINT('Ctrl Pts',(2.98165085923738,4.49256031758063,72.6150317602455));
#56656=CARTESIAN_POINT('Ctrl Pts',(-2.15713385601469,4.94167113239301,72.7737925224911));
#56657=CARTESIAN_POINT('Ctrl Pts',(-5.32164377573057,0.868013581529248,
72.9325532847373));
#56658=CARTESIAN_POINT('Ctrl Pts',(-3.61562276017225,-4.00007651297025,
73.091314046983));
#56659=CARTESIAN_POINT('Ctrl Pts',(1.39952664613108,-5.20717439887132,73.250074809229));
#56660=CARTESIAN_POINT('Ctrl Pts',(5.13378651679711,-1.64850721971224,73.4088355714748));
#56661=CARTESIAN_POINT('Ctrl Pts',(4.16944815373948,3.41892412123604,73.5675963337207));
#56662=CARTESIAN_POINT('Ctrl Pts',(-0.610896517072584,5.35725167403211,
73.7263570959665));
#56663=CARTESIAN_POINT('Ctrl Pts',(-4.83213003538284,2.39245885537094,73.8851178582126));
#56664=CARTESIAN_POINT('Ctrl Pts',(-4.63085054597687,-2.76198538633308,
74.0438786204583));
#56665=CARTESIAN_POINT('Ctrl Pts',(-0.191275185721079,-5.38857623652284,
74.2026393827044));
#56666=CARTESIAN_POINT('Ctrl Pts',(4.42336106708315,-3.08337751884262,74.3614001449501));
#56667=CARTESIAN_POINT('Ctrl Pts',(4.98960215796993,2.04382248707493,74.5201609071961));
#56668=CARTESIAN_POINT('Ctrl Pts',(0.989206944500219,5.30045372345089,74.678921669442));
#56669=CARTESIAN_POINT('Ctrl Pts',(-3.9165406802957,3.70594780765739,74.8376824316877));
#56670=CARTESIAN_POINT('Ctrl Pts',(-5.23775064219211,-1.2803547413539,74.9964431939339));
#56671=CARTESIAN_POINT('Ctrl Pts',(-1.76521122717783,-5.09483752213321,
75.1552039561795));
#56672=CARTESIAN_POINT('Ctrl Pts',(3.32290342202856,-4.24636937881787,75.3139647184255));
#56673=CARTESIAN_POINT('Ctrl Pts',(5.36979535998785,0.488505727033064,75.4727254806714));
#56674=CARTESIAN_POINT('Ctrl Pts',(2.50208656195135,4.77628546990172,75.6314862429173));
#56675=CARTESIAN_POINT('Ctrl Pts',(-2.65560828481232,4.69266285717694,75.7902470051632));
#56676=CARTESIAN_POINT('Ctrl Pts',(-5.38280931270438,0.314171858310403,
75.9490077674091));
#56677=CARTESIAN_POINT('Ctrl Pts',(-3.18349883755812,-4.35185882178607,
76.107768529655));
#56678=CARTESIAN_POINT('Ctrl Pts',(1.92944701495941,-5.03493537892548,76.2665292919008));
#56679=CARTESIAN_POINT('Ctrl Pts',(5.27650402365974,-1.10988528316864,76.4252900541468));
#56680=CARTESIAN_POINT('Ctrl Pts',(3.7943433769926,3.83096572563162,76.5840508163925));
#56681=CARTESIAN_POINT('Ctrl Pts',(-1.16051622802576,5.26559988396195,76.7428115786386));
#56682=CARTESIAN_POINT('Ctrl Pts',(-5.0532359327251,1.88099618864767,76.9015723408843));
#56683=CARTESIAN_POINT('Ctrl Pts',(-4.32107975869319,-3.22515267429361,
77.0603331031303));
#56684=CARTESIAN_POINT('Ctrl Pts',(0.365860599594574,-5.37954329615034,
77.2190938653761));
#56685=CARTESIAN_POINT('Ctrl Pts',(4.7179541617759,-2.61041157308061,77.3778546276221));
#56686=CARTESIAN_POINT('Ctrl Pts',(4.75203196331349,2.54784855773221,77.5366153898679));
#56687=CARTESIAN_POINT('Ctrl Pts',(0.436904959320356,5.37423986346092,77.6953761521139));
#56688=CARTESIAN_POINT('Ctrl Pts',(-4.27809080887851,3.28196268785622,77.8541369143598));
#56689=CARTESIAN_POINT('Ctrl Pts',(-5.07764719280662,-1.81406698853016,
78.0128976766055));
#56690=CARTESIAN_POINT('Ctrl Pts',(-1.22998576712498,-5.24980714561609,
78.1716584388517));
#56691=CARTESIAN_POINT('Ctrl Pts',(3.74339620303386,-3.88076344558682,78.3304192010973));
#56692=CARTESIAN_POINT('Ctrl Pts',(5.29070762465021,1.0400734993063,78.4891799633433));
#56693=CARTESIAN_POINT('Ctrl Pts',(1.99580182141817,5.00900340817564,78.6479407255891));
#56694=CARTESIAN_POINT('Ctrl Pts',(-3.12572277133616,4.39354039588141,78.8067014878351));
#56695=CARTESIAN_POINT('Ctrl Pts',(-5.38649040731852,-0.243024989162281,
78.965462250081));
#56696=CARTESIAN_POINT('Ctrl Pts',(-2.71737749003105,-4.65716648082978,
79.1242230123268));
#56697=CARTESIAN_POINT('Ctrl Pts',(2.43876230950906,-4.8089269542393,79.2829837745728));
#56698=CARTESIAN_POINT('Ctrl Pts',(5.36287235042167,-0.559410588542699,
79.4417445368186));
#56699=CARTESIAN_POINT('Ctrl Pts',(3.37871780515969,4.20209543520715,79.6005052990646));
#56700=CARTESIAN_POINT('Ctrl Pts',(-1.69774247966381,5.11771536197905,79.7592660613104));
#56701=CARTESIAN_POINT('Ctrl Pts',(-5.2203769888794,1.34944586681667,79.9180268235563));
#56702=CARTESIAN_POINT('Ctrl Pts',(-3.96516301938171,-3.65387770501744,
80.0767875858022));
#56703=CARTESIAN_POINT('Ctrl Pts',(0.91908926293675,-5.31306079207099,80.235548348048));
#56704=CARTESIAN_POINT('Ctrl Pts',(4.96216297786599,-2.10956835266785,80.3943091102941));
#56705=CARTESIAN_POINT('Ctrl Pts',(4.46371356421533,3.02466548070436,80.5530698725397));
#56706=CARTESIAN_POINT('Ctrl Pts',(-0.120062849320441,5.39063307652007,
80.7118306347859));
#56707=CARTESIAN_POINT('Ctrl Pts',(-4.59395407577343,2.82292862168424,80.8705913970315));
#56708=CARTESIAN_POINT('Ctrl Pts',(-4.86331820795707,-2.32840633521552,
81.0293521592777));
#56709=CARTESIAN_POINT('Ctrl Pts',(-0.681624964166643,-5.34871269198804,
81.1881129215234));
#56710=CARTESIAN_POINT('Ctrl Pts',(4.12391226721417,-3.47371381457424,81.3468736837694));
#56711=CARTESIAN_POINT('Ctrl Pts',(5.15511902533117,1.58053405205645,81.5056344460152));
#56712=CARTESIAN_POINT('Ctrl Pts',(1.46820338586184,5.18822887591951,81.6643952082611));
#56713=CARTESIAN_POINT('Ctrl Pts',(-3.56245683835765,4.04749815657105,81.823155970507));
#56714=CARTESIAN_POINT('Ctrl Pts',(-5.33264774907332,-0.797626509155247,
81.9819167327528));
#56715=CARTESIAN_POINT('Ctrl Pts',(-2.22223654888384,-4.91273902788576,
82.1406774949988));
#56716=CARTESIAN_POINT('Ctrl Pts',(2.92203341399256,-4.53156273055457,82.2994382572446));
#56717=CARTESIAN_POINT('Ctrl Pts',(5.39196915310808,-0.0029617965042665,
82.4581990194906));
#56718=CARTESIAN_POINT('Ctrl Pts',(2.92701000162586,4.52834985013744,82.6169597817364));
#56719=CARTESIAN_POINT('Ctrl Pts',(-2.21683806821556,4.91517742057454,82.7757205439824));
#56720=CARTESIAN_POINT('Ctrl Pts',(-5.33176830391211,0.803484428152502,
82.9344813062282));
#56721=CARTESIAN_POINT('Ctrl Pts',(-3.56690117349271,-4.04358195702611,
83.0932420684741));
#56722=CARTESIAN_POINT('Ctrl Pts',(1.46250256952503,-5.18983881124397,83.2520028307201));
#56723=CARTESIAN_POINT('Ctrl Pts',(5.15337985091046,-1.58619629785924,83.4107635929658));
#56724=CARTESIAN_POINT('Ctrl Pts',(4.12772540290961,3.46918082523772,83.5695243552118));
#56725=CARTESIAN_POINT('Ctrl Pts',(-0.675747352509778,5.34945901705833,
83.7282851174576));
#56726=CARTESIAN_POINT('Ctrl Pts',(-4.86075944383677,2.33374637252957,83.8870458797035));
#56727=CARTESIAN_POINT('Ctrl Pts',(-4.59704844530487,-2.81787736745293,
84.0458066419496));
#56728=CARTESIAN_POINT('Ctrl Pts',(-0.125992795831606,-5.39050299503273,
84.2045674041953));
#56729=CARTESIAN_POINT('Ctrl Pts',(4.46040309055735,-3.02955776127604,84.3633281664412));
#56730=CARTESIAN_POINT('Ctrl Pts',(4.96444861251837,2.10409705678322,84.5220889286871));
#56731=CARTESIAN_POINT('Ctrl Pts',(0.924981040394022,5.31208351664113,84.6808496909329));
#56732=CARTESIAN_POINT('Ctrl Pts',(-3.96125263942776,3.65816335371309,84.8396104531789));
#56733=CARTESIAN_POINT('Ctrl Pts',(-5.22165301904991,-1.3435792187099,84.9983712154247));
#56734=CARTESIAN_POINT('Ctrl Pts',(-1.70375320028204,-5.11609758128303,
85.1571319776708));
#56735=CARTESIAN_POINT('Ctrl Pts',(3.37484546343723,-4.20532487574203,85.3158927399164));
#56736=CARTESIAN_POINT('Ctrl Pts',(5.36205285859353,0.552597767150946,85.4746535021625));
#56737=CARTESIAN_POINT('Ctrl Pts',(2.4468005092104,4.80802425479881,85.6334142644084));
#56738=CARTESIAN_POINT('Ctrl Pts',(-2.7176845769921,4.65659903150035,85.7921750266542));
#56739=CARTESIAN_POINT('Ctrl Pts',(-4.93173550418608,0.99029557446776,85.9244756618591));
#56740=CARTESIAN_POINT('Ctrl Pts',(-4.26716318148111,-2.08115166207624,
86.0303161700231));
#56741=CARTESIAN_POINT('Ctrl Pts',(-3.26619649360748,-3.2739962098191,86.083236424105));
#56742=CARTESIAN_POINT('Ctrl Pts',(-2.64867169498456,-3.71434815979703,
86.109696551146));
#56743=CARTESIAN_POINT('Ctrl Pts',(-2.08577545033697,4.2697827545171,25.890303448854));
#56744=CARTESIAN_POINT('Ctrl Pts',(-2.79564340622372,3.92301449006545,25.9167635758949));
#56745=CARTESIAN_POINT('Ctrl Pts',(-4.02828411678504,2.86869268329956,25.9696838299769));
#56746=CARTESIAN_POINT('Ctrl Pts',(-5.2368061558258,-0.173451583736938,
26.0755243381408));
#56747=CARTESIAN_POINT('Ctrl Pts',(-3.58937700474797,-4.31948327041665,
26.2078249733457));
#56748=CARTESIAN_POINT('Ctrl Pts',(1.69117135154962,-5.35897536965486,26.3665857355916));
#56749=CARTESIAN_POINT('Ctrl Pts',(5.4148867130437,-1.48550731689914,26.5253464978375));
#56750=CARTESIAN_POINT('Ctrl Pts',(4.18736849490951,3.74332949976516,26.6841072600834));
#56751=CARTESIAN_POINT('Ctrl Pts',(-0.874969621673782,5.54834523009075,
26.8428680223293));
#56752=CARTESIAN_POINT('Ctrl Pts',(-5.13525022907948,2.27420458855161,27.0016287845751));
#56753=CARTESIAN_POINT('Ctrl Pts',(-4.6962499784134,-3.08076179886732,27.1603895468211));
#56754=CARTESIAN_POINT('Ctrl Pts',(0.0412447165789918,-5.61643191744809,
27.319150309067));
#56755=CARTESIAN_POINT('Ctrl Pts',(4.7408118992853,-3.01160959987317,27.4779110713129));
#56756=CARTESIAN_POINT('Ctrl Pts',(5.1015367238218,2.34944503074463,27.6366718335587));
#56757=CARTESIAN_POINT('Ctrl Pts',(0.793130492629709,5.56026007017329,27.7954325958046));
#56758=CARTESIAN_POINT('Ctrl Pts',(-4.24114750411255,3.68213214181093,27.9541933580505));
#56759=CARTESIAN_POINT('Ctrl Pts',(-5.39381106478857,-1.56598352850948,
28.1129541202964));
#56760=CARTESIAN_POINT('Ctrl Pts',(-1.60988703512753,-5.3808695398533,28.2717148825423));
#56761=CARTESIAN_POINT('Ctrl Pts',(3.6474511562916,-4.2710160983281,28.4304756447882));
#56762=CARTESIAN_POINT('Ctrl Pts',(5.5665325305163,0.747800018975952,28.5892364070341));
#56763=CARTESIAN_POINT('Ctrl Pts',(2.39095231205807,5.08220761366869,28.74799716928));
#56764=CARTESIAN_POINT('Ctrl Pts',(-2.97289997872796,4.76522309415968,28.9067579315259));
#56765=CARTESIAN_POINT('Ctrl Pts',(-5.61586367010893,0.0869610876472672,
29.0655186937718));
#56766=CARTESIAN_POINT('Ctrl Pts',(-3.11901725108991,-4.67089049014597,
29.2242794560176));
#56767=CARTESIAN_POINT('Ctrl Pts',(2.23244895427517,-5.15380035052699,29.3830402182635));
#56768=CARTESIAN_POINT('Ctrl Pts',(5.54070972400729,-0.91979474000819,29.5418009805094));
#56769=CARTESIAN_POINT('Ctrl Pts',(3.77794369111745,4.15603513022305,29.7005617427553));
#56770=CARTESIAN_POINT('Ctrl Pts',(-1.44251179621886,5.42813469204637,29.8593225050012));
#56771=CARTESIAN_POINT('Ctrl Pts',(-5.34273643101869,1.73223958412626,30.0180832672471));
#56772=CARTESIAN_POINT('Ctrl Pts',(-4.35312548529055,-3.54905410571791,
30.176844029493));
#56773=CARTESIAN_POINT('Ctrl Pts',(0.620598871036556,-5.58214506939038,
30.3356047917389));
#56774=CARTESIAN_POINT('Ctrl Pts',(5.02633218492865,-2.50628635742007,30.4943655539847));
#56775=CARTESIAN_POINT('Ctrl Pts',(4.83181275145273,2.86340218474256,30.6531263162307));
#56776=CARTESIAN_POINT('Ctrl Pts',(0.215070698416827,5.61241758347815,30.8118870784765));
#56777=CARTESIAN_POINT('Ctrl Pts',(-4.59851062734073,3.22477697638755,30.9706478407224));
#56778=CARTESIAN_POINT('Ctrl Pts',(-5.2033945635623,-2.11427802164059,31.1294086029683));
#56779=CARTESIAN_POINT('Ctrl Pts',(-1.04597285548533,-5.51828119277288,
31.2881693652142));
#56780=CARTESIAN_POINT('Ctrl Pts',(4.06875515960443,-3.87178485819991,31.4469301274601));
#56781=CARTESIAN_POINT('Ctrl Pts',(5.4596341708714,1.31828724381346,31.605690889706));
#56782=CARTESIAN_POINT('Ctrl Pts',(1.853689222264,5.30182259267667,31.7644516519519));
#56783=CARTESIAN_POINT('Ctrl Pts',(-3.4488087242362,4.43296795844451,31.9232124141977));
#56784=CARTESIAN_POINT('Ctrl Pts',(-5.59485158108012,-0.493074358126545,
32.0819731764437));
#56785=CARTESIAN_POINT('Ctrl Pts',(-2.62031537395337,-4.96783996098723,
32.2407339386895));
#56786=CARTESIAN_POINT('Ctrl Pts',(2.75241350199106,-4.89588668690527,32.3994947009355));
#56787=CARTESIAN_POINT('Ctrl Pts',(5.60604946734801,-0.343068370161422,
32.5582554631813));
#56788=CARTESIAN_POINT('Ctrl Pts',(3.3288577211775,4.52373659811392,32.7170162254272));
#56789=CARTESIAN_POINT('Ctrl Pts',(-1.99500629269775,5.25027965246184,32.8757769876731));
#56790=CARTESIAN_POINT('Ctrl Pts',(-5.49297960923532,1.17160639699654,33.034537749919));
#56791=CARTESIAN_POINT('Ctrl Pts',(-3.96361020215392,-3.97935682018335,
33.1932985121649));
#56792=CARTESIAN_POINT('Ctrl Pts',(1.19337633198882,-5.48829112449471,33.3520592744107));
#56793=CARTESIAN_POINT('Ctrl Pts',(5.25814839494067,-1.97417374963327,33.5108200366567));
#56794=CARTESIAN_POINT('Ctrl Pts',(4.51050243460883,3.34676774281486,33.6695807989025));
#56795=CARTESIAN_POINT('Ctrl Pts',(-0.365293128967798,5.60464516868708,
33.8283415611484));
#56796=CARTESIAN_POINT('Ctrl Pts',(-4.9067612628892,2.73298014006108,33.9871023233943));
#56797=CARTESIAN_POINT('Ctrl Pts',(-4.95741161004009,-2.63999179271414,
34.1458630856402));
#56798=CARTESIAN_POINT('Ctrl Pts',(-0.470887425572999,-5.59676259719809,
34.3046238478861));
#56799=CARTESIAN_POINT('Ctrl Pts',(4.4466073142222,-3.43120531738688,34.463384610132));
#56800=CARTESIAN_POINT('Ctrl Pts',(5.29443121665232,1.87469587642792,34.6221453723779));
#56801=CARTESIAN_POINT('Ctrl Pts',(1.296629949095,5.4648181408047,34.7809061346238));
#56802=CARTESIAN_POINT('Ctrl Pts',(-3.88788665395154,4.05337191767345,34.9396668968696));
#56803=CARTESIAN_POINT('Ctrl Pts',(-5.51409063425751,-1.06784409636987,
35.0984276591156));
#56804=CARTESIAN_POINT('Ctrl Pts',(-2.09363043599948,-5.21173657569289,
35.2571884213614));
#56805=CARTESIAN_POINT('Ctrl Pts',(3.2429842880596,-4.58568854637521,35.4159491836074));
#56806=CARTESIAN_POINT('Ctrl Pts',(5.61152073344166,0.237321712265504,35.5747099458532));
#56807=CARTESIAN_POINT('Ctrl Pts',(2.8442219974453,4.84312789075476,35.7334707080991));
#56808=CARTESIAN_POINT('Ctrl Pts',(-2.52619558850515,5.01635548835761,35.892231470345));
#56809=CARTESIAN_POINT('Ctrl Pts',(-5.58456180820669,0.598461316442061,
36.0509922325909));
#56810=CARTESIAN_POINT('Ctrl Pts',(-3.53176647837594,-4.36716293252018,
36.2097529948368));
#56811=CARTESIAN_POINT('Ctrl Pts',(1.7534094116762,-5.33582626891128,36.3685137570827));
#56812=CARTESIAN_POINT('Ctrl Pts',(5.43381144957445,-1.4209784190592,36.5272745193285));
#56813=CARTESIAN_POINT('Ctrl Pts',(4.14102327089027,3.79439228426682,36.6860352815745));
#56814=CARTESIAN_POINT('Ctrl Pts',(-0.941755894515449,5.5370192678104,36.8447960438203));
#56815=CARTESIAN_POINT('Ctrl Pts',(-5.16261129895229,2.2119970869982,37.0035568060662));
#56816=CARTESIAN_POINT('Ctrl Pts',(-4.65848714857258,-3.13751239416556,
37.1623175683121));
#56817=CARTESIAN_POINT('Ctrl Pts',(0.109226735523501,-5.61547469562505,
37.321078330558));
#56818=CARTESIAN_POINT('Ctrl Pts',(4.77697297489437,-2.95398302874052,37.4798390928039));
#56819=CARTESIAN_POINT('Ctrl Pts',(5.07268763310252,2.4110841366338,37.6385998550498));
#56820=CARTESIAN_POINT('Ctrl Pts',(0.725723622233936,5.56945345263699,37.7973606172957));
#56821=CARTESIAN_POINT('Ctrl Pts',(-4.2854448152198,3.63048884761598,37.9561213795416));
#56822=CARTESIAN_POINT('Ctrl Pts',(-5.37444325716809,-1.63121004546892,
38.1148821417874));
#56823=CARTESIAN_POINT('Ctrl Pts',(-1.54458706564933,-5.39997567898108,
38.2736429040334));
#56824=CARTESIAN_POINT('Ctrl Pts',(3.69892238837796,-4.22651862668493,38.4324036662792));
#56825=CARTESIAN_POINT('Ctrl Pts',(5.55706508750621,0.815177373445694,38.5911644285252));
#56826=CARTESIAN_POINT('Ctrl Pts',(2.32921207578554,5.11079814148172,38.749925190771));
#56827=CARTESIAN_POINT('Ctrl Pts',(-3.0304069744033,4.7288603390718,38.908685953017));
#56828=CARTESIAN_POINT('Ctrl Pts',(-5.61650499663195,0.0189251094235045,
39.0674467152627));
#56829=CARTESIAN_POINT('Ctrl Pts',(-3.0622060875641,-4.70833095844415,39.2262074775087));
#56830=CARTESIAN_POINT('Ctrl Pts',(2.29471736914525,-5.126378715302,39.3849682397545));
#56831=CARTESIAN_POINT('Ctrl Pts',(5.55144539655818,-0.852608084638733,
39.5437290020005));
#56832=CARTESIAN_POINT('Ctrl Pts',(3.72732102593349,4.20149550833897,39.7024897642464));
#56833=CARTESIAN_POINT('Ctrl Pts',(-1.50816140012871,5.41026207573349,39.8612505264922));
#56834=CARTESIAN_POINT('Ctrl Pts',(-5.3633284454033,1.66739153280986,40.0200112887382));
#56835=CARTESIAN_POINT('Ctrl Pts',(-4.30981347244434,-3.60152667207889,
40.178772050984));
#56836=CARTESIAN_POINT('Ctrl Pts',(0.688174435462339,-5.57421765661644,
40.3375328132299));
#56837=CARTESIAN_POINT('Ctrl Pts',(5.05632407947203,-2.4452143751233,40.4962935754758));
#56838=CARTESIAN_POINT('Ctrl Pts',(4.79677147851891,2.92172379252827,40.6550543377217));
#56839=CARTESIAN_POINT('Ctrl Pts',(0.147067101132706,5.61461110004271,40.8138150999676));
#56840=CARTESIAN_POINT('Ctrl Pts',(-4.63723757943327,3.16883482826894,40.9725758622135));
#56841=CARTESIAN_POINT('Ctrl Pts',(-5.1774007810357,-2.17715587165673,41.1313366244594));
#56842=CARTESIAN_POINT('Ctrl Pts',(-0.979048642068222,-5.53054701575012,
41.2900973867053));
#56843=CARTESIAN_POINT('Ctrl Pts',(4.11535871955024,-3.82221259827082,41.4488581489512));
#56844=CARTESIAN_POINT('Ctrl Pts',(5.44326407576748,1.38432754014994,41.607618911197));
#56845=CARTESIAN_POINT('Ctrl Pts',(1.7893278831762,5.32388882899019,41.7663796734429));
#56846=CARTESIAN_POINT('Ctrl Pts',(-3.50225584382976,4.39086444123689,41.9251404356888));
#56847=CARTESIAN_POINT('Ctrl Pts',(-5.58846804476507,-0.560813203837097,
42.0839011979347));
#56848=CARTESIAN_POINT('Ctrl Pts',(-2.55994358915231,-4.99921747449702,
42.2426619601806));
#56849=CARTESIAN_POINT('Ctrl Pts',(2.81151943374774,-4.86218520941121,42.4014227224265));
#56850=CARTESIAN_POINT('Ctrl Pts',(5.60979399190252,-0.275132523291236,
42.5601834846724));
#56851=CARTESIAN_POINT('Ctrl Pts',(3.27381373527952,4.56372985217721,42.7189442469183));
#56852=CARTESIAN_POINT('Ctrl Pts',(-2.05846085181392,5.22572726598967,42.8777050091642));
#56853=CARTESIAN_POINT('Ctrl Pts',(-5.50676919082185,1.10497946405063,43.03646577141));
#56854=CARTESIAN_POINT('Ctrl Pts',(-3.91511415993451,-4.02707929542473,
43.1952265336559));
#56855=CARTESIAN_POINT('Ctrl Pts',(1.25977293884402,-5.47343207498865,43.3539872959018));
#56856=CARTESIAN_POINT('Ctrl Pts',(5.28167736372706,-1.91033263136333,43.5127480581477));
#56857=CARTESIAN_POINT('Ctrl Pts',(4.46962933439137,3.40116158835573,43.6715088203935));
#56858=CARTESIAN_POINT('Ctrl Pts',(-0.433159988384986,5.59980883257818,
43.8302695826396));
#56859=CARTESIAN_POINT('Ctrl Pts',(-4.93950805874728,2.67333998483713,43.9890303448854));
#56860=CARTESIAN_POINT('Ctrl Pts',(-4.92506747450587,-2.69985127525994,
44.1477911071313));
#56861=CARTESIAN_POINT('Ctrl Pts',(-0.403054699451855,-5.60205618020814,
44.3065518693771));
#56862=CARTESIAN_POINT('Ctrl Pts',(4.48784604800658,-3.37708815199574,44.4653126316231));
#56863=CARTESIAN_POINT('Ctrl Pts',(5.27133300928694,1.93869410742388,44.6240733938689));
#56864=CARTESIAN_POINT('Ctrl Pts',(1.2303349855046,5.48012430154663,44.7828341561148));
#56865=CARTESIAN_POINT('Ctrl Pts',(-3.93670319808305,4.00597734231749,44.9415949183607));
#56866=CARTESIAN_POINT('Ctrl Pts',(-5.50075036662014,-1.13456244477178,
45.1003556806066));
#56867=CARTESIAN_POINT('Ctrl Pts',(-2.03034277701881,-5.23671602674481,
45.2591164428525));
#56868=CARTESIAN_POINT('Ctrl Pts',(3.2982965397378,-4.5460671434672,45.4178772050984));
#56869=CARTESIAN_POINT('Ctrl Pts',(5.60823411554676,0.305281250940591,45.5766379673442));
#56870=CARTESIAN_POINT('Ctrl Pts',(2.78534452306571,4.87722691955032,45.7353987295903));
#56871=CARTESIAN_POINT('Ctrl Pts',(-2.5867774563813,4.98538553455152,45.894159491836));
#56872=CARTESIAN_POINT('Ctrl Pts',(-5.59140169360195,0.53076702774728,46.052920254082));
#56873=CARTESIAN_POINT('Ctrl Pts',(-3.47860430924953,-4.40962567534128,
46.2116810163279));
#56874=CARTESIAN_POINT('Ctrl Pts',(1.81791799428017,-5.3141942665874,46.3704417785737));
#56875=CARTESIAN_POINT('Ctrl Pts',(5.45062622041652,-1.35504994087535,46.5292025408197));
#56876=CARTESIAN_POINT('Ctrl Pts',(4.09475483808194,3.84427748126524,46.6879633030655));
#56877=CARTESIAN_POINT('Ctrl Pts',(-1.00876124798033,5.52520472756723,46.8467240653114));
#56878=CARTESIAN_POINT('Ctrl Pts',(-5.18902822687748,2.14929583762384,47.0054848275573));
#56879=CARTESIAN_POINT('Ctrl Pts',(-4.62013807160538,-3.19371425400909,
47.1642455898032));
#56880=CARTESIAN_POINT('Ctrl Pts',(0.177243570754919,-5.61373950710082,
47.3230063520491));
#56881=CARTESIAN_POINT('Ctrl Pts',(4.81240648318495,-2.89589888938787,47.4817671142949));
#56882=CARTESIAN_POINT('Ctrl Pts',(5.04310798533405,2.47235684827615,47.6405278765409));
#56883=CARTESIAN_POINT('Ctrl Pts',(0.658203015566318,5.57783607927463,47.7992886387866));
#56884=CARTESIAN_POINT('Ctrl Pts',(-4.32910945912064,3.57830935329949,47.9580494010327));
#56885=CARTESIAN_POINT('Ctrl Pts',(-5.35428872245015,-1.69619539369769,
48.1168101632785));
#56886=CARTESIAN_POINT('Ctrl Pts',(-1.47905939811478,-5.41829030541985,
48.2755709255244));
#56887=CARTESIAN_POINT('Ctrl Pts',(3.74985026583283,-4.18140042578941,48.4343316877703));
#56888=CARTESIAN_POINT('Ctrl Pts',(5.54678242582246,0.882434846062579,48.5930924500162));
#56889=CARTESIAN_POINT('Ctrl Pts',(2.26712988102407,5.13863879247473,48.7518532122621));
#56890=CARTESIAN_POINT('Ctrl Pts',(-3.08746918127143,4.69180355424833,48.9106139745079));
#56891=CARTESIAN_POINT('Ctrl Pts',(-5.61632214089325,-0.0491136098317049,
49.0693747367539));
#56892=CARTESIAN_POINT('Ctrl Pts',(-3.00494552437603,-4.74508049799904,
49.2281354989997));
#56893=CARTESIAN_POINT('Ctrl Pts',(2.35664902330628,-5.09820477402661,49.3868962612456));
#56894=CARTESIAN_POINT('Ctrl Pts',(5.561366400077,-0.785296314172567,49.5456570234916));
#56895=CARTESIAN_POINT('Ctrl Pts',(3.67615137334867,4.24633931960047,49.7044177857373));
#56896=CARTESIAN_POINT('Ctrl Pts',(-1.57358967977417,5.39159550195178,49.8631785479833));
#56897=CARTESIAN_POINT('Ctrl Pts',(-5.38313339204505,1.60229879248781,50.0219393102291));
#56898=CARTESIAN_POINT('Ctrl Pts',(-4.26586899396583,-3.65347071471485,
50.1807000724751));
#56899=CARTESIAN_POINT('Ctrl Pts',(0.755649010055931,-5.56547222709447,
50.339460834721));
#56900=CARTESIAN_POINT('Ctrl Pts',(5.08557395847498,-2.38378355767454,50.4982215969668));
#56901=CARTESIAN_POINT('Ctrl Pts',(4.76102627921851,2.97961663734597,50.6569823592128));
#56902=CARTESIAN_POINT('Ctrl Pts',(0.0790419217800287,5.61598067229221,
50.8157431214586));
#56903=CARTESIAN_POINT('Ctrl Pts',(-4.6752840168385,3.11242765359339,50.9745038837046));
#56904=CARTESIAN_POINT('Ctrl Pts',(-5.15064721483666,-2.2397142240147,51.1332646459504));
#56905=CARTESIAN_POINT('Ctrl Pts',(-0.911980753248584,-5.54200123084275,
51.2920254081963));
#56906=CARTESIAN_POINT('Ctrl Pts',(4.16135835052739,-3.77207942857173,51.4507861704422));
#56907=CARTESIAN_POINT('Ctrl Pts',(5.42609518155485,1.45016468639448,51.6095469326881));
#56908=CARTESIAN_POINT('Ctrl Pts',(1.72470396018791,5.34517378451539,51.768307694934));
#56909=CARTESIAN_POINT('Ctrl Pts',(-3.55518900731147,4.34811656458864,51.9270684571799));
#56910=CARTESIAN_POINT('Ctrl Pts',(-5.58126440065713,-0.62846975019945,
52.0858292194257));
#56911=CARTESIAN_POINT('Ctrl Pts',(-2.49919613258049,-5.0298613527465,52.2445899816716));
#56912=CARTESIAN_POINT('Ctrl Pts',(2.87021277497366,-4.82777020614449,52.4033507439175));
#56913=CARTESIAN_POINT('Ctrl Pts',(5.61271527908117,-0.207156300717966,
52.5621115061634));
#56914=CARTESIAN_POINT('Ctrl Pts',(3.2182893171531,4.60305337879721,52.7208722684093));
#56915=CARTESIAN_POINT('Ctrl Pts',(-2.12161333176065,5.20040800394102,52.8796330306552));
#56916=CARTESIAN_POINT('Ctrl Pts',(-5.51975065392403,1.03819037534721,53.038393792901));
#56917=CARTESIAN_POINT('Ctrl Pts',(-3.86604357463707,-4.07421079670234,
53.197154555147));
#56918=CARTESIAN_POINT('Ctrl Pts',(1.32598467399636,-5.45776979922066,53.3559153173929));
#56919=CARTESIAN_POINT('Ctrl Pts',(5.30443124625904,-1.84621117174306,53.5146760796387));
#56920=CARTESIAN_POINT('Ctrl Pts',(4.4281003159834,3.4550563133683,53.6734368418847));
#56921=CARTESIAN_POINT('Ctrl Pts',(-0.500963281565584,5.59415072441577,
53.8321976041305));
#56922=CARTESIAN_POINT('Ctrl Pts',(-4.97152998170303,2.61330751691913,53.9909583663765));
#56923=CARTESIAN_POINT('Ctrl Pts',(-4.89200058522532,-2.75931455457936,
54.1497191286223));
#56924=CARTESIAN_POINT('Ctrl Pts',(-0.33516282504586,-5.60652766136632,
54.3084798908682));
#56925=CARTESIAN_POINT('Ctrl Pts',(4.5284261902974,-3.32247539885354,54.4672406531142));
#56926=CARTESIAN_POINT('Ctrl Pts',(5.24746123370139,2.00240783502248,54.6260014153599));
#56927=CARTESIAN_POINT('Ctrl Pts',(1.16385947023147,5.49462625394218,54.7847621776059));
#56928=CARTESIAN_POINT('Ctrl Pts',(-3.9849420309447,3.95799488970978,54.9435229398517));
#56929=CARTESIAN_POINT('Ctrl Pts',(-5.48660286376106,-1.20111429611312,
55.1022837020977));
#56930=CARTESIAN_POINT('Ctrl Pts',(-1.96675716519669,-5.26092698961938,
55.2610444643435));
#56931=CARTESIAN_POINT('Ctrl Pts',(3.35312476633552,-4.50577860511874,55.4198052265895));
#56932=CARTESIAN_POINT('Ctrl Pts',(5.60412448918787,0.373195989586127,55.5785659888352));
#56933=CARTESIAN_POINT('Ctrl Pts',(2.72605829932405,4.91061021520187,55.7373267510813));
#56934=CARTESIAN_POINT('Ctrl Pts',(-2.64697971461612,4.95368397532273,55.8960875133271));
#56935=CARTESIAN_POINT('Ctrl Pts',(-5.59742104069143,0.462994848981032,
56.054848275573));
#56936=CARTESIAN_POINT('Ctrl Pts',(-3.4249316548741,-4.45144130550992,56.2136090378189));
#56937=CARTESIAN_POINT('Ctrl Pts',(1.88215979738361,-5.29178240615308,56.3723698000648));
#56938=CARTESIAN_POINT('Ctrl Pts',(5.46664111175626,-1.28892260908666,56.5311305623107));
#56939=CARTESIAN_POINT('Ctrl Pts',(4.04788549992257,3.8935985304696,56.6898913245566));
#56940=CARTESIAN_POINT('Ctrl Pts',(-1.07561856571275,5.51257936342436,56.8486520868024));
#56941=CARTESIAN_POINT('Ctrl Pts',(-5.21468366481089,2.08627917904408,57.0074128490483));
#56942=CARTESIAN_POINT('Ctrl Pts',(-4.58111098928757,-3.24944743622466,
57.1661736112942));
#56943=CARTESIAN_POINT('Ctrl Pts',(0.245234395488895,-5.61118050219625,
57.3249343735402));
#56944=CARTESIAN_POINT('Ctrl Pts',(4.84713377073179,-2.83738977681774,57.4836951357859));
#56945=CARTESIAN_POINT('Ctrl Pts',(5.01278826137211,2.53326674150361,57.6424558980319));
#56946=CARTESIAN_POINT('Ctrl Pts',(0.590585817593506,5.58540015836071,57.8012166602777));
#56947=CARTESIAN_POINT('Ctrl Pts',(-4.37213880612535,3.52560474201678,57.9599774225237));
#56948=CARTESIAN_POINT('Ctrl Pts',(-5.33334844575954,-1.76093182521995,
58.1187381847696));
#56949=CARTESIAN_POINT('Ctrl Pts',(-1.41331467858517,-5.43580979765242,
58.2774989470154));
#56950=CARTESIAN_POINT('Ctrl Pts',(3.80022785268933,-4.1356686043012,58.4362597092614));
#56951=CARTESIAN_POINT('Ctrl Pts',(5.53568577371134,0.949562821348838,58.5950204715072));
#56952=CARTESIAN_POINT('Ctrl Pts',(2.20471498490915,5.16572534812638,58.7537812337531));
#56953=CARTESIAN_POINT('Ctrl Pts',(-3.144078301978,4.65405824716339,58.9125419959989));
#56954=CARTESIAN_POINT('Ctrl Pts',(-5.61531508977269,-0.117145121663757,
59.071302758245));
#56955=CARTESIAN_POINT('Ctrl Pts',(-2.94724398537462,-4.78113369689988,
59.2300635204908));
#56956=CARTESIAN_POINT('Ctrl Pts',(2.41823483917798,-5.06928267110287,59.3888242827367));
#56957=CARTESIAN_POINT('Ctrl Pts',(5.57047127296998,-0.717869301457213,
59.5475850449825));
#56958=CARTESIAN_POINT('Ctrl Pts',(3.6244422454793,4.29055998048545,59.7063458072285));
#56959=CARTESIAN_POINT('Ctrl Pts',(-1.63878703510391,5.37213771142675,59.8651065694744));
#56960=CARTESIAN_POINT('Ctrl Pts',(-5.40214836375828,1.53697091478732,60.0238673317203));
#56961=CARTESIAN_POINT('Ctrl Pts',(-4.22129849913074,-3.70487861045338,
60.1826280939661));
#56962=CARTESIAN_POINT('Ctrl Pts',(0.823012693142843,-5.55591006441646,
60.3413888562121));
#56963=CARTESIAN_POINT('Ctrl Pts',(5.11407752940203,-2.32200291994295,60.5001496184578));
#56964=CARTESIAN_POINT('Ctrl Pts',(4.72458239922035,3.03707222336503,60.6589103807039));
#56965=CARTESIAN_POINT('Ctrl Pts',(0.0110051430237869,5.61652609927038,
60.8176711429496));
#56966=CARTESIAN_POINT('Ctrl Pts',(-4.71264435622464,3.05556373009997,60.9764319051957));
#56967=CARTESIAN_POINT('Ctrl Pts',(-5.12313779106008,-2.30194389826733,
61.1351926674413));
#56968=CARTESIAN_POINT('Ctrl Pts',(-0.844779031235954,-5.55264215714847,
61.2939534296875));
#56969=CARTESIAN_POINT('Ctrl Pts',(4.20674730208683,-3.72139270614424,61.4527141919332));
#56970=CARTESIAN_POINT('Ctrl Pts',(5.4081300077703,1.51578902094353,61.6114749541792));
#56971=CARTESIAN_POINT('Ctrl Pts',(1.65982693686032,5.36567433568524,61.770235716425));
#56972=CARTESIAN_POINT('Ctrl Pts',(-3.60760044673811,4.30473060175118,61.9289964786709));
#56973=CARTESIAN_POINT('Ctrl Pts',(-5.5732417058914,-0.696034068613847,
62.0877572409168));
#56974=CARTESIAN_POINT('Ctrl Pts',(-2.43808191892836,-5.05976709874605,
62.2465180031627));
#56975=CARTESIAN_POINT('Ctrl Pts',(2.92848491241984,-4.79264672750744,62.4052787654085));
#56976=CARTESIAN_POINT('Ctrl Pts',(5.61481290018499,-0.139149677953565,
62.5640395276545));
#56977=CARTESIAN_POINT('Ctrl Pts',(3.16229261500766,4.64170140724564,62.7228002899003));
#56978=CARTESIAN_POINT('Ctrl Pts',(-2.18445446491029,5.17432558191808,62.8815610521463));
#56979=CARTESIAN_POINT('Ctrl Pts',(-5.53192209351194,0.97124893218624,63.0403218143921));
#56980=CARTESIAN_POINT('Ctrl Pts',(-3.81640564737093,-4.12074440746734,
63.199082576638));
#56981=CARTESIAN_POINT('Ctrl Pts',(1.39200182087229,-5.44130659563001,63.357843338884));
#56982=CARTESIAN_POINT('Ctrl Pts',(5.32640670340396,-1.78181878059799,63.5166041011298));
#56983=CARTESIAN_POINT('Ctrl Pts',(4.38592147376913,3.50844400880067,63.6753648633758));
#56984=CARTESIAN_POINT('Ctrl Pts',(-0.568693058375023,5.58767167452727,
63.8341256256215));
#56985=CARTESIAN_POINT('Ctrl Pts',(-5.00282233253868,2.55289154607289,63.9928863878675));
#56986=CARTESIAN_POINT('Ctrl Pts',(-4.85821579476509,-2.818372904435,64.1516471501133));
#56987=CARTESIAN_POINT('Ctrl Pts',(-0.267221765488804,-5.61017638448271,
64.3104079123593));
#56988=CARTESIAN_POINT('Ctrl Pts',(4.56834178595791,-3.26737507238287,64.4691686746051));
#56989=CARTESIAN_POINT('Ctrl Pts',(5.2228193930792,2.06582770923283,64.6279294368511));
#56990=CARTESIAN_POINT('Ctrl Pts',(1.0972131585588,5.50832186982966,64.7866901990968));
#56991=CARTESIAN_POINT('Ctrl Pts',(-4.03259607348695,3.90943160127608,64.9454509613429));
#56992=CARTESIAN_POINT('Ctrl Pts',(-5.4716502018265,-1.26748988390853,65.1042117235886));
#56993=CARTESIAN_POINT('Ctrl Pts',(-1.90288293172278,-5.28436591135743,
65.2629724858347));
#56994=CARTESIAN_POINT('Ctrl Pts',(3.40746092180959,-4.46482884367352,65.4217332480805));
#56995=CARTESIAN_POINT('Ctrl Pts',(5.59919245745271,0.441055961713188,65.5804940103263));
#56996=CARTESIAN_POINT('Ctrl Pts',(2.66637202647467,4.94327287871016,65.7392547725723));
#56997=CARTESIAN_POINT('Ctrl Pts',(-2.70679352852708,4.92125546287557,65.8980155348181));
#56998=CARTESIAN_POINT('Ctrl Pts',(-5.60261896613596,0.395154725711709,
66.0567762970641));
#56999=CARTESIAN_POINT('Ctrl Pts',(-3.37075639171248,-4.49260368658171,
66.2155370593099));
#57000=CARTESIAN_POINT('Ctrl Pts',(1.94612539350076,-5.26859397654912,66.3742978215559));
#57001=CARTESIAN_POINT('Ctrl Pts',(5.48185377340806,-1.22260612788034,66.5330585838017));
#57002=CARTESIAN_POINT('Ctrl Pts',(4.00042213448843,3.94234819401505,66.6918193460476));
#57003=CARTESIAN_POINT('Ctrl Pts',(-1.1423180364002,5.49914502815419,66.8505801082935));
#57004=CARTESIAN_POINT('Ctrl Pts',(-5.23957384781653,2.02295635895467,67.0093408705393));
#57005=CARTESIAN_POINT('Ctrl Pts',(-4.54141162884421,-3.30470376196668,
67.1681016327853));
#57006=CARTESIAN_POINT('Ctrl Pts',(0.31318923207078,-5.60779805644547,67.3268623950311));
#57007=CARTESIAN_POINT('Ctrl Pts',(4.88114974130499,-2.77846427724327,67.4856231572771));
#57008=CARTESIAN_POINT('Ctrl Pts',(4.98173291063654,2.59380487778839,67.6443839195229));
#57009=CARTESIAN_POINT('Ctrl Pts',(0.522881951140529,5.59214457986643,67.8031446817689));
#57010=CARTESIAN_POINT('Ctrl Pts',(-4.41452654167645,3.47238274817052,67.9619054440147));
#57011=CARTESIAN_POINT('Ctrl Pts',(-5.31162550008227,-1.82540983996319,
68.1206662062607));
#57012=CARTESIAN_POINT('Ctrl Pts',(-1.34736255509922,-5.45253158469304,
68.2794269685065));
#57013=CARTESIAN_POINT('Ctrl Pts',(3.85004775603573,-4.08932987336585,68.4381877307524));
#57014=CARTESIAN_POINT('Ctrl Pts',(5.52377675960678,1.01655144827307,68.5969484929983));
#57015=CARTESIAN_POINT('Ctrl Pts',(2.14197654682777,5.19205383348419,68.7557092552442));
#57016=CARTESIAN_POINT('Ctrl Pts',(-3.20022602913364,4.61562995694134,68.9144700174901));
#57017=CARTESIAN_POINT('Ctrl Pts',(-5.61348399105505,-0.185159442447144,
69.073230779736));
#57018=CARTESIAN_POINT('Ctrl Pts',(-2.88910993826166,-4.81648526433911,
69.2319915419818));
#57019=CARTESIAN_POINT('Ctrl Pts',(2.47946577904082,-5.0396166508499,69.3907523042278));
#57020=CARTESIAN_POINT('Ctrl Pts',(5.57875867909682,-0.650336941407984,
69.5495130664736));
#57021=CARTESIAN_POINT('Ctrl Pts',(3.57220123064088,4.33415100161104,69.7082738287195));
#57022=CARTESIAN_POINT('Ctrl Pts',(-1.70374389840499,5.35189155958961,69.8670345909654));
#57023=CARTESIAN_POINT('Ctrl Pts',(-5.42037057009564,1.47141748657539,70.0257953532113));
#57024=CARTESIAN_POINT('Ctrl Pts',(-4.17610852865976,-3.75574281518495,
70.1845561154572));
#57025=CARTESIAN_POINT('Ctrl Pts',(0.89025559910136,-5.54553257182993,70.343316877703));
#57026=CARTESIAN_POINT('Ctrl Pts',(5.14183060935358,-2.2598815282383,70.5020776399489));
#57027=CARTESIAN_POINT('Ctrl Pts',(4.68744518666451,3.09408211897719,70.6608384021949));
#57028=CARTESIAN_POINT('Ctrl Pts',(-0.0570332507375796,5.61624730093583,
70.8195991644407));
#57029=CARTESIAN_POINT('Ctrl Pts',(-4.74931311496125,2.99825140257037,70.9783599266866));
#57030=CARTESIAN_POINT('Ctrl Pts',(-5.09487654671437,-2.36383576220895,
71.1371206889325));
#57031=CARTESIAN_POINT('Ctrl Pts',(-0.777453337884133,-5.56246823311117,
71.2958814511784));
#57032=CARTESIAN_POINT('Ctrl Pts',(4.25151891339917,-3.67015986926562,71.4546422134243));
#57033=CARTESIAN_POINT('Ctrl Pts',(5.38937119080337,1.58119091342487,71.6134029756702));
#57034=CARTESIAN_POINT('Ctrl Pts',(1.59470633389773,5.38538747404349,71.7721637379161));
#57035=CARTESIAN_POINT('Ctrl Pts',(-3.65948247073021,4.26071291961525,71.9309245001618));
#57036=CARTESIAN_POINT('Ctrl Pts',(-5.56440113779842,-0.763496244015491,
72.089685262408));
#57037=CARTESIAN_POINT('Ctrl Pts',(-2.3766099167077,-5.08893032382693,72.2484460246537));
#57038=CARTESIAN_POINT('Ctrl Pts',(2.98632729464914,-4.75681992787116,72.4072067868998));
#57039=CARTESIAN_POINT('Ctrl Pts',(5.61608654738804,-0.0711226349710497,
72.5659675491454));
#57040=CARTESIAN_POINT('Ctrl Pts',(3.10583184636022,4.67966826592364,72.7247283113916));
#57041=CARTESIAN_POINT('Ctrl Pts',(-2.24697502932542,5.14748382751671,72.8834890736371));
#57042=CARTESIAN_POINT('Ctrl Pts',(-5.54328172342653,0.904164958225804,
73.0422498358833));
#57043=CARTESIAN_POINT('Ctrl Pts',(-3.76620766250282,-4.1666732989117,73.2010105981289));
#57044=CARTESIAN_POINT('Ctrl Pts',(1.45781469145456,-5.42404488019209,73.3597713603751));
#57045=CARTESIAN_POINT('Ctrl Pts',(5.34760051026307,-1.71716490751244,73.5185321226207));
#57046=CARTESIAN_POINT('Ctrl Pts',(4.3430989974944,3.56131684000752,73.6772928848668));
#57047=CARTESIAN_POINT('Ctrl Pts',(-0.636339379467287,5.58037263371339,
73.8360536471125));
#57048=CARTESIAN_POINT('Ctrl Pts',(-5.03338051910119,2.49210093834326,73.9948144093586));
#57049=CARTESIAN_POINT('Ctrl Pts',(-4.82371806104376,-2.87701765801306,
74.1535751716043));
#57050=CARTESIAN_POINT('Ctrl Pts',(-0.199241491132339,-5.61300181410709,
74.3123359338505));
#57051=CARTESIAN_POINT('Ctrl Pts',(4.60758697737389,-3.21179525855753,74.4710966960961));
#57052=CARTESIAN_POINT('Ctrl Pts',(5.19741110361085,2.12894442318739,74.6298574583422));
#57053=CARTESIAN_POINT('Ctrl Pts',(1.0304058308339,5.52120913937719,74.7886182205879));
#57054=CARTESIAN_POINT('Ctrl Pts',(-4.07965833247825,3.86029460367982,74.9473789828338));
#57055=CARTESIAN_POINT('Ctrl Pts',(-5.45589457511983,-1.33367946753936,
75.1061397450798));
#57056=CARTESIAN_POINT('Ctrl Pts',(-1.8387294501421,-5.30702935229665,75.2649005073255));
#57057=CARTESIAN_POINT('Ctrl Pts',(3.46129703232802,-4.42322386850986,75.4236612695716));
#57058=CARTESIAN_POINT('Ctrl Pts',(5.5934387441171,0.508851208869345,75.5824220318174));
#57059=CARTESIAN_POINT('Ctrl Pts',(2.60629446347919,4.97521011682889,75.7411827940634));
#57060=CARTESIAN_POINT('Ctrl Pts',(-2.76621012043596,4.88810475609477,75.8999435563092));
#57061=CARTESIAN_POINT('Ctrl Pts',(-5.60699470713969,0.327256613478776,
76.0587043185551));
#57062=CARTESIAN_POINT('Ctrl Pts',(-3.31608646998587,-4.53310677797631,
76.2174650808009));
#57063=CARTESIAN_POINT('Ctrl Pts',(2.00980539567907,-5.24463238067812,76.3762258430469));
#57064=CARTESIAN_POINT('Ctrl Pts',(5.49626197291347,-1.15611022920134,76.5349866052928));
#57065=CARTESIAN_POINT('Ctrl Pts',(3.95237170702942,3.99051931788734,76.6937473675386));
#57066=CARTESIAN_POINT('Ctrl Pts',(-1.20884987189374,5.48490369324573,76.8525081297847));
#57067=CARTESIAN_POINT('Ctrl Pts',(-5.26369512325953,1.95933666998091,77.0112688920303));
#57068=CARTESIAN_POINT('Ctrl Pts',(-4.50104581615728,-3.35947512236825,
77.1700296542764));
#57069=CARTESIAN_POINT('Ctrl Pts',(0.381098108126755,-5.60359266622235,
77.3287904165222));
#57070=CARTESIAN_POINT('Ctrl Pts',(4.91444940305996,-2.71913103798297,77.4875511787681));
#57071=CARTESIAN_POINT('Ctrl Pts',(4.94994649050095,2.65396237315744,77.646311941014));
#57072=CARTESIAN_POINT('Ctrl Pts',(0.455101351751309,5.59806835404786,77.8050727032599));
#57073=CARTESIAN_POINT('Ctrl Pts',(-4.45626644537291,3.41865118208945,77.9638334655057));
#57074=CARTESIAN_POINT('Ctrl Pts',(-5.28912307326102,-1.88961997577731,
78.1225942277517));
#57075=CARTESIAN_POINT('Ctrl Pts',(-1.28121270613263,-5.468453212619,78.2813549899975));
#57076=CARTESIAN_POINT('Ctrl Pts',(3.89930266479998,-4.04239103319333,78.4401157522435));
#57077=CARTESIAN_POINT('Ctrl Pts',(5.51105713115687,1.08339089625261,78.5988765144893));
#57078=CARTESIAN_POINT('Ctrl Pts',(2.07892377364716,5.21762038484239,78.7576372767352));
#57079=CARTESIAN_POINT('Ctrl Pts',(-3.2559041230579,4.57652432293467,78.9163980389812));
#57080=CARTESIAN_POINT('Ctrl Pts',(-5.61082911345409,-0.253146591078478,
79.0751588012269));
#57081=CARTESIAN_POINT('Ctrl Pts',(-2.83055191421017,-4.85113001247338,
79.2339195634729));
#57082=CARTESIAN_POINT('Ctrl Pts',(2.54033285725292,-5.00921106675685,79.3926803257188));
#57083=CARTESIAN_POINT('Ctrl Pts',(5.58622740228054,-0.582709144400273,
79.5514410879646));
#57084=CARTESIAN_POINT('Ctrl Pts',(3.51943599520346,4.37710598599406,79.7102018502106));
#57085=CARTESIAN_POINT('Ctrl Pts',(-1.7684507372563,5.33086001756339,79.8689626124564));
#57086=CARTESIAN_POINT('Ctrl Pts',(-5.43779733694764,1.40564812781938,80.0277233747023));
#57087=CARTESIAN_POINT('Ctrl Pts',(-4.13030571418267,-3.80605586458648,
80.1864841369483));
#57088=CARTESIAN_POINT('Ctrl Pts',(0.95736786003426,-5.53434127223174,80.345244899194));
#57089=CARTESIAN_POINT('Ctrl Pts',(5.16882912556325,-2.19742849887699,80.5040056614401));
#57090=CARTESIAN_POINT('Ctrl Pts',(4.64962009144032,3.15063795798068,80.6627664236858));
#57091=CARTESIAN_POINT('Ctrl Pts',(-0.125063274873211,5.61514431819889,
80.8215271859319));
#57092=CARTESIAN_POINT('Ctrl Pts',(-4.78528491189737,2.9404990815964,80.9802879481776));
#57093=CARTESIAN_POINT('Ctrl Pts',(-5.06586762915643,-2.42538073321897,
81.1390487104236));
#57094=CARTESIAN_POINT('Ctrl Pts',(-0.710013553204522,-5.5714780167311,
81.2978094726694));
#57095=CARTESIAN_POINT('Ctrl Pts',(4.29566661416096,-3.61838843639986,81.4565702349154));
#57096=CARTESIAN_POINT('Ctrl Pts',(5.36982148364171,1.64636076619313,81.6153309971612));
#57097=CARTESIAN_POINT('Ctrl Pts',(1.52935170749991,5.4043103065256,81.7740917594071));
#57098=CARTESIAN_POINT('Ctrl Pts',(-3.71082746511973,4.21606997808528,81.932852521653));
#57099=CARTESIAN_POINT('Ctrl Pts',(-5.55474399465067,-0.830846376919461,
82.0916132838989));
#57100=CARTESIAN_POINT('Ctrl Pts',(-2.3147891451765,-5.11734674715333,82.2503740461448));
#57101=CARTESIAN_POINT('Ctrl Pts',(3.04373142991963,-4.72029506698704,82.4091348083907));
#57102=CARTESIAN_POINT('Ctrl Pts',(5.61653604023885,-0.00308515058908493,
82.5678955706366));
#57103=CARTESIAN_POINT('Ctrl Pts',(3.04891528446413,4.71694837524191,82.7266563328824));
#57104=CARTESIAN_POINT('Ctrl Pts',(-2.30916582642725,5.11988669499558,82.8854170951283));
#57105=CARTESIAN_POINT('Ctrl Pts',(-5.55382792200581,0.836948268868883,
83.0441778573743));
#57106=CARTESIAN_POINT('Ctrl Pts',(-3.71545689970117,-4.21199067509615,
83.2029386196201));
#57107=CARTESIAN_POINT('Ctrl Pts',(1.52341346128536,-5.40598729308003,83.3616993818661));
#57108=CARTESIAN_POINT('Ctrl Pts',(5.36800987538946,-1.65225883547266,83.5204601441119));
#57109=CARTESIAN_POINT('Ctrl Pts',(4.29963856085619,3.61366665531133,83.6792209063577));
#57110=CARTESIAN_POINT('Ctrl Pts',(-0.703891148427739,5.57225542504627,
83.8379816686037));
#57111=CARTESIAN_POINT('Ctrl Pts',(-5.06320229660515,2.43094317454181,83.9967424308495));
#57112=CARTESIAN_POINT('Ctrl Pts',(-4.78850815696806,-2.93523745070957,
84.1555031930955));
#57113=CARTESIAN_POINT('Ctrl Pts',(-0.131240194167233,-5.61500881902578,
84.3142639553413));
#57114=CARTESIAN_POINT('Ctrl Pts',(4.64617174185204,-3.15573399420934,84.4730247175873));
#57115=CARTESIAN_POINT('Ctrl Pts',(5.17120995324134,2.19172933227414,84.6317854798331));
#57116=CARTESIAN_POINT('Ctrl Pts',(0.963505020594375,5.53332329484411,84.790546242079));
#57117=CARTESIAN_POINT('Ctrl Pts',(-4.12623247316118,3.81052000369223,84.949307004325));
#57118=CARTESIAN_POINT('Ctrl Pts',(-5.43912651173278,-1.39953714320699,
85.1080677665708));
#57119=CARTESIAN_POINT('Ctrl Pts',(-1.77471179476972,-5.32917485889023,
85.2668285288167));
#57120=CARTESIAN_POINT('Ctrl Pts',(3.51540237664497,-4.38046992755931,85.4255892910626));
#57121=CARTESIAN_POINT('Ctrl Pts',(5.58537377992907,0.575612579899635,85.5843500533083));
#57122=CARTESIAN_POINT('Ctrl Pts',(2.54870583510895,5.00827077132932,85.7431108155546));
#57123=CARTESIAN_POINT('Ctrl Pts',(-2.83087179085208,4.8505389297872,85.9018715778));
#57124=CARTESIAN_POINT('Ctrl Pts',(-5.13713439629382,1.0315398004976,86.0341722130053));
#57125=CARTESIAN_POINT('Ctrl Pts',(-4.44488369978034,-2.16782829859426,
86.140012721169));
#57126=CARTESIAN_POINT('Ctrl Pts',(-3.40222835107896,-3.41035291299011,
86.1929329752511));
#57127=CARTESIAN_POINT('Ctrl Pts',(-2.75898463274135,-3.86904481704426,
86.219393102292));
#57128=CARTESIAN_POINT('Ctrl Pts',(-2.16917135428577,4.44050218283316,26.));
#57129=CARTESIAN_POINT('Ctrl Pts',(-2.90742207776898,4.07986902565299,26.026460127041));
#57130=CARTESIAN_POINT('Ctrl Pts',(-4.18934766522561,2.98339209614179,26.0793803811229));
#57131=CARTESIAN_POINT('Ctrl Pts',(-5.44619024033903,-0.180386727026251,
26.1852208892869));
#57132=CARTESIAN_POINT('Ctrl Pts',(-3.73289165771545,-4.49218988265986,
26.3175215244917));
#57133=CARTESIAN_POINT('Ctrl Pts',(1.7587897347136,-5.57324416600043,26.4762822867377));
#57134=CARTESIAN_POINT('Ctrl Pts',(5.63139102185651,-1.54490260103424,26.6350430489835));
#57135=CARTESIAN_POINT('Ctrl Pts',(4.35479274028667,3.89299966074075,26.7938038112295));
#57136=CARTESIAN_POINT('Ctrl Pts',(-0.909953676412603,5.770185632809,26.9525645734753));
#57137=CARTESIAN_POINT('Ctrl Pts',(-5.34057378621867,2.36513448582097,27.1113253357212));
#57138=CARTESIAN_POINT('Ctrl Pts',(-4.88402091610239,-3.20394040614541,
27.2700860979671));
#57139=CARTESIAN_POINT('Ctrl Pts',(0.0428938108868349,-5.84099464142013,
27.428846860213));
#57140=CARTESIAN_POINT('Ctrl Pts',(4.93036456360867,-3.13202328336963,27.5876076224589));
#57141=CARTESIAN_POINT('Ctrl Pts',(5.30551230831797,2.44338327902792,27.7463683847048));
#57142=CARTESIAN_POINT('Ctrl Pts',(0.824842359969521,5.78257686590837,27.9051291469507));
#57143=CARTESIAN_POINT('Ctrl Pts',(-4.41072200448754,3.82935543872663,28.0638899091965));
#57144=CARTESIAN_POINT('Ctrl Pts',(-5.60947270247999,-1.62859650629097,
28.2226506714425));
#57145=CARTESIAN_POINT('Ctrl Pts',(-1.67425541405712,-5.59601373441819,
28.3814114336883));
#57146=CARTESIAN_POINT('Ctrl Pts',(3.79328779764178,-4.44178483963319,28.5401721959342));
#57147=CARTESIAN_POINT('Ctrl Pts',(5.78910011906805,0.777699430509262,28.6989329581801));
#57148=CARTESIAN_POINT('Ctrl Pts',(2.48655015281781,5.28541035916478,28.8576937204261));
#57149=CARTESIAN_POINT('Ctrl Pts',(-3.09176592905605,4.95575179531496,29.0164544826718));
#57150=CARTESIAN_POINT('Ctrl Pts',(-5.84040367375386,0.0904380671616019,
29.1752152449178));
#57151=CARTESIAN_POINT('Ctrl Pts',(-3.24372543242543,-4.85764747523187,
29.3339760071636));
#57152=CARTESIAN_POINT('Ctrl Pts',(2.32170932913062,-5.35986560023234,29.4927367694096));
#57153=CARTESIAN_POINT('Ctrl Pts',(5.76224483502612,-0.956571044848404,
29.6514975316554));
#57154=CARTESIAN_POINT('Ctrl Pts',(3.92899783701638,4.32220656851071,29.8102582939014));
#57155=CARTESIAN_POINT('Ctrl Pts',(-1.50018798335741,5.64516869698926,29.9690190561472));
#57156=CARTESIAN_POINT('Ctrl Pts',(-5.55635594320173,1.80150000520858,30.1277798183931));
#57157=CARTESIAN_POINT('Ctrl Pts',(-4.52717721976122,-3.69095652156115,
30.286540580639));
#57158=CARTESIAN_POINT('Ctrl Pts',(0.645412378085751,-5.80533689665976,
30.4453013428849));
#57159=CARTESIAN_POINT('Ctrl Pts',(5.22730085393893,-2.60649561834369,30.6040621051308));
#57160=CARTESIAN_POINT('Ctrl Pts',(5.02500391786172,2.97789006670843,30.7628228673767));
#57161=CARTESIAN_POINT('Ctrl Pts',(0.223669905634492,5.83681980167278,30.9215836296225));
#57162=CARTESIAN_POINT('Ctrl Pts',(-4.78237363643064,3.35371376626822,31.0803443918685));
#57163=CARTESIAN_POINT('Ctrl Pts',(-5.41144274686964,-2.19881354860029,
31.2391051541144));
#57164=CARTESIAN_POINT('Ctrl Pts',(-1.08779416073393,-5.73891954012705,
31.3978659163602));
#57165=CARTESIAN_POINT('Ctrl Pts',(4.23143686842713,-4.0265910709645,31.5566266786062));
#57166=CARTESIAN_POINT('Ctrl Pts',(5.67792762467303,1.37099654017823,31.715387440852));
#57167=CARTESIAN_POINT('Ctrl Pts',(1.92780558426513,5.51380624011119,31.8741482030979));
#57168=CARTESIAN_POINT('Ctrl Pts',(-3.58670301245285,4.61021204769197,32.0329089653438));
#57169=CARTESIAN_POINT('Ctrl Pts',(-5.81855145490275,-0.512789031536669,
32.1916697275897));
#57170=CARTESIAN_POINT('Ctrl Pts',(-2.72508387585791,-5.16646992575742,
32.3504304898355));
#57171=CARTESIAN_POINT('Ctrl Pts',(2.86246370514321,-5.09163973204659,32.5091912520815));
#57172=CARTESIAN_POINT('Ctrl Pts',(5.83019706810478,-0.35678532940591,32.6679520143274));
#57173=CARTESIAN_POINT('Ctrl Pts',(3.46195598864868,4.7046099048568,32.8267127765732));
#57174=CARTESIAN_POINT('Ctrl Pts',(-2.0747729584413,5.46020245001391,32.9854735388191));
#57175=CARTESIAN_POINT('Ctrl Pts',(-5.71260631920057,1.21845092886281,33.144234301065));
#57176=CARTESIAN_POINT('Ctrl Pts',(-4.12208788279547,-4.13846410045175,
33.3029950633109));
#57177=CARTESIAN_POINT('Ctrl Pts',(1.24109129475792,-5.70773037400097,33.4617558255568));
#57178=CARTESIAN_POINT('Ctrl Pts',(5.46838580972161,-2.05310746437012,33.6205165878027));
#57179=CARTESIAN_POINT('Ctrl Pts',(4.69084659760865,3.48058210963631,33.7792773500486));
#57180=CARTESIAN_POINT('Ctrl Pts',(-0.379898704410712,5.82873662113877,
33.9380381122945));
#57181=CARTESIAN_POINT('Ctrl Pts',(-5.1029491079964,2.8422533358967,34.0967988745404));
#57182=CARTESIAN_POINT('Ctrl Pts',(-5.15562461633369,-2.74554702011659,
34.2555596367863));
#57183=CARTESIAN_POINT('Ctrl Pts',(-0.489714995198005,-5.82053887949348,
34.4143203990321));
#57184=CARTESIAN_POINT('Ctrl Pts',(4.62439674808221,-3.56839576568293,34.573081161278));
#57185=CARTESIAN_POINT('Ctrl Pts',(5.50611933347969,1.94965215094856,34.7318419235239));
#57186=CARTESIAN_POINT('Ctrl Pts',(1.3484733182716,5.68331886613153,34.8906026857698));
#57187=CARTESIAN_POINT('Ctrl Pts',(-4.04333666747246,4.2154385557958,35.0493634480157));
#57188=CARTESIAN_POINT('Ctrl Pts',(-5.73456142981912,-1.11053988305151,
35.2081242102616));
#57189=CARTESIAN_POINT('Ctrl Pts',(-2.17734040713567,-5.42011829904768,
35.3668849725075));
#57190=CARTESIAN_POINT('Ctrl Pts',(3.37264906388706,-4.76903888808624,35.5256457347534));
#57191=CARTESIAN_POINT('Ctrl Pts',(5.83588709273329,0.246810585441287,35.6844064969993));
#57192=CARTESIAN_POINT('Ctrl Pts',(2.95794299481775,5.03677147224547,35.8431672592451));
#57193=CARTESIAN_POINT('Ctrl Pts',(-2.62720088350026,5.21692525746274,36.001928021491));
#57194=CARTESIAN_POINT('Ctrl Pts',(-5.80785026434291,0.622389693993225,
36.160688783737));
#57195=CARTESIAN_POINT('Ctrl Pts',(-3.67297768016272,-4.54177592855961,
36.3194495459828));
#57196=CARTESIAN_POINT('Ctrl Pts',(1.82351626946645,-5.54916949094261,36.4782103082287));
#57197=CARTESIAN_POINT('Ctrl Pts',(5.65107242925025,-1.47779363362579,36.6369710704746));
#57198=CARTESIAN_POINT('Ctrl Pts',(4.30659448752927,3.94610409697964,36.7957318327205));
#57199=CARTESIAN_POINT('Ctrl Pts',(-0.979410275819905,5.7584068227102,36.9544925949664));
#57200=CARTESIAN_POINT('Ctrl Pts',(-5.36902883826232,2.30043973146977,37.1132533572123));
#57201=CARTESIAN_POINT('Ctrl Pts',(-4.84474820880581,-3.26296006985836,
37.2720141194581));
#57202=CARTESIAN_POINT('Ctrl Pts',(0.113593966110691,-5.839999146839,37.4307748817041));
#57203=CARTESIAN_POINT('Ctrl Pts',(4.96797147346979,-3.07209261953597,37.5895356439499));
#57204=CARTESIAN_POINT('Ctrl Pts',(5.27550973964484,2.50748691145728,37.7482964061959));
#57205=CARTESIAN_POINT('Ctrl Pts',(0.754740349553719,5.79213782889985,37.9070571684417));
#57206=CARTESIAN_POINT('Ctrl Pts',(-4.4567904622931,3.77564728217961,38.0658179306876));
#57207=CARTESIAN_POINT('Ctrl Pts',(-5.58933050861204,-1.69643098583928,
38.2245786929334));
#57208=CARTESIAN_POINT('Ctrl Pts',(-1.60634454512588,-5.6158837974589,38.3833394551794));
#57209=CARTESIAN_POINT('Ctrl Pts',(3.84681701249253,-4.39550821823998,38.5421002174252));
#57210=CARTESIAN_POINT('Ctrl Pts',(5.77925413772213,0.847770744858901,38.7008609796712));
#57211=CARTESIAN_POINT('Ctrl Pts',(2.42234134649229,5.31514402676831,38.859621741917));
#57212=CARTESIAN_POINT('Ctrl Pts',(-3.15157223642715,4.91793514219116,39.018382504163));
#57213=CARTESIAN_POINT('Ctrl Pts',(-5.84107064254106,0.0196817951957224,
39.1771432664088));
#57214=CARTESIAN_POINT('Ctrl Pts',(-3.18464277877548,-4.89658493195106,
39.3359040286547));
#57215=CARTESIAN_POINT('Ctrl Pts',(2.38646743230569,-5.33134756124203,39.4946647909006));
#57216=CARTESIAN_POINT('Ctrl Pts',(5.77340975374383,-0.886698054352646,
39.6534255531465));
#57217=CARTESIAN_POINT('Ctrl Pts',(3.87635111745847,4.36948459642503,39.8121863153924));
#57218=CARTESIAN_POINT('Ctrl Pts',(-1.56846246621147,5.62658147690965,39.9709470776383));
#57219=CARTESIAN_POINT('Ctrl Pts',(-5.57777129149482,1.73405912355756,40.1297078398841));
#57220=CARTESIAN_POINT('Ctrl Pts',(-4.48213345555963,-3.74552710720003,
40.2884686021301));
#57221=CARTESIAN_POINT('Ctrl Pts',(0.7156898274528,-5.79709252083298,40.4472293643759));
#57222=CARTESIAN_POINT('Ctrl Pts',(5.25849191934999,-2.5429817849029,40.6059901266219));
#57223=CARTESIAN_POINT('Ctrl Pts',(4.98856158393098,3.03854355696032,40.7647508888677));
#57224=CARTESIAN_POINT('Ctrl Pts',(0.152947309300711,5.83910102197203,40.9235116511136));
#57225=CARTESIAN_POINT('Ctrl Pts',(-4.82264901463799,3.29553487401187,41.0822724133595));
#57226=CARTESIAN_POINT('Ctrl Pts',(-5.38440965064774,-2.26420545406742,
41.2410331756054));
#57227=CARTESIAN_POINT('Ctrl Pts',(-1.0181941054504,-5.75167578952804,41.3997939378513));
#57228=CARTESIAN_POINT('Ctrl Pts',(4.27990378619904,-3.97503675518808,41.5585547000972));
#57229=CARTESIAN_POINT('Ctrl Pts',(5.66090300135578,1.43967733657867,41.7173154623431));
#57230=CARTESIAN_POINT('Ctrl Pts',(1.86087087513805,5.53675475439179,41.8760762245889));
#57231=CARTESIAN_POINT('Ctrl Pts',(-3.64228711704701,4.56642509860946,42.0348369868349));
#57232=CARTESIAN_POINT('Ctrl Pts',(-5.81191268460203,-0.583236290691027,
42.1935977490807));
#57233=CARTESIAN_POINT('Ctrl Pts',(-2.66229823602482,-5.19910201156664,
42.3523585113267));
#57234=CARTESIAN_POINT('Ctrl Pts',(2.92393287912081,-5.05659076281771,42.5111192735725));
#57235=CARTESIAN_POINT('Ctrl Pts',(5.83409131060233,-0.286133192362046,
42.6698800358184));
#57236=CARTESIAN_POINT('Ctrl Pts',(3.4047111699812,4.74620221579552,42.8286407980643));
#57237=CARTESIAN_POINT('Ctrl Pts',(-2.14076463166355,5.43466838142269,42.9874015603102));
#57238=CARTESIAN_POINT('Ctrl Pts',(-5.72694725190272,1.1491600402646,43.1461623225561));
#57239=CARTESIAN_POINT('Ctrl Pts',(-4.07165281531897,-4.18809467129411,
43.3049230848019));
#57240=CARTESIAN_POINT('Ctrl Pts',(1.31014264809932,-5.69227721266703,43.4636838470478));
#57241=CARTESIAN_POINT('Ctrl Pts',(5.49285554114887,-1.98671377613569,43.6224446092938));
#57242=CARTESIAN_POINT('Ctrl Pts',(4.64833926148183,3.53715079327751,43.7812053715396));
#57243=CARTESIAN_POINT('Ctrl Pts',(-0.450479095664875,5.82370691300532,
43.9399661337855));
#57244=CARTESIAN_POINT('Ctrl Pts',(-5.13700522439592,2.78022857850681,44.0987268960314));
#57245=CARTESIAN_POINT('Ctrl Pts',(-5.12198725989218,-2.80779987422883,
44.2574876582773));
#57246=CARTESIAN_POINT('Ctrl Pts',(-0.419170101997096,-5.82604411670637,
44.4162484205232));
#57247=CARTESIAN_POINT('Ctrl Pts',(4.66728433696318,-3.51211482473953,44.575009182769));
#57248=CARTESIAN_POINT('Ctrl Pts',(5.48209758667841,2.01620923377307,44.733769945015));
#57249=CARTESIAN_POINT('Ctrl Pts',(1.27952767221442,5.69923701562366,44.8925307072609));
#57250=CARTESIAN_POINT('Ctrl Pts',(-4.09410505154189,4.16614899531406,45.0512914695068));
#57251=CARTESIAN_POINT('Ctrl Pts',(-5.72068777605988,-1.17992584218497,
45.2100522317526));
#57252=CARTESIAN_POINT('Ctrl Pts',(-2.11152230724456,-5.4460965076122,45.3688129939986));
#57253=CARTESIAN_POINT('Ctrl Pts',(3.43017287444968,-4.72783329608889,45.5275737562444));
#57254=CARTESIAN_POINT('Ctrl Pts',(5.83246906545287,0.317487361563403,45.6863345184903));
#57255=CARTESIAN_POINT('Ctrl Pts',(2.89671141266624,5.07223388813511,45.8450952807362));
#57256=CARTESIAN_POINT('Ctrl Pts',(-2.69020500619468,5.1847170268841,46.003856042982));
#57257=CARTESIAN_POINT('Ctrl Pts',(-5.8149636300044,0.551988773385138,46.162616805228));
#57258=CARTESIAN_POINT('Ctrl Pts',(-3.61768991925726,-4.58593646623255,
46.3213775674738));
#57259=CARTESIAN_POINT('Ctrl Pts',(1.89060410937151,-5.5266725727009,46.4801383297198));
#57260=CARTESIAN_POINT('Ctrl Pts',(5.66855950784905,-1.40922912622162,46.6388990919655));
#57261=CARTESIAN_POINT('Ctrl Pts',(4.25847609633845,3.99798386203986,46.7976598542116));
#57262=CARTESIAN_POINT('Ctrl Pts',(-1.04909471538713,5.74611989975528,46.9564206164574));
#57263=CARTESIAN_POINT('Ctrl Pts',(-5.39650199857509,2.23523148769702,47.1151813787033));
#57264=CARTESIAN_POINT('Ctrl Pts',(-4.80486581436728,-3.32140905793637,
47.2739421409491));
#57265=CARTESIAN_POINT('Ctrl Pts',(0.184330329686807,-5.83819457998573,
47.4327029031951));
#57266=CARTESIAN_POINT('Ctrl Pts',(5.00482172556827,-3.01168609245668,47.5914636654409));
#57267=CARTESIAN_POINT('Ctrl Pts',(5.24474740393951,2.5712095000382,47.7502244276869));
#57268=CARTESIAN_POINT('Ctrl Pts',(0.684520055329939,5.80085561948134,47.9089851899327));
#57269=CARTESIAN_POINT('Ctrl Pts',(-4.50220095685495,3.72138148653313,48.0677459521787));
#57270=CARTESIAN_POINT('Ctrl Pts',(-5.56837013180732,-1.76401465396777,
48.2265067144245));
#57271=CARTESIAN_POINT('Ctrl Pts',(-1.53819687404933,-5.63493070062818,
48.3852674766705));
#57272=CARTESIAN_POINT('Ctrl Pts',(3.89978114767392,-4.3485860488743,48.5440282389163));
#57273=CARTESIAN_POINT('Ctrl Pts',(5.76856034267981,0.917717384099773,48.7027890011622));
#57274=CARTESIAN_POINT('Ctrl Pts',(2.35777690909515,5.34409783510322,48.8615497634081));
#57275=CARTESIAN_POINT('Ctrl Pts',(-3.21091597092679,4.87939670982634,49.020310525654));
#57276=CARTESIAN_POINT('Ctrl Pts',(-5.84088047565118,-0.0510773273967016,
49.1790712878999));
#57277=CARTESIAN_POINT('Ctrl Pts',(-3.12509275704243,-4.93480383440904,
49.3378320501458));
#57278=CARTESIAN_POINT('Ctrl Pts',(2.45087531001271,-5.3020471366244,49.4965928123917));
#57279=CARTESIAN_POINT('Ctrl Pts',(5.78372743038313,-0.816694946262622,
49.6553535746376));
#57280=CARTESIAN_POINT('Ctrl Pts',(3.82313554021223,4.41612140519068,49.8141143368834));
#57281=CARTESIAN_POINT('Ctrl Pts',(-1.63650677555656,5.60716855442876,49.9728750991293));
#57282=CARTESIAN_POINT('Ctrl Pts',(-5.59836810258563,1.66636376946,50.1316358613752));
#57283=CARTESIAN_POINT('Ctrl Pts',(-4.43643193774801,-3.79954803706259,
50.2903966236211));
#57284=CARTESIAN_POINT('Ctrl Pts',(0.785862249094534,-5.78799742135959,
50.4491573858669));
#57285=CARTESIAN_POINT('Ctrl Pts',(5.28891130109086,-2.47909476894502,50.6079181481129));
#57286=CARTESIAN_POINT('Ctrl Pts',(4.95138717842959,3.0987511409437,50.7666789103587));
#57287=CARTESIAN_POINT('Ctrl Pts',(0.0822022679789686,5.84052535405474,
50.9254396726047));
#57288=CARTESIAN_POINT('Ctrl Pts',(-4.86221666902701,3.23687236196503,51.0842004348505));
#57289=CARTESIAN_POINT('Ctrl Pts',(-5.35658639219748,-2.32926508734879,
51.2429611970965));
#57290=CARTESIAN_POINT('Ctrl Pts',(-0.948444630167017,-5.76358798039247,
51.4017219593423));
#57291=CARTESIAN_POINT('Ctrl Pts',(4.32774262801073,-3.92289910269379,51.5604827215883));
#57292=CARTESIAN_POINT('Ctrl Pts',(5.64304764041327,1.50814686030353,51.7192434838341));
#57293=CARTESIAN_POINT('Ctrl Pts',(1.79366308317505,5.55889074980541,51.87800424608));
#57294=CARTESIAN_POINT('Ctrl Pts',(-3.69733671593728,4.52196802655651,52.0367650083259));
#57295=CARTESIAN_POINT('Ctrl Pts',(-5.80442101600325,-0.653597959908777,
52.1955257705718));
#57296=CARTESIAN_POINT('Ctrl Pts',(-2.59912190387458,-5.2309711290559,52.3542865328177));
#57297=CARTESIAN_POINT('Ctrl Pts',(2.98497296589237,-5.02079973879747,52.5130472950635));
#57298=CARTESIAN_POINT('Ctrl Pts',(5.83712940008821,-0.215439065266698,
52.6718080573094));
#57299=CARTESIAN_POINT('Ctrl Pts',(3.34696670988424,4.78709802146808,52.8305688195553));
#57300=CARTESIAN_POINT('Ctrl Pts',(-2.20644214763509,5.4083367751423,52.9893295818012));
#57301=CARTESIAN_POINT('Ctrl Pts',(-5.74044775498584,1.07970051240847,53.1480903440471));
#57302=CARTESIAN_POINT('Ctrl Pts',(-4.02062023271376,-4.2371106391632,53.306851106293));
#57303=CARTESIAN_POINT('Ctrl Pts',(1.37900173798208,-5.675988709543,53.4656118685389));
#57304=CARTESIAN_POINT('Ctrl Pts',(5.51651919592013,-1.92002853761645,53.6243726307848));
#57305=CARTESIAN_POINT('Ctrl Pts',(4.60514978147925,3.59320039997198,53.7831333930307));
#57306=CARTESIAN_POINT('Ctrl Pts',(-0.520993379103106,5.81782257577076,
53.9418941552766));
#57307=CARTESIAN_POINT('Ctrl Pts',(-5.1703074851803,2.71779582251969,54.1006549175224));
#57308=CARTESIAN_POINT('Ctrl Pts',(-5.08759825172204,-2.86964068365571,
54.2594156797684));
#57309=CARTESIAN_POINT('Ctrl Pts',(-0.348563695575712,-5.83069438183342,
54.4181764420142));
#57310=CARTESIAN_POINT('Ctrl Pts',(4.70948700177826,-3.45531848087826,54.5769372042601));
#57311=CARTESIAN_POINT('Ctrl Pts',(5.45727134195117,2.08247043785393,54.735697966506));
#57312=CARTESIAN_POINT('Ctrl Pts',(1.21039425544677,5.71431880197442,54.8944587287519));
#57313=CARTESIAN_POINT('Ctrl Pts',(-4.14427262561643,4.11624805238744,55.0532194909978));
#57314=CARTESIAN_POINT('Ctrl Pts',(-5.70597461125989,-1.24913864717843,
55.2119802532437));
#57315=CARTESIAN_POINT('Ctrl Pts',(-2.04539434141439,-5.47127550140978,
55.3707410154896));
#57316=CARTESIAN_POINT('Ctrl Pts',(3.48719330707719,-4.68593389446471,55.5295017777355));
#57317=CARTESIAN_POINT('Ctrl Pts',(5.82819512322526,0.388117546408988,55.6882625399813));
#57318=CARTESIAN_POINT('Ctrl Pts',(2.83505473805949,5.10695195360438,55.8470233022273));
#57319=CARTESIAN_POINT('Ctrl Pts',(-2.75281434125286,5.15174793898243,56.0057840644731));
#57320=CARTESIAN_POINT('Ctrl Pts',(-5.82122364964165,0.481506848414017,
56.1645448267191));
#57321=CARTESIAN_POINT('Ctrl Pts',(-3.56187126228685,-4.6294240176411,56.3233055889649));
#57322=CARTESIAN_POINT('Ctrl Pts',(1.95741450308725,-5.50336461515325,56.4820663512108));
#57323=CARTESIAN_POINT('Ctrl Pts',(5.6852147252314,-1.34045781441613,56.6408271134567));
#57324=CARTESIAN_POINT('Ctrl Pts',(4.20973277369882,4.0492769228917,56.7995878757026));
#57325=CARTESIAN_POINT('Ctrl Pts',(-1.11862520028478,5.73298973359492,56.9583486379484));
#57326=CARTESIAN_POINT('Ctrl Pts',(-5.42318322211612,2.16969522366057,57.1171094001944));
#57327=CARTESIAN_POINT('Ctrl Pts',(-4.76427830577834,-3.3793706291715,57.2758701624402));
#57328=CARTESIAN_POINT('Ctrl Pts',(0.255039642783455,-5.83553325796587,
57.4346309246862));
#57329=CARTESIAN_POINT('Ctrl Pts',(5.04093751998252,-2.95083760038564,57.593391686932));
#57330=CARTESIAN_POINT('Ctrl Pts',(5.21321540145215,2.63455476357568,57.7521524491779));
#57331=CARTESIAN_POINT('Ctrl Pts',(0.614199307774883,5.80872213438946,57.9109132114238));
#57332=CARTESIAN_POINT('Ctrl Pts',(-4.54695075334007,3.66656957808212,58.0696739736697));
#57333=CARTESIAN_POINT('Ctrl Pts',(-5.54659259657899,-1.83133945291199,
58.2284347359156));
#57334=CARTESIAN_POINT('Ctrl Pts',(-1.469823472552,-5.65315067760911,58.3871954981615));
#57335=CARTESIAN_POINT('Ctrl Pts',(3.95217298989717,-4.30102572442254,58.5459562604074));
#57336=CARTESIAN_POINT('Ctrl Pts',(5.75702001129657,0.987529348296885,58.7047170226532));
#57337=CARTESIAN_POINT('Ctrl Pts',(2.29286646789146,5.37226739697831,58.8634777848992));
#57338=CARTESIAN_POINT('Ctrl Pts',(-3.26978850344612,4.84014222590088,59.022238547145));
#57339=CARTESIAN_POINT('Ctrl Pts',(-5.83983315943952,-0.121828954390395,
59.180999309391));
#57340=CARTESIAN_POINT('Ctrl Pts',(-3.06508412788734,-4.97229855430969,
59.3397600716368));
#57341=CARTESIAN_POINT('Ctrl Pts',(2.51492352172104,-5.27196863648781,59.4985208338828));
#57342=CARTESIAN_POINT('Ctrl Pts',(5.79319634491114,-0.746571988173542,
59.6572815961285));
#57343=CARTESIAN_POINT('Ctrl Pts',(3.76935891775212,4.46211014805548,59.8160423583745));
#57344=CARTESIAN_POINT('Ctrl Pts',(-1.70431092750091,5.58693277985496,59.9748031206203));
#57345=CARTESIAN_POINT('Ctrl Pts',(-5.61814335305001,1.59842387644741,60.1335638828663));
#57346=CARTESIAN_POINT('Ctrl Pts',(-4.39007937346456,-3.85301138317786,
60.2923246451121));
#57347=CARTESIAN_POINT('Ctrl Pts',(0.85591934543619,-5.77805293315363,60.451085407358));
#57348=CARTESIAN_POINT('Ctrl Pts',(5.31855453499689,-2.41484394578226,60.609846169604));
#57349=CARTESIAN_POINT('Ctrl Pts',(4.91348615676483,3.15850398313777,60.7686069318498));
#57350=CARTESIAN_POINT('Ctrl Pts',(0.0114451634727917,5.84109258892977,
60.9273676940957));
#57351=CARTESIAN_POINT('Ctrl Pts',(-4.90107079302665,3.17773483883697,61.0861284563416));
#57352=CARTESIAN_POINT('Ctrl Pts',(-5.32797705459145,-2.3939829009339,61.2448892185875));
#57353=CARTESIAN_POINT('Ctrl Pts',(-0.878555970616003,-5.77465436461024,
61.4036499808334));
#57354=CARTESIAN_POINT('Ctrl Pts',(4.37494637350877,-3.87018576468102,61.5624107430792));
#57355=CARTESIAN_POINT('Ctrl Pts',(5.62436416212133,1.57639506344776,61.7211715053253));
#57356=CARTESIAN_POINT('Ctrl Pts',(1.72619207112014,5.58021097789493,61.879932267571));
#57357=CARTESIAN_POINT('Ctrl Pts',(-3.75184373059352,4.47684735560896,62.038693029817));
#57358=CARTESIAN_POINT('Ctrl Pts',(-5.79607754850909,-0.723863713613315,
62.1974537920628));
#57359=CARTESIAN_POINT('Ctrl Pts',(-2.53556415053518,-5.26207260143168,
62.3562145543087));
#57360=CARTESIAN_POINT('Ctrl Pts',(3.04557500782399,-4.9842719123193,62.5149753165546));
#57361=CARTESIAN_POINT('Ctrl Pts',(5.8393108907227,-0.144713322484355,62.6737360788005));
#57362=CARTESIAN_POINT('Ctrl Pts',(3.28873108235841,4.82729132041423,62.8324968410464));
#57363=CARTESIAN_POINT('Ctrl Pts',(-2.27179586817918,5.38121149533645,62.9912576032922));
#57364=CARTESIAN_POINT('Ctrl Pts',(-5.75310584725087,1.01008253848138,63.1500183655383));
#57365=CARTESIAN_POINT('Ctrl Pts',(-3.96899762401232,-4.28550481096468,
63.3087791277839));
#57366=CARTESIAN_POINT('Ctrl Pts',(1.44765845933327,-5.65886725496703,63.4675398900301));
#57367=CARTESIAN_POINT('Ctrl Pts',(5.53937330139366,-1.85306153487257,63.6263006522757));
#57368=CARTESIAN_POINT('Ctrl Pts',(4.56128449565793,3.64872270443888,63.7850614145219));
#57369=CARTESIAN_POINT('Ctrl Pts',(-0.591431206752995,5.81108447296164,
63.9438221767675));
#57370=CARTESIAN_POINT('Ctrl Pts',(-5.20285100324211,2.65496422994348,64.1025829390136));
#57371=CARTESIAN_POINT('Ctrl Pts',(-5.05246263841092,-2.93106037325727,
64.2613437012593));
#57372=CARTESIAN_POINT('Ctrl Pts',(-0.277906137425253,-5.83448899244814,
64.4201044635054));
#57373=CARTESIAN_POINT('Ctrl Pts',(4.75099854928546,-3.3980150689637,64.5788652257511));
#57374=CARTESIAN_POINT('Ctrl Pts',(5.4316442425499,2.14842603935805,64.7376259879971));
#57375=CARTESIAN_POINT('Ctrl Pts',(1.14108321329899,5.72856201193147,64.896386750243));
#57376=CARTESIAN_POINT('Ctrl Pts',(-4.19383202760378,4.06574304998017,65.0551475124888));
#57377=CARTESIAN_POINT('Ctrl Pts',(-5.69042409457625,-1.31816814105151,
65.2139082747347));
#57378=CARTESIAN_POINT('Ctrl Pts',(-1.97896621392534,-5.49565158542271,
65.3726690369806));
#57379=CARTESIAN_POINT('Ctrl Pts',(3.54370199402013,-4.6433468319516,65.5314297992266));
#57380=CARTESIAN_POINT('Ctrl Pts',(5.82306589325152,0.458690774997357,65.6901905614723));
#57381=CARTESIAN_POINT('Ctrl Pts',(2.77298201911554,5.14092057377652,65.8489513237183));
#57382=CARTESIAN_POINT('Ctrl Pts',(-2.8150197007537,5.11802283197194,66.0077120859641));
#57383=CARTESIAN_POINT('Ctrl Pts',(-5.8266294045968,0.410954262303533,66.1664728482102));
#57384=CARTESIAN_POINT('Ctrl Pts',(-3.50552990064023,-4.67223220098639,
66.3252336104559));
#57385=CARTESIAN_POINT('Ctrl Pts',(2.0239376461872,-5.47924903874272,66.483994372702));
#57386=CARTESIAN_POINT('Ctrl Pts',(5.70103563724385,-1.27148979040063,66.6427551349476));
#57387=CARTESIAN_POINT('Ctrl Pts',(4.16037167269387,4.09997575227756,66.8015158971937));
#57388=CARTESIAN_POINT('Ctrl Pts',(-1.18799152691301,5.71901825108119,66.9602766594395));
#57389=CARTESIAN_POINT('Ctrl Pts',(-5.44906859341531,2.10384055680833,67.1190374216854));
#57390=CARTESIAN_POINT('Ctrl Pts',(-4.72299163925665,-3.43683627770202,
67.2777981839313));
#57391=CARTESIAN_POINT('Ctrl Pts',(0.325711528807802,-5.8320155713286,67.4365589461772));
#57392=CARTESIAN_POINT('Ctrl Pts',(5.07631355671921,-2.88955607283996,67.5953197084231));
#57393=CARTESIAN_POINT('Ctrl Pts',(5.18091835950451,2.6975134061513,67.754080470669));
#57394=CARTESIAN_POINT('Ctrl Pts',(0.54378842645952,5.81573621921296,67.9128412329148));
#57395=CARTESIAN_POINT('Ctrl Pts',(-4.59103328471497,3.61121960047518,68.0716019951608));
#57396=CARTESIAN_POINT('Ctrl Pts',(-5.52400109878079,-1.8983955027565,68.2303627574066));
#57397=CARTESIAN_POINT('Ctrl Pts',(-1.40123437443171,-5.67054105461978,
68.3891235196526));
#57398=CARTESIAN_POINT('Ctrl Pts',(4.00398485065851,-4.2528342243631,68.5478842818984));
#57399=CARTESIAN_POINT('Ctrl Pts',(5.74463483711628,1.05719639254342,68.7066450441444));
#57400=CARTESIAN_POINT('Ctrl Pts',(2.22761954848948,5.39964857850993,68.8654058063901));
#57401=CARTESIAN_POINT('Ctrl Pts',(-3.32818119444006,4.80017745101086,69.0241665686361));
#57402=CARTESIAN_POINT('Ctrl Pts',(-5.83792884759976,-0.192562702982879,
69.182927330882));
#57403=CARTESIAN_POINT('Ctrl Pts',(-3.00462569757752,-5.00906358930226,
69.3416880931278));
#57404=CARTESIAN_POINT('Ctrl Pts',(2.57860266835449,-5.24111647485266,69.5004488553739));
#57405=CARTESIAN_POINT('Ctrl Pts',(5.80181510776444,-0.676339470630766,
69.6592096176196));
#57406=CARTESIAN_POINT('Ctrl Pts',(3.71502914179852,4.50744407617051,69.8179703798656));
#57407=CARTESIAN_POINT('Ctrl Pts',(-1.77186497178415,5.56587712278864,69.9767311421114));
#57408=CARTESIAN_POINT('Ctrl Pts',(-5.63709414086971,1.53024941470006,70.1354919043573));
#57409=CARTESIAN_POINT('Ctrl Pts',(-4.34308256494864,-3.90590929979895,
70.2942526666033));
#57410=CARTESIAN_POINT('Ctrl Pts',(0.925850835597592,-5.7672605155689,70.453013428849));
#57411=CARTESIAN_POINT('Ctrl Pts',(5.34741727092293,-2.35023874422409,70.6117741910951));
#57412=CARTESIAN_POINT('Ctrl Pts',(4.87486408091236,3.21779331481187,70.7705349533408));
#57413=CARTESIAN_POINT('Ctrl Pts',(-0.0593136206115266,5.8408026433554,
70.9292957155867));
#57414=CARTESIAN_POINT('Ctrl Pts',(-4.93920568479356,3.11813098306019,71.0880564778327));
#57415=CARTESIAN_POINT('Ctrl Pts',(-5.29858583625043,-2.45834939748262,
71.2468172400784));
#57416=CARTESIAN_POINT('Ctrl Pts',(-0.808538382959287,-5.78487331818929,
71.4055780023245));
#57417=CARTESIAN_POINT('Ctrl Pts',(4.42150809554277,-3.81690447683292,71.5643387645703));
#57418=CARTESIAN_POINT('Ctrl Pts',(5.60485530828073,1.64441193058638,71.7230995268162));
#57419=CARTESIAN_POINT('Ctrl Pts',(1.65846774034549,5.6007123099165,71.8818602890621));
#57420=CARTESIAN_POINT('Ctrl Pts',(-3.80580016211055,4.43106970722601,72.040621051308));
#57421=CARTESIAN_POINT('Ctrl Pts',(-5.78688350652351,-0.794023240304163,
72.1993818135539));
#57422=CARTESIAN_POINT('Ctrl Pts',(-2.47163430310789,-5.29240186455242,
72.3581425757998));
#57423=CARTESIAN_POINT('Ctrl Pts',(3.10573011156498,-4.94701264384235,72.5169033380457));
#57424=CARTESIAN_POINT('Ctrl Pts',(5.84063546237199,-0.0739663430189528,
72.6756641002916));
#57425=CARTESIAN_POINT('Ctrl Pts',(3.23001283348305,4.86677621426665,72.8344248625374));
#57426=CARTESIAN_POINT('Ctrl Pts',(-2.33681620263615,5.35329652264041,72.9931856247833));
#57427=CARTESIAN_POINT('Ctrl Pts',(-5.76491967112249,0.940316334922364,
73.1519463870293));
#57428=CARTESIAN_POINT('Ctrl Pts',(-3.9167925648334,-4.33327008485316,73.3107071492751));
#57429=CARTESIAN_POINT('Ctrl Pts',(1.51610273677804,-5.64091536151285,73.469467911521));
#57430=CARTESIAN_POINT('Ctrl Pts',(5.56141450372903,-1.78582259531264,73.6282286737669));
#57431=CARTESIAN_POINT('Ctrl Pts',(4.51674984124932,3.70370955877901,73.7869894360128));
#57432=CARTESIAN_POINT('Ctrl Pts',(-0.661782241861996,5.80349359339467,
73.9457501982587));
#57433=CARTESIAN_POINT('Ctrl Pts',(-5.23463100281954,2.59174302131558,74.1045109605046));
#57434=CARTESIAN_POINT('Ctrl Pts',(-5.01658557611066,-2.99204992969303,
74.2632717227504));
#57435=CARTESIAN_POINT('Ctrl Pts',(-0.207207796543587,-5.83742739169134,
74.4220324849964));
#57436=CARTESIAN_POINT('Ctrl Pts',(4.79181288766461,-3.34021299827244,74.5807932472422));
#57437=CARTESIAN_POINT('Ctrl Pts',(5.4052200492518,2.21406635929985,74.7395540094881));
#57438=CARTESIAN_POINT('Ctrl Pts',(1.07160471716756,5.7419645553035,74.8983147717341));
#57439=CARTESIAN_POINT('Ctrl Pts',(-4.2427759846608,4.01464139970224,75.0570755339798));
#57440=CARTESIAN_POINT('Ctrl Pts',(-5.67403850804756,-1.38700419372482,
75.2158362962259));
#57441=CARTESIAN_POINT('Ctrl Pts',(-1.91224767310636,-5.51922118246009,
75.3745970584716));
#57442=CARTESIAN_POINT('Ctrl Pts',(3.59969064262747,-4.60007835820185,75.5333578207176));
#57443=CARTESIAN_POINT('Ctrl Pts',(5.81708212824635,0.529196690705634,75.6921185829634));
#57444=CARTESIAN_POINT('Ctrl Pts',(2.71050236500702,5.17413476375605,75.8508793452094));
#57445=CARTESIAN_POINT('Ctrl Pts',(-2.87681195605961,5.08354665501262,76.0096401074552));
#57446=CARTESIAN_POINT('Ctrl Pts',(-5.83118010157501,0.340341368647152,
76.1684008697012));
#57447=CARTESIAN_POINT('Ctrl Pts',(-3.4486741024136,-4.71435473416655,76.327161631947));
#57448=CARTESIAN_POINT('Ctrl Pts',(2.09016377639872,-5.45432938243075,76.4859223941929));
#57449=CARTESIAN_POINT('Ctrl Pts',(5.71601992216721,-1.20233517523405,76.6446831564388));
#57450=CARTESIAN_POINT('Ctrl Pts',(4.11040003706624,4.15007291014307,76.8034439186847));
#57451=CARTESIAN_POINT('Ctrl Pts',(-1.25718351576172,5.7042075025295,76.9622046809306));
#57452=CARTESIAN_POINT('Ctrl Pts',(-5.47415431379396,2.03767715131415,77.1209654431764));
#57453=CARTESIAN_POINT('Ctrl Pts',(-4.68101187362137,-3.49379757044288,
77.2797262054223));
#57454=CARTESIAN_POINT('Ctrl Pts',(0.39633561665894,-5.82764203629436,77.4384869676682));
#57455=CARTESIAN_POINT('Ctrl Pts',(5.11094464434401,-2.82785050288533,77.5972477299141));
#57456=CARTESIAN_POINT('Ctrl Pts',(5.1478610176884,2.76007618858267,77.75600849216));
#57457=CARTESIAN_POINT('Ctrl Pts',(0.473297744182263,5.82189684463481,77.9147692544059));
#57458=CARTESIAN_POINT('Ctrl Pts',(-4.63444208186731,3.55533967632268,78.0735300166519));
#57459=CARTESIAN_POINT('Ctrl Pts',(-5.50059895371541,-1.96517296302448,
78.2322907788976));
#57460=CARTESIAN_POINT('Ctrl Pts',(-1.33243964514028,-5.6870992796219,78.3910515411437));
#57461=CARTESIAN_POINT('Ctrl Pts',(4.0552091265661,-4.20401862079985,78.5498123033894));
#57462=CARTESIAN_POINT('Ctrl Pts',(5.73140663766353,1.12670829319891,78.7085730656353));
#57463=CARTESIAN_POINT('Ctrl Pts',(2.16204572587615,5.42623736150913,78.8673338278812));
#57464=CARTESIAN_POINT('Ctrl Pts',(-3.38608547477963,4.75950824998793,79.0260945901272));
#57465=CARTESIAN_POINT('Ctrl Pts',(-5.83516781958967,-0.263268192994679,
79.184855352373));
#57466=CARTESIAN_POINT('Ctrl Pts',(-2.94372633838929,-5.04509354411697,
79.3436161146189));
#57467=CARTESIAN_POINT('Ctrl Pts',(2.64190340499678,-5.2094951792744,79.5023768768649));
#57468=CARTESIAN_POINT('Ctrl Pts',(5.80958245413942,-0.606007700257848,
79.6611376391106));
#57469=CARTESIAN_POINT('Ctrl Pts',(3.66015418524723,4.55211653678098,79.8198984013567));
#57470=CARTESIAN_POINT('Ctrl Pts',(-1.8391589948488,5.54400467314773,79.9786591636023));
#57471=CARTESIAN_POINT('Ctrl Pts',(-5.65521768501588,1.46185038882208,80.1374199258485));
#57472=CARTESIAN_POINT('Ctrl Pts',(-4.29544840898361,-3.95823402415551,
80.2961806880941));
#57473=CARTESIAN_POINT('Ctrl Pts',(0.995646457131763,-5.7556217523925,80.4549414503402));
#57474=CARTESIAN_POINT('Ctrl Pts',(5.3754952732605,-2.28528864508612,80.613702212586));
#57475=CARTESIAN_POINT('Ctrl Pts',(4.83552661866532,3.27661043525698,80.7724629748319));
#57476=CARTESIAN_POINT('Ctrl Pts',(-0.130063700425983,5.83965555987772,
80.9312237370779));
#57477=CARTESIAN_POINT('Ctrl Pts',(-4.9766157480213,3.05806954150856,81.0899844993236));
#57478=CARTESIAN_POINT('Ctrl Pts',(-5.26841705035579,-2.52235513122241,
81.2487452615697));
#57479=CARTESIAN_POINT('Ctrl Pts',(-0.738402142242399,-5.79424334147416,
81.4075060238153));
#57480=CARTESIAN_POINT('Ctrl Pts',(4.46742096110774,-3.76306305822547,81.5662667860616));
#57481=CARTESIAN_POINT('Ctrl Pts',(5.58452394195224,1.71218748032981,81.7250275483071));
#57482=CARTESIAN_POINT('Ctrl Pts',(1.590500029138,5.62039173713168,81.8837883105533));
#57483=CARTESIAN_POINT('Ctrl Pts',(-3.85919809188181,4.38464179959952,82.0425490727989));
#57484=CARTESIAN_POINT('Ctrl Pts',(-5.776840240228,-0.864066244683674,82.201309835045));
#57485=CARTESIAN_POINT('Ctrl Pts',(-2.40734174146917,-5.3219544664209,82.3600705972908));
#57486=CARTESIAN_POINT('Ctrl Pts',(3.16542944584671,-4.9090274034195,82.5188313595367));
#57487=CARTESIAN_POINT('Ctrl Pts',(5.84110292736961,-0.00320850467390637,
82.6775921217826));
#57488=CARTESIAN_POINT('Ctrl Pts',(3.1708205673024,4.90554690034638,82.8363528840285));
#57489=CARTESIAN_POINT('Ctrl Pts',(-2.40149358463894,5.32459596941663,82.9951136462743));
#57490=CARTESIAN_POINT('Ctrl Pts',(-5.7758875400995,0.870412109585264,83.1538744085203));
#57491=CARTESIAN_POINT('Ctrl Pts',(-3.86401262590961,-4.3803993931662,83.3126351707661));
#57492=CARTESIAN_POINT('Ctrl Pts',(1.58432435304567,-5.62213577491609,83.4713959330121));
#57493=CARTESIAN_POINT('Ctrl Pts',(5.58263989986849,-1.71832137308609,83.6301566952579));
#57494=CARTESIAN_POINT('Ctrl Pts',(4.47155171880276,3.75815248538495,83.7889174575037));
#57495=CARTESIAN_POINT('Ctrl Pts',(-0.732034944345687,5.79505183303421,
83.9476782197497));
#57496=CARTESIAN_POINT('Ctrl Pts',(-5.26564514937354,2.52813997655405,84.1064389819955));
#57497=CARTESIAN_POINT('Ctrl Pts',(-4.97996786863125,-3.05259753396621,
84.2651997442416));
#57498=CARTESIAN_POINT('Ctrl Pts',(-0.136487592502867,-5.83951464301881,
84.4239605064873));
#57499=CARTESIAN_POINT('Ctrl Pts',(4.83194039314673,-3.28191022714265,84.5827212687333));
#57500=CARTESIAN_POINT('Ctrl Pts',(5.3779712939643,2.27936160776507,84.7414820309791));
#57501=CARTESIAN_POINT('Ctrl Pts',(1.00202900079473,5.75456307304708,84.9002427932251));
#57502=CARTESIAN_POINT('Ctrl Pts',(-4.29121230689459,3.96287665367137,85.059003555471));
#57503=CARTESIAN_POINT('Ctrl Pts',(-5.65660000441566,-1.45549506770408,
85.2177643177168));
#57504=CARTESIAN_POINT('Ctrl Pts',(-1.84567038925739,-5.54225213649743,
85.3765250799627));
#57505=CARTESIAN_POINT('Ctrl Pts',(3.65595928985271,-4.55561497937659,85.5352858422086));
#57506=CARTESIAN_POINT('Ctrl Pts',(5.8086947012646,0.598627392648328,85.6940466044544));
#57507=CARTESIAN_POINT('Ctrl Pts',(2.65061116100751,5.20851728785982,85.8528073667005));
#57508=CARTESIAN_POINT('Ctrl Pts',(-2.94405900471206,5.04447882807405,86.0115681289463));
#57509=CARTESIAN_POINT('Ctrl Pts',(-5.34253328840157,1.07278402652743,86.1438687641512));
#57510=CARTESIAN_POINT('Ctrl Pts',(-4.62260421807956,-2.25450493511227,
86.2497092723151));
#57511=CARTESIAN_POINT('Ctrl Pts',(-3.53826020855044,-3.54670961616112,
86.3026295263971));
#57512=CARTESIAN_POINT('Ctrl Pts',(-2.86929757049814,-4.02374147429149,
86.3290896534381));
#57513=CARTESIAN_POINT('',(-2.16917135428524,4.44050218283342,86.));
#57514=CARTESIAN_POINT('Ctrl Pts',(-2.17574227734826,4.44486702454923,86.));
#57515=CARTESIAN_POINT('Ctrl Pts',(-2.28013295862628,4.38716599510334,86.));
#57516=CARTESIAN_POINT('Ctrl Pts',(-2.38203491056673,4.32558764363711,86.));
#57517=CARTESIAN_POINT('Ctrl Pts',(-2.48120820121107,4.26013722079047,86.));
#57518=CARTESIAN_POINT('Ctrl Pts',(-2.60006688906204,4.18169521963978,86.));
#57519=CARTESIAN_POINT('Ctrl Pts',(-2.7150074127347,4.09769239705542,86.));
#57520=CARTESIAN_POINT('Ctrl Pts',(-2.825877147636,4.00855468944723,86.));
#57521=CARTESIAN_POINT('Ctrl Pts',(-2.93875239431318,3.9178045785764,86.));
#57522=CARTESIAN_POINT('Ctrl Pts',(-3.04740870522866,3.82173148785291,86.));
#57523=CARTESIAN_POINT('Ctrl Pts',(-3.15164741290182,3.72074618418362,86.));
#57524=CARTESIAN_POINT('Ctrl Pts',(-3.25648521909179,3.61918048051708,86.));
#57525=CARTESIAN_POINT('Ctrl Pts',(-3.35685490813916,3.51264518527105,86.));
#57526=CARTESIAN_POINT('Ctrl Pts',(-3.45251018852357,3.40153010769327,86.));
#57527=CARTESIAN_POINT('Ctrl Pts',(-3.48145067837577,3.36791225866138,86.));
#57528=CARTESIAN_POINT('Ctrl Pts',(-3.50995929996644,3.33387504208837,86.));
#57529=CARTESIAN_POINT('Ctrl Pts',(-3.53802835306874,3.2994289123823,86.));
#57530=CARTESIAN_POINT('Ctrl Pts',(-3.55893895860226,3.27376757539972,86.));
#57531=CARTESIAN_POINT('Ctrl Pts',(-3.57960560368256,3.24787929661303,86.));
#57532=CARTESIAN_POINT('Ctrl Pts',(-3.60002494885949,3.22176835839145,86.));
#57533=CARTESIAN_POINT('Ctrl Pts',(-3.61193639941707,3.20653676565705,86.));
#57534=CARTESIAN_POINT('Ctrl Pts',(-3.62375830311465,3.19123627397227,86.));
#57535=CARTESIAN_POINT('Ctrl Pts',(-3.63548790188773,3.17587102356872,86.));
#57536=CARTESIAN_POINT('Ctrl Pts',(-3.72304104356389,3.06118031918079,86.));
#57537=CARTESIAN_POINT('Ctrl Pts',(-3.80549810494951,2.94282892853622,86.));
#57538=CARTESIAN_POINT('Ctrl Pts',(-3.88269282098784,2.82123575460696,86.));
#57539=CARTESIAN_POINT('Ctrl Pts',(-3.96010237178875,2.69930418393253,86.));
#57540=CARTESIAN_POINT('Ctrl Pts',(-4.03222060518193,2.57411198603205,86.));
#57541=CARTESIAN_POINT('Ctrl Pts',(-4.09883515477919,2.44605409339683,86.));
#57542=CARTESIAN_POINT('Ctrl Pts',(-4.16485320331115,2.31914289723916,86.));
#57543=CARTESIAN_POINT('Ctrl Pts',(-4.2254659552961,2.18941632853557,86.));
#57544=CARTESIAN_POINT('Ctrl Pts',(-4.28041834739517,2.05724343991072,86.));
#57545=CARTESIAN_POINT('Ctrl Pts',(-4.33438117280193,1.92745068221766,86.));
#57546=CARTESIAN_POINT('Ctrl Pts',(-4.38288583069982,1.79529822126205,86.));
#57547=CARTESIAN_POINT('Ctrl Pts',(-4.42564090526442,1.66113144401598,86.));
#57548=CARTESIAN_POINT('Ctrl Pts',(-4.43255967958786,1.63942011119941,86.));
#57549=CARTESIAN_POINT('Ctrl Pts',(-4.43932777954855,1.61765603376178,86.));
#57550=CARTESIAN_POINT('Ctrl Pts',(-4.4459438397712,1.59584068384471,86.));
#57551=CARTESIAN_POINT('Ctrl Pts',(-4.45171251084707,1.57681945764039,86.));
#57552=CARTESIAN_POINT('Ctrl Pts',(-4.45736585345657,1.55775815091916,86.));
#57553=CARTESIAN_POINT('Ctrl Pts',(-4.46289825998277,1.53867450299572,86.));
#57554=CARTESIAN_POINT('Ctrl Pts',(-4.50224730205451,1.40294274476988,86.));
#57555=CARTESIAN_POINT('Ctrl Pts',(-4.53554254717084,1.2658880814313,86.));
#57556=CARTESIAN_POINT('Ctrl Pts',(-4.56258502829437,1.12787819891714,86.));
#57557=CARTESIAN_POINT('Ctrl Pts',(-4.58931759393923,0.991449953775849,
86.));
#57558=CARTESIAN_POINT('Ctrl Pts',(-4.60994008626122,0.854087541637941,
86.));
#57559=CARTESIAN_POINT('Ctrl Pts',(-4.62421031200347,0.716138535076822,
86.));
#57560=CARTESIAN_POINT('Ctrl Pts',(-4.63813932416541,0.581488009932714,
86.));
#57561=CARTESIAN_POINT('Ctrl Pts',(-4.64601628194546,0.446277995360083,
86.));
#57562=CARTESIAN_POINT('Ctrl Pts',(-4.64756630557454,0.310834136529796,
86.));
#57563=CARTESIAN_POINT('Ctrl Pts',(-4.64793240287716,0.278843894287929,
86.));
#57564=CARTESIAN_POINT('Ctrl Pts',(-4.6479453277195,0.246840640295154,86.));
#57565=CARTESIAN_POINT('Ctrl Pts',(-4.64760103388387,0.214828741346587,
86.));
#57566=CARTESIAN_POINT('Ctrl Pts',(-4.64657805635091,0.119713900408526,
86.));
#57567=CARTESIAN_POINT('Ctrl Pts',(-4.64240219271064,0.0245223992060761,
86.));
#57568=CARTESIAN_POINT('Ctrl Pts',(-4.63512171526216,-0.0706009649893001,
86.));
#57569=CARTESIAN_POINT('Ctrl Pts',(-4.63272301775774,-0.101941241491998,
86.));
#57570=CARTESIAN_POINT('Ctrl Pts',(-4.62998723239254,-0.133274083991166,
86.));
#57571=CARTESIAN_POINT('Ctrl Pts',(-4.62691585213729,-0.16459419159554,
86.));
#57572=CARTESIAN_POINT('Ctrl Pts',(-4.62511596030474,-0.182948417118559,
86.));
#57573=CARTESIAN_POINT('Ctrl Pts',(-4.62320081633973,-0.201298267969776,
86.));
#57574=CARTESIAN_POINT('Ctrl Pts',(-4.62117070299388,-0.21964266601306,
86.));
#57575=CARTESIAN_POINT('Ctrl Pts',(-4.61910605502354,-0.238299123921961,
86.));
#57576=CARTESIAN_POINT('Ctrl Pts',(-4.6169235721841,-0.256940116225532,
86.));
#57577=CARTESIAN_POINT('Ctrl Pts',(-4.61462417515337,-0.275562596752177,
86.));
#57578=CARTESIAN_POINT('Ctrl Pts',(-4.59791089402231,-0.410921018216574,
86.));
#57579=CARTESIAN_POINT('Ctrl Pts',(-4.57502130177171,-0.545336418557933,
86.));
#57580=CARTESIAN_POINT('Ctrl Pts',(-4.54619383694625,-0.678403869974182,
86.));
#57581=CARTESIAN_POINT('Ctrl Pts',(-4.51690235263596,-0.81361323330078,
86.));
#57582=CARTESIAN_POINT('Ctrl Pts',(-4.48148002405017,-0.947431726142265,
86.));
#57583=CARTESIAN_POINT('Ctrl Pts',(-4.44012512005541,-1.07942238906511,
86.));
#57584=CARTESIAN_POINT('Ctrl Pts',(-4.39891579514076,-1.21094841351862,
86.));
#57585=CARTESIAN_POINT('Ctrl Pts',(-4.35181516564808,-1.34066022876501,
86.));
#57586=CARTESIAN_POINT('Ctrl Pts',(-4.29897383984103,-1.46810153698611,
86.));
#57587=CARTESIAN_POINT('Ctrl Pts',(-4.26316764637209,-1.55445796480857,
86.));
#57588=CARTESIAN_POINT('Ctrl Pts',(-4.22472458946287,-1.639771352916,86.));
#57589=CARTESIAN_POINT('Ctrl Pts',(-4.18368102987994,-1.72389071907676,
86.));
#57590=CARTESIAN_POINT('Ctrl Pts',(-4.16189573536735,-1.76853999376555,
86.));
#57591=CARTESIAN_POINT('Ctrl Pts',(-4.13937765883534,-1.81285273679093,
86.));
#57592=CARTESIAN_POINT('Ctrl Pts',(-4.11613135978827,-1.85680534418916,
86.));
#57593=CARTESIAN_POINT('Ctrl Pts',(-4.10598652796122,-1.87598653985015,
86.));
#57594=CARTESIAN_POINT('Ctrl Pts',(-4.09570182816448,-1.8951012704791,86.));
#57595=CARTESIAN_POINT('Ctrl Pts',(-4.08528136703263,-1.91414066944428,
86.));
#57596=CARTESIAN_POINT('Ctrl Pts',(-4.07459370444932,-1.93366827665418,
86.));
#57597=CARTESIAN_POINT('Ctrl Pts',(-4.06376686324371,-1.95311008122927,
86.));
#57598=CARTESIAN_POINT('Ctrl Pts',(-4.05280165642382,-1.97246424292779,
86.));
#57599=CARTESIAN_POINT('Ctrl Pts',(-3.98545341209713,-2.09133740530588,
86.));
#57600=CARTESIAN_POINT('Ctrl Pts',(-3.91288886269624,-2.20690686036164,
86.));
#57601=CARTESIAN_POINT('Ctrl Pts',(-3.83535609314517,-2.31888838615919,
86.));
#57602=CARTESIAN_POINT('Ctrl Pts',(-3.75793727989042,-2.43070532348649,
86.));
#57603=CARTESIAN_POINT('Ctrl Pts',(-3.67556431499777,-2.53894540267671,
86.));
#57604=CARTESIAN_POINT('Ctrl Pts',(-3.58844692437017,-2.6432897533722,86.));
#57605=CARTESIAN_POINT('Ctrl Pts',(-3.55106838804729,-2.68805967903758,
86.));
#57606=CARTESIAN_POINT('Ctrl Pts',(-3.51281602034817,-2.7321119355856,86.));
#57607=CARTESIAN_POINT('Ctrl Pts',(-3.47370464217661,-2.77541893263456,
86.));
#57608=CARTESIAN_POINT('Ctrl Pts',(-3.45527487716358,-2.79582572514213,
86.));
#57609=CARTESIAN_POINT('Ctrl Pts',(-3.43665436275494,-2.81606701722102,
86.));
#57610=CARTESIAN_POINT('Ctrl Pts',(-3.41784457942235,-2.83613979970913,
86.));
#57611=CARTESIAN_POINT('Ctrl Pts',(-3.40161580152966,-2.85345827291681,
86.));
#57612=CARTESIAN_POINT('Ctrl Pts',(-3.38525177230088,-2.87064524159307,
86.));
#57613=CARTESIAN_POINT('Ctrl Pts',(-3.36875789576418,-2.88769480011766,
86.));
#57614=CARTESIAN_POINT('Ctrl Pts',(-3.27548691461708,-2.98410809920928,
86.));
#57615=CARTESIAN_POINT('Ctrl Pts',(-3.1780247285723,-3.07617507300169,86.));
#57616=CARTESIAN_POINT('Ctrl Pts',(-3.07658549505738,-3.16359906081916,
86.));
#57617=CARTESIAN_POINT('Ctrl Pts',(-2.97674507744291,-3.24964513146433,
86.));
#57618=CARTESIAN_POINT('Ctrl Pts',(-2.87305144560376,-3.33119379608769,
86.));
#57619=CARTESIAN_POINT('Ctrl Pts',(-2.76568166074672,-3.40792026882373,
86.));
#57620=CARTESIAN_POINT('Ctrl Pts',(-2.691638695275,-3.46083138882947,86.));
#57621=CARTESIAN_POINT('Ctrl Pts',(-2.61584694697416,-3.51144841450292,
86.));
#57622=CARTESIAN_POINT('Ctrl Pts',(-2.53835875722777,-3.5596515025498,86.));
#57623=CARTESIAN_POINT('Ctrl Pts',(-4.94096920053978,-0.0044629540342261,
85.1776795453431));
#57624=CARTESIAN_POINT('Ctrl Pts',(-4.94470425404279,-0.419442432737937,
85.1910411361343));
#57625=CARTESIAN_POINT('Ctrl Pts',(-4.89679105157154,-0.83357493998294,
85.2044027269256));
#57626=CARTESIAN_POINT('Ctrl Pts',(-4.79388045230233,-1.23355929227409,
85.2177643177168));
#57627=CARTESIAN_POINT('Ctrl Pts',(-4.38629013269605,-2.81774742396872,
85.2706845717988));
#57628=CARTESIAN_POINT('Ctrl Pts',(-3.11598026097668,-4.17999978023304,
85.3236048258808));
#57629=CARTESIAN_POINT('Ctrl Pts',(-1.5638870452654,-4.69668643217841,85.3765250799627));
#57630=CARTESIAN_POINT('Ctrl Pts',(-0.0117938295540432,-5.21337308412381,
85.4294453340447));
#57631=CARTESIAN_POINT('Ctrl Pts',(1.82208273014937,-4.88449403175019,85.4823655881266));
#57632=CARTESIAN_POINT('Ctrl Pts',(3.09781024523634,-3.86101411022591,85.5352858422086));
#57633=CARTESIAN_POINT('Ctrl Pts',(4.37353776032332,-2.83753418870164,85.5882060962905));
#57634=CARTESIAN_POINT('Ctrl Pts',(5.0911162307939,-1.11945339802691,85.6411263503725));
#57635=CARTESIAN_POINT('Ctrl Pts',(4.92355820931981,0.507901979845797,85.6940466044544));
#57636=CARTESIAN_POINT('Ctrl Pts',(4.75600018784572,2.1352573577185,85.7469668585364));
#57637=CARTESIAN_POINT('Ctrl Pts',(3.70330567442676,3.67188732278906,85.7998871126184));
#57638=CARTESIAN_POINT('Ctrl Pts',(2.24451339009742,4.41286256202677,85.8528073667004));
#57639=CARTESIAN_POINT('Ctrl Pts',(0.892016244518137,5.09984651908455,85.9018715778003));
#57640=CARTESIAN_POINT('Ctrl Pts',(-0.809554018707134,5.10290237899098,
85.9509357889001));
#57641=CARTESIAN_POINT('Ctrl Pts',(-2.17574227734751,4.44486702454959,86.));
#57642=CARTESIAN_POINT('',(-2.53835875722709,-3.55965150255029,26.));
#57643=CARTESIAN_POINT('Ctrl Pts',(-2.54472725763298,-3.56250530678305,
26.));
#57644=CARTESIAN_POINT('Ctrl Pts',(-2.63508309937759,-3.50703322951937,
26.));
#57645=CARTESIAN_POINT('Ctrl Pts',(-2.72311007746572,-3.44818980724315,
26.));
#57646=CARTESIAN_POINT('Ctrl Pts',(-2.80858488092082,-3.38601400346164,
26.));
#57647=CARTESIAN_POINT('Ctrl Pts',(-2.91385291450225,-3.30944027253914,
26.));
#57648=CARTESIAN_POINT('Ctrl Pts',(-3.01525129898596,-3.22781364096124,
26.));
#57649=CARTESIAN_POINT('Ctrl Pts',(-3.11268784287649,-3.1415518359691,26.));
#57650=CARTESIAN_POINT('Ctrl Pts',(-3.17680627098234,-3.08478698039414,
26.));
#57651=CARTESIAN_POINT('Ctrl Pts',(-3.23920859831056,-3.02601391139215,
26.));
#57652=CARTESIAN_POINT('Ctrl Pts',(-3.29986195943645,-2.96534150637499,
26.));
#57653=CARTESIAN_POINT('Ctrl Pts',(-3.33570437568566,-2.9294878363541,26.));
#57654=CARTESIAN_POINT('Ctrl Pts',(-3.37093593415121,-2.89297075792499,
26.));
#57655=CARTESIAN_POINT('Ctrl Pts',(-3.40554888779674,-2.85581160143786,
26.));
#57656=CARTESIAN_POINT('Ctrl Pts',(-3.4189115430604,-2.84146596069563,26.));
#57657=CARTESIAN_POINT('Ctrl Pts',(-3.43218080021828,-2.82702583304496,
26.));
#57658=CARTESIAN_POINT('Ctrl Pts',(-3.44534999888201,-2.81249952818835,
26.));
#57659=CARTESIAN_POINT('Ctrl Pts',(-3.53470458244056,-2.71393681725578,
26.));
#57660=CARTESIAN_POINT('Ctrl Pts',(-3.61953742655147,-2.6113223183339,26.));
#57661=CARTESIAN_POINT('Ctrl Pts',(-3.69975229053408,-2.50508736800556,
26.));
#57662=CARTESIAN_POINT('Ctrl Pts',(-3.78158309623279,-2.39671229701354,
26.));
#57663=CARTESIAN_POINT('Ctrl Pts',(-3.85860846570253,-2.28456889207013,
26.));
#57664=CARTESIAN_POINT('Ctrl Pts',(-3.93069241652625,-2.16907329602735,
26.));
#57665=CARTESIAN_POINT('Ctrl Pts',(-3.96222914501164,-2.11854397275863,
26.));
#57666=CARTESIAN_POINT('Ctrl Pts',(-3.99281958123178,-2.06737253695488,
26.));
#57667=CARTESIAN_POINT('Ctrl Pts',(-4.02244999738294,-2.01559181929177,
26.));
#57668=CARTESIAN_POINT('Ctrl Pts',(-4.03719360535128,-1.98982658543039,
26.));
#57669=CARTESIAN_POINT('Ctrl Pts',(-4.05169949925962,-1.96391048284628,
26.));
#57670=CARTESIAN_POINT('Ctrl Pts',(-4.06596584566683,-1.93784746217908,
26.));
#57671=CARTESIAN_POINT('Ctrl Pts',(-4.07831325232761,-1.91529012999318,
26.));
#57672=CARTESIAN_POINT('Ctrl Pts',(-4.09048280358417,-1.89261955019595,
26.));
#57673=CARTESIAN_POINT('Ctrl Pts',(-4.10246124623198,-1.86986160408455,
26.));
#57674=CARTESIAN_POINT('Ctrl Pts',(-4.16682782765767,-1.74757098296373,
26.));
#57675=CARTESIAN_POINT('Ctrl Pts',(-4.22575033277333,-1.62263418183686,
26.));
#57676=CARTESIAN_POINT('Ctrl Pts',(-4.27912376767658,-1.49549834075104,
26.));
#57677=CARTESIAN_POINT('Ctrl Pts',(-4.333101839857,-1.36692225005554,26.));
#57678=CARTESIAN_POINT('Ctrl Pts',(-4.38140486252481,-1.23609633060621,
26.));
#57679=CARTESIAN_POINT('Ctrl Pts',(-4.42388482122499,-1.10344716235086,
26.));
#57680=CARTESIAN_POINT('Ctrl Pts',(-4.46661826556875,-0.970006452370537,
26.));
#57681=CARTESIAN_POINT('Ctrl Pts',(-4.50345940350737,-0.83471991605117,
26.));
#57682=CARTESIAN_POINT('Ctrl Pts',(-4.53421101307421,-0.697996575960625,
26.));
#57683=CARTESIAN_POINT('Ctrl Pts',(-4.55727472024934,-0.595454070892716,
26.));
#57684=CARTESIAN_POINT('Ctrl Pts',(-4.57691215392772,-0.492102769524819,
26.));
#57685=CARTESIAN_POINT('Ctrl Pts',(-4.59302069983613,-0.388109915197262,
26.));
#57686=CARTESIAN_POINT('Ctrl Pts',(-4.59983051322201,-0.344147416318648,
26.));
#57687=CARTESIAN_POINT('Ctrl Pts',(-4.60600945165704,-0.300070227388598,
26.));
#57688=CARTESIAN_POINT('Ctrl Pts',(-4.61154878947915,-0.25589088056297,
26.));
#57689=CARTESIAN_POINT('Ctrl Pts',(-4.6146089290101,-0.231484539947162,
26.));
#57690=CARTESIAN_POINT('Ctrl Pts',(-4.61747426508659,-0.207042538674214,
26.));
#57691=CARTESIAN_POINT('Ctrl Pts',(-4.62014035545176,-0.182595807090288,
26.));
#57692=CARTESIAN_POINT('Ctrl Pts',(-4.6355064624287,-0.0416961970611351,
26.));
#57693=CARTESIAN_POINT('Ctrl Pts',(-4.64428121342256,0.099526957690747,
26.));
#57694=CARTESIAN_POINT('Ctrl Pts',(-4.64631642071577,0.240645210364403,
26.));
#57695=CARTESIAN_POINT('Ctrl Pts',(-4.64782495501833,0.345244739654039,
26.));
#57696=CARTESIAN_POINT('Ctrl Pts',(-4.64562987589745,0.449787288147385,
26.));
#57697=CARTESIAN_POINT('Ctrl Pts',(-4.6396534459514,0.554104703798643,26.));
#57698=CARTESIAN_POINT('Ctrl Pts',(-4.63179775743763,0.691224210145253,
26.));
#57699=CARTESIAN_POINT('Ctrl Pts',(-4.61741097334291,0.827954978565883,
26.));
#57700=CARTESIAN_POINT('Ctrl Pts',(-4.59676076751363,0.963919018344825,
26.));
#57701=CARTESIAN_POINT('Ctrl Pts',(-4.57581741441672,1.1018131835223,26.));
#57702=CARTESIAN_POINT('Ctrl Pts',(-4.54843137134414,1.23891944459888,26.));
#57703=CARTESIAN_POINT('Ctrl Pts',(-4.51482841662203,1.3748401921847,26.));
#57704=CARTESIAN_POINT('Ctrl Pts',(-4.50509310232456,1.41421861019102,26.));
#57705=CARTESIAN_POINT('Ctrl Pts',(-4.49483564045414,1.45349746044631,26.));
#57706=CARTESIAN_POINT('Ctrl Pts',(-4.48406073341117,1.49266688179373,26.));
#57707=CARTESIAN_POINT('Ctrl Pts',(-4.47783668509381,1.51529281908091,26.));
#57708=CARTESIAN_POINT('Ctrl Pts',(-4.47143997379187,1.53788224103568,26.));
#57709=CARTESIAN_POINT('Ctrl Pts',(-4.46487145429867,1.56043322804307,26.));
#57710=CARTESIAN_POINT('Ctrl Pts',(-4.45973334069111,1.57807335734872,26.));
#57711=CARTESIAN_POINT('Ctrl Pts',(-4.45449021537901,1.59568938184522,26.));
#57712=CARTESIAN_POINT('Ctrl Pts',(-4.44914654369818,1.61326759097873,26.));
#57713=CARTESIAN_POINT('Ctrl Pts',(-4.40827604464057,1.7477126360219,26.));
#57714=CARTESIAN_POINT('Ctrl Pts',(-4.36147201478811,1.88014056905998,26.));
#57715=CARTESIAN_POINT('Ctrl Pts',(-4.30904356529584,2.01016709268461,26.));
#57716=CARTESIAN_POINT('Ctrl Pts',(-4.25484746504965,2.14457752399178,26.));
#57717=CARTESIAN_POINT('Ctrl Pts',(-4.19464124103037,2.27642270082558,26.));
#57718=CARTESIAN_POINT('Ctrl Pts',(-4.12870910753944,2.4052752225727,26.));
#57719=CARTESIAN_POINT('Ctrl Pts',(-4.06277697404851,2.53412774431982,26.));
#57720=CARTESIAN_POINT('Ctrl Pts',(-3.991118562445,2.65998845878048,26.));
#57721=CARTESIAN_POINT('Ctrl Pts',(-3.91396546539836,2.78241449550764,26.));
#57722=CARTESIAN_POINT('Ctrl Pts',(-3.8599022254897,2.86820169586649,26.));
#57723=CARTESIAN_POINT('Ctrl Pts',(-3.80313988532888,2.95230207537908,26.));
#57724=CARTESIAN_POINT('Ctrl Pts',(-3.74376497539126,3.03461721426763,26.));
#57725=CARTESIAN_POINT('Ctrl Pts',(-3.71778845229355,3.07063008753137,26.));
#57726=CARTESIAN_POINT('Ctrl Pts',(-3.69131172751679,3.10630115823714,26.));
#57727=CARTESIAN_POINT('Ctrl Pts',(-3.66434142116742,3.1416216999591,26.));
#57728=CARTESIAN_POINT('Ctrl Pts',(-3.64886736739569,3.16188665189447,26.));
#57729=CARTESIAN_POINT('Ctrl Pts',(-3.63323082853231,3.18203621015477,26.));
#57730=CARTESIAN_POINT('Ctrl Pts',(-3.61743300165625,3.20206867796743,26.));
#57731=CARTESIAN_POINT('Ctrl Pts',(-3.60562290128194,3.21704450074792,26.));
#57732=CARTESIAN_POINT('Ctrl Pts',(-3.59372248215876,3.23195501636103,26.));
#57733=CARTESIAN_POINT('Ctrl Pts',(-3.58174179779154,3.24678792441536,26.));
#57734=CARTESIAN_POINT('Ctrl Pts',(-3.49102566491969,3.35910071195637,26.));
#57735=CARTESIAN_POINT('Ctrl Pts',(-3.39558140635013,3.46713215575717,26.));
#57736=CARTESIAN_POINT('Ctrl Pts',(-3.29573453983928,3.57065014592309,26.));
#57737=CARTESIAN_POINT('Ctrl Pts',(-3.19481521819522,3.67528002275919,26.));
#57738=CARTESIAN_POINT('Ctrl Pts',(-3.08939783097439,3.77529957447928,26.));
#57739=CARTESIAN_POINT('Ctrl Pts',(-2.97977151694561,3.87044492257043,26.));
#57740=CARTESIAN_POINT('Ctrl Pts',(-2.87044051512184,3.9653339673936,26.));
#57741=CARTESIAN_POINT('Ctrl Pts',(-2.75692276267532,4.05537559850027,26.));
#57742=CARTESIAN_POINT('Ctrl Pts',(-2.63946507568592,4.14027538885812,26.));
#57743=CARTESIAN_POINT('Ctrl Pts',(-2.52377549108901,4.22389717412067,26.));
#57744=CARTESIAN_POINT('Ctrl Pts',(-2.40426319127569,4.30253122094905,26.));
#57745=CARTESIAN_POINT('Ctrl Pts',(-2.28113248745318,4.37585694114117,26.));
#57746=CARTESIAN_POINT('Ctrl Pts',(-2.24413725288456,4.39788801977718,26.));
#57747=CARTESIAN_POINT('Ctrl Pts',(-2.20681518281834,4.41943960051781,26.));
#57748=CARTESIAN_POINT('Ctrl Pts',(-2.16917135428626,4.44050218283292,26.));
#57749=CARTESIAN_POINT('Ctrl Pts',(-2.54472725763282,-3.56250530678316,
26.));
#57750=CARTESIAN_POINT('Ctrl Pts',(-1.44818804155806,-4.33531677513798,
26.0490642110999));
#57751=CARTESIAN_POINT('Ctrl Pts',(1.63914523023693,-4.84388073813931,26.1510486762817));
#57752=CARTESIAN_POINT('Ctrl Pts',(4.98187809541805,-1.36671674862893,26.3059533955455));
#57753=CARTESIAN_POINT('Ctrl Pts',(3.85252000415521,3.44398917781397,26.4647141577913));
#57754=CARTESIAN_POINT('Ctrl Pts',(-0.805001512196143,5.10466442465425,
26.6234749200372));
#57755=CARTESIAN_POINT('Ctrl Pts',(-3.96413630374849,2.67678406505067,26.7514334980751));
#57756=CARTESIAN_POINT('Ctrl Pts',(-4.3679444184666,0.611489669763926,26.826471822031));
#57757=CARTESIAN_POINT('Ctrl Pts',(-4.36558297706963,0.00185075076461511,
26.848589891905));
#57758=CARTESIAN_POINT('Origin',(0.,0.,24.1514101080949));
#57759=CARTESIAN_POINT('',(2.5383587572269,-3.55965150255042,26.));
#57760=CARTESIAN_POINT('Origin',(0.,0.,26.));
#57761=CARTESIAN_POINT('Ctrl Pts',(2.53835875722654,-3.55965150255068,26.));
#57762=CARTESIAN_POINT('Ctrl Pts',(3.13016463613492,-3.13763950664917,26.026460127041));
#57763=CARTESIAN_POINT('Ctrl Pts',(4.08944058768451,-1.99447514282845,26.079380381123));
#57764=CARTESIAN_POINT('Ctrl Pts',(4.72633908941221,0.949051473338421,26.1852208892869));
#57765=CARTESIAN_POINT('Ctrl Pts',(2.60449620246589,4.46265906441401,26.3175215244918));
#57766=CARTESIAN_POINT('Ctrl Pts',(-2.34489469821123,4.60777770546463,26.4762822867377));
#57767=CARTESIAN_POINT('Ctrl Pts',(-4.30346090622908,1.74883727013167,26.5875784812721));
#57768=CARTESIAN_POINT('Ctrl Pts',(-4.3779262327693,0.151632086931482,26.6459544217245));
#57769=CARTESIAN_POINT('Ctrl Pts',(-4.37688026104952,0.00226901643694839,
26.651410108095));
#57770=CARTESIAN_POINT('Ctrl Pts',(2.86929757049756,-4.02374147429191,25.6709103465619));
#57771=CARTESIAN_POINT('Ctrl Pts',(3.53826020854994,-3.54670961616163,25.6973704736029));
#57772=CARTESIAN_POINT('Ctrl Pts',(4.62260187198943,-2.25450506767067,25.7502907276849));
#57773=CARTESIAN_POINT('Ctrl Pts',(5.34253608871791,1.0727841677129,25.8561312358488));
#57774=CARTESIAN_POINT('Ctrl Pts',(2.94405769272283,5.04447875030544,25.9884318710537));
#57775=CARTESIAN_POINT('Ctrl Pts',(-2.65061061266289,5.20851725077882,26.1471926332996));
#57776=CARTESIAN_POINT('Ctrl Pts',(-5.80869481541901,0.598627327994403,
26.3059533955455));
#57777=CARTESIAN_POINT('Ctrl Pts',(-3.6559591721986,-4.55561486272761,26.4647141577913));
#57778=CARTESIAN_POINT('Ctrl Pts',(1.84567034813922,-5.54225209737284,26.6234749200373));
#57779=CARTESIAN_POINT('Ctrl Pts',(5.65659992177503,-1.45549501989441,26.7822356822831));
#57780=CARTESIAN_POINT('Ctrl Pts',(4.29121225256454,3.96287657984353,26.940996444529));
#57781=CARTESIAN_POINT('Ctrl Pts',(-1.00202899277672,5.75456300236789,27.0997572067749));
#57782=CARTESIAN_POINT('Ctrl Pts',(-5.37797121296738,2.27936156876184,27.2585179690208));
#57783=CARTESIAN_POINT('Ctrl Pts',(-4.83194032779028,-3.28191017660925,
27.4172787312667));
#57784=CARTESIAN_POINT('Ctrl Pts',(0.136487592633803,-5.83951456248522,
27.5760394935126));
#57785=CARTESIAN_POINT('Ctrl Pts',(4.97996779668276,-3.05259748930662,27.7348002557585));
#57786=CARTESIAN_POINT('Ctrl Pts',(5.26564507543792,2.52813993990873,27.8935610180044));
#57787=CARTESIAN_POINT('Ctrl Pts',(0.732034933496452,5.79505175124635,28.0523217802503));
#57788=CARTESIAN_POINT('Ctrl Pts',(-4.47155165508331,3.75815243181214,28.2110825424962));
#57789=CARTESIAN_POINT('Ctrl Pts',(-5.58263982081247,-1.71832134856424,
28.369843304742));
#57790=CARTESIAN_POINT('Ctrl Pts',(-1.58432433047622,-5.62213569522022,
28.5286040669879));
#57791=CARTESIAN_POINT('Ctrl Pts',(3.86401257103054,-4.38039933096899,28.6873648292338));
#57792=CARTESIAN_POINT('Ctrl Pts',(5.77588745817332,0.870412097209825,28.8461255914797));
#57793=CARTESIAN_POINT('Ctrl Pts',(2.40149355054825,5.32459589387785,29.0048863537256));
#57794=CARTESIAN_POINT('Ctrl Pts',(-3.17082052230127,4.90554683073371,29.1636471159715));
#57795=CARTESIAN_POINT('Ctrl Pts',(-5.84110284449404,-0.00320850462351047,
29.3224078782174));
#57796=CARTESIAN_POINT('Ctrl Pts',(-3.16542940092975,-4.90902733376601,
29.4811686404633));
#57797=CARTESIAN_POINT('Ctrl Pts',(2.40734170730851,-5.32195439090584,29.6399294027091));
#57798=CARTESIAN_POINT('Ctrl Pts',(5.77684015826,-0.8640662324248,29.7986901649551));
#57799=CARTESIAN_POINT('Ctrl Pts',(3.85919803712304,4.38464173738479,29.9574509272009));
#57800=CARTESIAN_POINT('Ctrl Pts',(-1.59050000656898,5.62039165738282,30.1162116894468));
#57801=CARTESIAN_POINT('Ctrl Pts',(-5.58452386271215,1.71218745603623,30.2749724516927));
#57802=CARTESIAN_POINT('Ctrl Pts',(-4.46742089771919,-3.76306300482994,
30.4337332139386));
#57803=CARTESIAN_POINT('Ctrl Pts',(0.738402131764131,-5.79424325925859,
30.5924939761845));
#57804=CARTESIAN_POINT('Ctrl Pts',(5.26841697560084,-2.522355095433,30.7512547384304));
#57805=CARTESIAN_POINT('Ctrl Pts',(4.97661567740753,3.05806949811635,30.9100155006762));
#57806=CARTESIAN_POINT('Ctrl Pts',(0.130063698581311,5.83965547701761,31.0687762629222));
#57807=CARTESIAN_POINT('Ctrl Pts',(-4.83552655005252,3.27661038876524,31.227537025168));
#57808=CARTESIAN_POINT('Ctrl Pts',(-5.37549519698693,-2.28528861265885,
31.386297787414));
#57809=CARTESIAN_POINT('Ctrl Pts',(-0.995646443005195,-5.75562167072471,
31.5450585496598));
#57810=CARTESIAN_POINT('Ctrl Pts',(4.2954483480341,-3.95823396799194,31.7038193119058));
#57811=CARTESIAN_POINT('Ctrl Pts',(5.65521760477304,1.46185036807875,31.8625800741516));
#57812=CARTESIAN_POINT('Ctrl Pts',(1.83915896875347,5.54400459448242,32.0213408363975));
#57813=CARTESIAN_POINT('Ctrl Pts',(-3.66015413331184,4.5521164721907,32.1801015986434));
#57814=CARTESIAN_POINT('Ctrl Pts',(-5.80958237170622,-0.606007691658192,
32.3388623608893));
#57815=CARTESIAN_POINT('Ctrl Pts',(-2.64190336751104,-5.20949510535547,
32.4976231231352));
#57816=CARTESIAN_POINT('Ctrl Pts',(2.9437262966194,-5.04509347253155,32.6563838853811));
#57817=CARTESIAN_POINT('Ctrl Pts',(5.83516773679323,-0.263268189260048,
32.8151446476269));
#57818=CARTESIAN_POINT('Ctrl Pts',(3.3860854267346,4.75950818245377,32.9739054098728));
#57819=CARTESIAN_POINT('Ctrl Pts',(-2.1620456951976,5.42623728451552,33.1326661721187));
#57820=CARTESIAN_POINT('Ctrl Pts',(-5.73140655633933,1.12670827721268,33.2914269343647));
#57821=CARTESIAN_POINT('Ctrl Pts',(-4.0552090690265,-4.20401856114767,33.4501876966105));
#57822=CARTESIAN_POINT('Ctrl Pts',(1.33243962623321,-5.68709919892666,33.6089484588564));
#57823=CARTESIAN_POINT('Ctrl Pts',(5.50059887566598,-1.96517293514109,33.7677092211022));
#57824=CARTESIAN_POINT('Ctrl Pts',(4.63444201610888,3.55533962587452,33.9264699833482));
#57825=CARTESIAN_POINT('Ctrl Pts',(-0.473297737465698,5.82189676202686,
34.0852307455941));
#57826=CARTESIAN_POINT('Ctrl Pts',(-5.14786094464401,2.7600761494201,34.24399150784));
#57827=CARTESIAN_POINT('Ctrl Pts',(-5.11094457182416,-2.82785046275963,
34.4027522700858));
#57828=CARTESIAN_POINT('Ctrl Pts',(-0.396335611036177,-5.82764195360469,
34.5615130323317));
#57829=CARTESIAN_POINT('Ctrl Pts',(4.68101180720102,-3.49379752086946,34.7202737945776));
#57830=CARTESIAN_POINT('Ctrl Pts',(5.47415423612042,2.03767712240033,34.8790345568235));
#57831=CARTESIAN_POINT('Ctrl Pts',(1.2571834979241,5.7042074215912,35.0377953190694));
#57832=CARTESIAN_POINT('Ctrl Pts',(-4.11039997874232,4.15007285125745,35.1965560813153));
#57833=CARTESIAN_POINT('Ctrl Pts',(-5.71601984106162,-1.20233515817297,
35.3553168435612));
#57834=CARTESIAN_POINT('Ctrl Pts',(-2.09016374674189,-5.45432930503785,
35.5140776058071));
#57835=CARTESIAN_POINT('Ctrl Pts',(3.44867405347895,-4.71435466727419,35.6728383680529));
#57836=CARTESIAN_POINT('Ctrl Pts',(5.8311800188353,0.340341363817132,35.8315991302989));
#57837=CARTESIAN_POINT('Ctrl Pts',(2.87681191524069,5.0835465828807,35.9903598925447));
#57838=CARTESIAN_POINT('Ctrl Pts',(-2.7105023265463,5.17413469033962,36.1491206547906));
#57839=CARTESIAN_POINT('Ctrl Pts',(-5.81708204570653,0.529196683197753,
36.3078814170365));
#57840=CARTESIAN_POINT('Ctrl Pts',(-3.5996905915515,-4.60007829292986,36.4666421792824));
#57841=CARTESIAN_POINT('Ctrl Pts',(1.91224764597227,-5.51922110414707,36.6254029415283));
#57842=CARTESIAN_POINT('Ctrl Pts',(5.67403842753732,-1.38700417404515,36.7841637037742));
#57843=CARTESIAN_POINT('Ctrl Pts',(4.24277592445978,4.01464134273703,36.9429244660201));
#57844=CARTESIAN_POINT('Ctrl Pts',(-1.07160470196143,5.74196447382976,37.1016852282659));
#57845=CARTESIAN_POINT('Ctrl Pts',(-5.40521997255572,2.2140663278849,37.2604459905119));
#57846=CARTESIAN_POINT('Ctrl Pts',(-4.79181281967314,-3.34021295087678,
37.4192067527577));
#57847=CARTESIAN_POINT('Ctrl Pts',(0.207207793602656,-5.83742730886296,
37.5779675150036));
#57848=CARTESIAN_POINT('Ctrl Pts',(5.01658550492884,-2.99204988723897,37.7367282772495));
#57849=CARTESIAN_POINT('Ctrl Pts',(5.23463092854471,2.59174298453994,37.8954890394954));
#57850=CARTESIAN_POINT('Ctrl Pts',(0.661782232472825,5.80349351104764,38.0542498017413));
#57851=CARTESIAN_POINT('Ctrl Pts',(-4.51674977715968,3.70370950622708,38.2130105639872));
#57852=CARTESIAN_POINT('Ctrl Pts',(-5.5614144248173,-1.78582256997244,38.371771326233));
#57853=CARTESIAN_POINT('Ctrl Pts',(-1.51610271526659,-5.64091528147253,
38.530532088479));
#57854=CARTESIAN_POINT('Ctrl Pts',(3.91679250925652,-4.33327002336813,38.6892928507249));
#57855=CARTESIAN_POINT('Ctrl Pts',(5.76491958932306,0.940316321579044,38.8480536129708));
#57856=CARTESIAN_POINT('Ctrl Pts',(2.33681616947948,5.35329644668107,39.0068143752167));
#57857=CARTESIAN_POINT('Ctrl Pts',(-3.23001278765103,4.86677614521149,39.1655751374625));
#57858=CARTESIAN_POINT('Ctrl Pts',(-5.84063537949807,-0.0739663419686063,
39.3243358997085));
#57859=CARTESIAN_POINT('Ctrl Pts',(-3.10573006749788,-4.94701257364771,
39.4830966619543));
#57860=CARTESIAN_POINT('Ctrl Pts',(2.47163426803653,-5.29240178945783,39.6418574242002));
#57861=CARTESIAN_POINT('Ctrl Pts',(5.78688342441216,-0.794023229038551,
39.8006181864461));
#57862=CARTESIAN_POINT('Ctrl Pts',(3.80580010810998,4.43106964435213,39.959378948692));
#57863=CARTESIAN_POINT('Ctrl Pts',(-1.65846771681237,5.60071223044711,40.1181397109378));
#57864=CARTESIAN_POINT('Ctrl Pts',(-5.60485522875205,1.64441190725433,40.2769004731838));
#57865=CARTESIAN_POINT('Ctrl Pts',(-4.4215080328057,-3.81690442267336,40.4356612354296));
#57866=CARTESIAN_POINT('Ctrl Pts',(0.808538371485783,-5.78487323610672,
40.5944219976756));
#57867=CARTESIAN_POINT('Ctrl Pts',(5.29858576106737,-2.45834936260147,40.7531827599214));
#57868=CARTESIAN_POINT('Ctrl Pts',(4.93920561471065,3.1181309388157,40.9119435221673));
#57869=CARTESIAN_POINT('Ctrl Pts',(0.0593136197707885,5.84080256047905,
41.0707042844132));
#57870=CARTESIAN_POINT('Ctrl Pts',(-4.87486401174139,3.21779326915472,41.2294650466591));
#57871=CARTESIAN_POINT('Ctrl Pts',(-5.34741719504777,-2.35023871087517,
41.388225808905));
#57872=CARTESIAN_POINT('Ctrl Pts',(-0.925850822461446,-5.76726043373597,
41.5469865711509));
#57873=CARTESIAN_POINT('Ctrl Pts',(4.34308250332321,-3.90590924437788,41.7057473333967));
#57874=CARTESIAN_POINT('Ctrl Pts',(5.63709406088405,1.53024939298615,41.8645080956427));
#57875=CARTESIAN_POINT('Ctrl Pts',(1.77186494664376,5.56587704381296,42.0232688578886));
#57876=CARTESIAN_POINT('Ctrl Pts',(-3.71502908908446,4.50744401221416,42.1820296201344));
#57877=CARTESIAN_POINT('Ctrl Pts',(-5.80181502544146,-0.676339461033121,
42.3407903823803));
#57878=CARTESIAN_POINT('Ctrl Pts',(-2.57860263176698,-5.24111640048504,
42.4995511446262));
#57879=CARTESIAN_POINT('Ctrl Pts',(3.00462565494359,-5.00906351822809,42.6583119068721));
#57880=CARTESIAN_POINT('Ctrl Pts',(5.83792876476416,-0.192562700251437,
42.817072669118));
#57881=CARTESIAN_POINT('Ctrl Pts',(3.32818114721658,4.80017738289961,42.9758334313639));
#57882=CARTESIAN_POINT('Ctrl Pts',(-2.22761951688042,5.39964850189364,43.1345941936098));
#57883=CARTESIAN_POINT('Ctrl Pts',(-5.74463475560437,1.05719637754358,43.2933549558557));
#57884=CARTESIAN_POINT('Ctrl Pts',(-4.0039847938458,-4.25283416401821,43.4521157181015));
#57885=CARTESIAN_POINT('Ctrl Pts',(1.40123435454846,-5.67054097415953,43.6108764803475));
#57886=CARTESIAN_POINT('Ctrl Pts',(5.5240010203993,-1.89839547582067,43.7696372425933));
#57887=CARTESIAN_POINT('Ctrl Pts',(4.59103321957251,3.61121954923408,43.9283980048393));
#57888=CARTESIAN_POINT('Ctrl Pts',(-0.543788418742688,5.81573613669244,
44.0871587670851));
#57889=CARTESIAN_POINT('Ctrl Pts',(-5.18091828599107,2.69751336787648,44.245919529331));
#57890=CARTESIAN_POINT('Ctrl Pts',(-5.07631348469077,-2.88955603183869,
44.4046802915769));
#57891=CARTESIAN_POINT('Ctrl Pts',(-0.325711524187161,-5.83201548857688,
44.5634410538228));
#57892=CARTESIAN_POINT('Ctrl Pts',(4.7229915722406,-3.43683622893689,44.7222018160687));
#57893=CARTESIAN_POINT('Ctrl Pts',(5.44906851609775,2.1038405269557,44.8809625783145));
#57894=CARTESIAN_POINT('Ctrl Pts',(1.18799151005716,5.71901816993276,45.0397233405605));
#57895=CARTESIAN_POINT('Ctrl Pts',(-4.16037161366087,4.09997569410277,45.1984841028063));
#57896=CARTESIAN_POINT('Ctrl Pts',(-5.70103555635091,-1.27148977235826,
45.3572448650522));
#57897=CARTESIAN_POINT('Ctrl Pts',(-2.02393761747008,-5.47924896099626,
45.5160056272981));
#57898=CARTESIAN_POINT('Ctrl Pts',(3.50552985089882,-4.67223213469171,45.674766389544));
#57899=CARTESIAN_POINT('Ctrl Pts',(5.82662932192163,0.410954256471436,45.8335271517899));
#57900=CARTESIAN_POINT('Ctrl Pts',(2.81501966081174,5.11802275935076,45.9922879140358));
#57901=CARTESIAN_POINT('Ctrl Pts',(-2.77298197976823,5.1409205008315,46.1510486762817));
#57902=CARTESIAN_POINT('Ctrl Pts',(-5.82306581062682,0.458690768489886,
46.3098094385276));
#57903=CARTESIAN_POINT('Ctrl Pts',(-3.54370194373858,-4.64334676606566,
46.4685702007734));
#57904=CARTESIAN_POINT('Ctrl Pts',(1.97896618584451,-5.49565150744413,46.6273309630194));
#57905=CARTESIAN_POINT('Ctrl Pts',(5.69042401383344,-1.31816812234872,46.7860917252652));
#57906=CARTESIAN_POINT('Ctrl Pts',(4.19383196809736,4.0657429922898,46.9448524875111));
#57907=CARTESIAN_POINT('Ctrl Pts',(-1.14108319710691,5.72856193064797,47.103613249757));
#57908=CARTESIAN_POINT('Ctrl Pts',(-5.4316441654788,2.14842600887457,47.2623740120029));
#57909=CARTESIAN_POINT('Ctrl Pts',(-4.75099848187323,-3.39801502074773,
47.4211347742488));
#57910=CARTESIAN_POINT('Ctrl Pts',(0.277906133480956,-5.83448890966147,
47.5798955364947));
#57911=CARTESIAN_POINT('Ctrl Pts',(5.05246256671996,-2.93106033166876,47.7386562987406));
#57912=CARTESIAN_POINT('Ctrl Pts',(5.20285092941832,2.65496419227074,47.8974170609865));
#57913=CARTESIAN_POINT('Ctrl Pts',(0.591431198362095,5.8110843905069,48.0561778232323));
#57914=CARTESIAN_POINT('Ctrl Pts',(-4.56128443093633,3.6487226526672,48.2149385854782));
#57915=CARTESIAN_POINT('Ctrl Pts',(-5.53937322279471,-1.85306150857812,
48.3736993477241));
#57916=CARTESIAN_POINT('Ctrl Pts',(-1.44765843879317,-5.65886717467194,
48.53246010997));
#57917=CARTESIAN_POINT('Ctrl Pts',(3.96899756769466,-4.28550475015754,48.6912208722159));
#57918=CARTESIAN_POINT('Ctrl Pts',(5.75310576561908,1.01008252414809,48.8499816344618));
#57919=CARTESIAN_POINT('Ctrl Pts',(2.27179583594514,5.38121141898098,49.0087423967076));
#57920=CARTESIAN_POINT('Ctrl Pts',(-3.28873103569315,4.8272912519194,49.1675031589537));
#57921=CARTESIAN_POINT('Ctrl Pts',(-5.83931080786754,-0.144713320429998,
49.3262639211994));
#57922=CARTESIAN_POINT('Ctrl Pts',(-3.04557496461057,-4.98427184159595,
49.4850246834454));
#57923=CARTESIAN_POINT('Ctrl Pts',(2.53556411455661,-5.26207252676754,49.6437854456913));
#57924=CARTESIAN_POINT('Ctrl Pts',(5.79607746626723,-0.72386370334331,49.8025462079371));
#57925=CARTESIAN_POINT('Ctrl Pts',(3.75184367735869,4.47684729208542,49.961306970183));
#57926=CARTESIAN_POINT('Ctrl Pts',(-1.72619204662586,5.58021089871651,50.120067732429));
#57927=CARTESIAN_POINT('Ctrl Pts',(-5.62436408231579,1.57639504108098,50.2788284946748));
#57928=CARTESIAN_POINT('Ctrl Pts',(-4.37494631143252,-3.87018570976535,
50.4375892569207));
#57929=CARTESIAN_POINT('Ctrl Pts',(0.878555958148904,-5.77465428267269,
50.5963500191666));
#57930=CARTESIAN_POINT('Ctrl Pts',(5.32797697899131,-2.39398286696617,50.7551107814125));
#57931=CARTESIAN_POINT('Ctrl Pts',(4.90107072348494,3.17773479374659,50.9138715436583));
#57932=CARTESIAN_POINT('Ctrl Pts',(-0.0114451633093337,5.84109250604932,
51.0726323059043));
#57933=CARTESIAN_POINT('Ctrl Pts',(-4.91348608704586,3.15850393832203,51.2313930681501));
#57934=CARTESIAN_POINT('Ctrl Pts',(-5.31855445953128,-2.4148439115166,51.3901538303961));
#57935=CARTESIAN_POINT('Ctrl Pts',(-0.855919333292373,-5.77805285116754,
51.5489145926419));
#57936=CARTESIAN_POINT('Ctrl Pts',(4.39007931117216,-3.85301132850749,51.7076753548878));
#57937=CARTESIAN_POINT('Ctrl Pts',(5.61814327333331,1.59842385376603,51.8664361171337));
#57938=CARTESIAN_POINT('Ctrl Pts',(1.70431090331913,5.58693270058057,52.0251968793796));
#57939=CARTESIAN_POINT('Ctrl Pts',(-3.76935886426715,4.46211008474238,52.1839576416255));
#57940=CARTESIAN_POINT('Ctrl Pts',(-5.79319626271042,-0.746571977579234,
52.3427184038713));
#57941=CARTESIAN_POINT('Ctrl Pts',(-2.51492348603726,-5.27196856168236,
52.5014791661173));
#57942=CARTESIAN_POINT('Ctrl Pts',(3.06508408439537,-4.9722984837573,52.6602399283631));
#57943=CARTESIAN_POINT('Ctrl Pts',(5.83983307657691,-0.121828952662795,
52.8190006906091));
#57944=CARTESIAN_POINT('Ctrl Pts',(3.26978845705136,4.84014215722252,52.9777614528549));
#57945=CARTESIAN_POINT('Ctrl Pts',(-2.29286643535651,5.37226732075056,53.1365222151009));
#57946=CARTESIAN_POINT('Ctrl Pts',(-5.75701992960891,0.98752933428568,53.2952829773466));
#57947=CARTESIAN_POINT('Ctrl Pts',(-3.95217293381976,-4.30102566339373,
53.4540437395927));
#57948=CARTESIAN_POINT('Ctrl Pts',(1.46982345169535,-5.65315059739567,53.6128045018384));
#57949=CARTESIAN_POINT('Ctrl Pts',(5.54659251787697,-1.83133942692776,53.7715652640845));
#57950=CARTESIAN_POINT('Ctrl Pts',(4.54695068882314,3.66656952605562,53.9303260263302));
#57951=CARTESIAN_POINT('Ctrl Pts',(-0.61419929905889,5.80872205196845,54.0890867885762));
#57952=CARTESIAN_POINT('Ctrl Pts',(-5.21321532748033,2.63455472619438,54.2478475508221));
#57953=CARTESIAN_POINT('Ctrl Pts',(-5.04093744845616,-2.95083755851469,
54.4066083130679));
#57954=CARTESIAN_POINT('Ctrl Pts',(-0.255039639165707,-5.8355331751643,
54.5653690753139));
#57955=CARTESIAN_POINT('Ctrl Pts',(4.76427823817645,-3.37937058122179,54.7241298375597));
#57956=CARTESIAN_POINT('Ctrl Pts',(5.42318314516584,2.16969519287334,54.8828905998057));
#57957=CARTESIAN_POINT('Ctrl Pts',(1.11862518441343,5.7329896522482,55.0416513620514));
#57958=CARTESIAN_POINT('Ctrl Pts',(-4.20973271396536,4.04927686543645,55.2004121242976));
#57959=CARTESIAN_POINT('Ctrl Pts',(-5.68521464456297,-1.34045779539507,
55.3591728865431));
#57960=CARTESIAN_POINT('Ctrl Pts',(-1.95741447531414,-5.50336453706454,
55.5179336487893));
#57961=CARTESIAN_POINT('Ctrl Pts',(3.56187121174587,-4.62942395195395,55.676694411035));
#57962=CARTESIAN_POINT('Ctrl Pts',(5.82122356704326,0.481506841580768,55.835455173281));
#57963=CARTESIAN_POINT('Ctrl Pts',(2.75281430219354,5.15174786588276,55.9942159355268));
#57964=CARTESIAN_POINT('Ctrl Pts',(-2.83505469783139,5.10695188114131,56.1529766977728));
#57965=CARTESIAN_POINT('Ctrl Pts',(-5.82819504052776,0.388117540903014,
56.3117374600186));
#57966=CARTESIAN_POINT('Ctrl Pts',(-3.48719325759759,-4.6859338279744,56.4704982222645));
#57967=CARTESIAN_POINT('Ctrl Pts',(2.04539431239091,-5.47127542377716,56.6292589845104));
#57968=CARTESIAN_POINT('Ctrl Pts',(5.70597453029646,-1.24913862945516,56.7880197467563));
#57969=CARTESIAN_POINT('Ctrl Pts',(4.14427256681325,4.11624799398041,56.9467805090021));
#57970=CARTESIAN_POINT('Ctrl Pts',(-1.21039423827122,5.71431872089305,57.1055412712481));
#57971=CARTESIAN_POINT('Ctrl Pts',(-5.4572712645165,2.08247040830632,57.2643020334939));
#57972=CARTESIAN_POINT('Ctrl Pts',(-4.709486934955,-3.45531843184919,57.4230627957399));
#57973=CARTESIAN_POINT('Ctrl Pts',(0.348563690628765,-5.8306942991006,57.5818235579858));
#57974=CARTESIAN_POINT('Ctrl Pts',(5.08759817953255,-2.86964064293877,57.7405843202316));
#57975=CARTESIAN_POINT('Ctrl Pts',(5.17030741181829,2.71779578395536,57.8993450824775));
#57976=CARTESIAN_POINT('Ctrl Pts',(0.520993371711727,5.81782249322041,58.0581058447234));
#57977=CARTESIAN_POINT('Ctrl Pts',(-4.60514971613518,3.59320034898822,58.2168666069693));
#57978=CARTESIAN_POINT('Ctrl Pts',(-5.51651911764551,-1.9200285103718,58.3756273692151));
#57979=CARTESIAN_POINT('Ctrl Pts',(-1.37900171841615,-5.67598862900501,
58.5343881314612));
#57980=CARTESIAN_POINT('Ctrl Pts',(4.02062017566359,-4.23711057904269,58.6931488937069));
#57981=CARTESIAN_POINT('Ctrl Pts',(5.74044767353369,1.07970049708729,58.8519096559529));
#57982=CARTESIAN_POINT('Ctrl Pts',(2.20644211632846,5.40833669840192,59.0106704181987));
#57983=CARTESIAN_POINT('Ctrl Pts',(-3.34696666239261,4.78709795354361,59.1694311804446));
#57984=CARTESIAN_POINT('Ctrl Pts',(-5.83712931726406,-0.215439062208749,
59.3281919426906));
#57985=CARTESIAN_POINT('Ctrl Pts',(-2.98497292353889,-5.02079966755579,
59.4869527049364));
#57986=CARTESIAN_POINT('Ctrl Pts',(2.59912186699419,-5.23097105483309,59.6457134671823));
#57987=CARTESIAN_POINT('Ctrl Pts',(5.80442093364305,-0.653597950635783,
59.8044742294282));
#57988=CARTESIAN_POINT('Ctrl Pts',(3.69733666347582,4.52196796239271,59.9632349916741));
#57989=CARTESIAN_POINT('Ctrl Pts',(-1.79366305772334,5.55889067092954,60.1219957539199));
#57990=CARTESIAN_POINT('Ctrl Pts',(-5.64304756034266,1.5081468389052,60.2807565161659));
#57991=CARTESIAN_POINT('Ctrl Pts',(-4.32774256660426,-3.92289904703017,
60.4395172784117));
#57992=CARTESIAN_POINT('Ctrl Pts',(0.948444616708253,-5.76358789861195,
60.5982780406577));
#57993=CARTESIAN_POINT('Ctrl Pts',(5.35658631619137,-2.32926505429939,60.7570388029035));
#57994=CARTESIAN_POINT('Ctrl Pts',(4.86221660003666,3.23687231603548,60.9157995651494));
#57995=CARTESIAN_POINT('Ctrl Pts',(-0.0822022668114812,5.84052527118238,
61.0745603273953));
#57996=CARTESIAN_POINT('Ctrl Pts',(-4.95138710817278,3.09875109697584,61.2333210896412));
#57997=CARTESIAN_POINT('Ctrl Pts',(-5.28891122604591,-2.47909473376766,
61.3920818518871));
#57998=CARTESIAN_POINT('Ctrl Pts',(-0.785862237944882,-5.78799733923239,
61.5508426141331));
#57999=CARTESIAN_POINT('Ctrl Pts',(4.43643187479794,-3.79954798315087,61.7096033763787));
#58000=CARTESIAN_POINT('Ctrl Pts',(5.59836802314956,1.66636374581465,61.8683641386249));
#58001=CARTESIAN_POINT('Ctrl Pts',(1.63650675233685,5.6071684748672,62.0271249008705));
#58002=CARTESIAN_POINT('Ctrl Pts',(-3.82313548596416,4.41612134253018,62.1858856631167));
#58003=CARTESIAN_POINT('Ctrl Pts',(-5.78372734831682,-0.816694934673283,
62.3446464253623));
#58004=CARTESIAN_POINT('Ctrl Pts',(-2.45087527523776,-5.30204706139213,
62.5034071876083));
#58005=CARTESIAN_POINT('Ctrl Pts',(3.12509271269893,-4.93480376438871,62.6621679498542));
#58006=CARTESIAN_POINT('Ctrl Pts',(5.84088039277376,-0.0510773266730637,
62.8209287121001));
#58007=CARTESIAN_POINT('Ctrl Pts',(3.21091592536738,4.879396640591,62.979689474346));
#58008=CARTESIAN_POINT('Ctrl Pts',(-2.35777687563918,5.34409775927519,63.1384502365919));
#58009=CARTESIAN_POINT('Ctrl Pts',(-5.76856026082839,0.917717371079188,
63.2972109988377));
#58010=CARTESIAN_POINT('Ctrl Pts',(-3.89978109233997,-4.34858598717061,
63.4559717610837));
#58011=CARTESIAN_POINT('Ctrl Pts',(1.53819685222249,-5.63493062067332,63.6147325233296));
#58012=CARTESIAN_POINT('Ctrl Pts',(5.56837005279627,-1.76401462893886,63.7734932855754));
#58013=CARTESIAN_POINT('Ctrl Pts',(4.50220089297303,3.72138143372885,63.9322540478213));
#58014=CARTESIAN_POINT('Ctrl Pts',(-0.684520045616047,5.80085553717197,
64.0910148100672));
#58015=CARTESIAN_POINT('Ctrl Pts',(-5.2447473295203,2.57120946355576,64.2497755723131));
#58016=CARTESIAN_POINT('Ctrl Pts',(-5.00482165455439,-3.01168604972238,
64.408536334559));
#58017=CARTESIAN_POINT('Ctrl Pts',(-0.184330327072359,-5.83819449714635,
64.5672970968048));
#58018=CARTESIAN_POINT('Ctrl Pts',(4.80486574618941,-3.32140901080918,64.7260578590508));
#58019=CARTESIAN_POINT('Ctrl Pts',(5.39650192200348,2.23523145597974,64.8848186212967));
#58020=CARTESIAN_POINT('Ctrl Pts',(1.04909470050257,5.74611981822221,65.0435793835425));
#58021=CARTESIAN_POINT('Ctrl Pts',(-4.25847603591327,3.99798380531258,65.2023401457885));
#58022=CARTESIAN_POINT('Ctrl Pts',(-5.66855942741703,-1.40922910622467,
65.3611009080343));
#58023=CARTESIAN_POINT('Ctrl Pts',(-1.8906040825464,-5.52667249428149,65.5198616702802));
#58024=CARTESIAN_POINT('Ctrl Pts',(3.61768986792422,-4.58593640116248,65.6786224325261));
#58025=CARTESIAN_POINT('Ctrl Pts',(5.8149635474948,0.551988765551636,65.8373831947719));
#58026=CARTESIAN_POINT('Ctrl Pts',(2.6902049680239,5.18471695331663,65.996143957018));
#58027=CARTESIAN_POINT('Ctrl Pts',(-2.89671137156331,5.07223381616474,66.1549047192637));
#58028=CARTESIAN_POINT('Ctrl Pts',(-5.83246898269471,0.317487357059558,
66.3136654815097));
#58029=CARTESIAN_POINT('Ctrl Pts',(-3.4301728257792,-4.72783322900402,66.4724262437555));
#58030=CARTESIAN_POINT('Ctrl Pts',(2.11152227728272,-5.44609643033688,66.6311870060015));
#58031=CARTESIAN_POINT('Ctrl Pts',(5.72068769488774,-1.1799258254438,66.7899477682473));
#58032=CARTESIAN_POINT('Ctrl Pts',(4.0941049934505,4.16614893619904,66.9487085304932));
#58033=CARTESIAN_POINT('Ctrl Pts',(-1.27952765405788,5.69923693475624,67.1074692927391));
#58034=CARTESIAN_POINT('Ctrl Pts',(-5.48209750889141,2.01620920516577,67.266230054985));
#58035=CARTESIAN_POINT('Ctrl Pts',(-4.66728427073886,-3.51211477490457,
67.4249908172309));
#58036=CARTESIAN_POINT('Ctrl Pts',(0.419170096048379,-5.82604403403957,
67.5837515794768));
#58037=CARTESIAN_POINT('Ctrl Pts',(5.12198718721476,-2.80779983438927,67.7425123417226));
#58038=CARTESIAN_POINT('Ctrl Pts',(5.13700515150643,2.78022853905663,67.9012731039686));
#58039=CARTESIAN_POINT('Ctrl Pts',(0.45047908927406,5.82370683037148,68.0600338662144));
#58040=CARTESIAN_POINT('Ctrl Pts',(-4.64833919552487,3.53715074308911,68.2187946284603));
#58041=CARTESIAN_POINT('Ctrl Pts',(-5.49285546321007,-1.98671374794472,
68.3775553907063));
#58042=CARTESIAN_POINT('Ctrl Pts',(-1.31014262951052,-5.69227713189796,
68.5363161529521));
#58043=CARTESIAN_POINT('Ctrl Pts',(4.07165275754471,-4.18809461186912,68.6950769151981));
#58044=CARTESIAN_POINT('Ctrl Pts',(5.72694717064212,1.14916002395785,68.8538376774439));
#58045=CARTESIAN_POINT('Ctrl Pts',(2.14076460128891,5.43466830430864,69.0125984396898));
#58046=CARTESIAN_POINT('Ctrl Pts',(-3.40471112167017,4.74620214845141,69.1713592019357));
#58047=CARTESIAN_POINT('Ctrl Pts',(-5.83409122782134,-0.28613318830099,
69.3301199641816));
#58048=CARTESIAN_POINT('Ctrl Pts',(-2.92393283763341,-5.0565906910682,69.4888807264275));
#58049=CARTESIAN_POINT('Ctrl Pts',(2.66229819824794,-5.19910193779603,69.6476414886733));
#58050=CARTESIAN_POINT('Ctrl Pts',(5.81191260213551,-0.583236282416525,
69.8064022509193));
#58051=CARTESIAN_POINT('Ctrl Pts',(3.64228706536681,4.56642503381477,69.9651630131651));
#58052=CARTESIAN_POINT('Ctrl Pts',(-1.86087084873268,5.53675467583008,70.123923775411));
#58053=CARTESIAN_POINT('Ctrl Pts',(-5.66090292103185,1.43967731615189,70.282684537657));
#58054=CARTESIAN_POINT('Ctrl Pts',(-4.27990372547136,-3.97503669878468,
70.4414452999028));
#58055=CARTESIAN_POINT('Ctrl Pts',(1.01819409100193,-5.75167570791655,70.6002060621487));
#58056=CARTESIAN_POINT('Ctrl Pts',(5.38440957424679,-2.26420542194124,70.7589668243946));
#58057=CARTESIAN_POINT('Ctrl Pts',(4.82264894620915,3.29553482724991,70.9177275866405));
#58058=CARTESIAN_POINT('Ctrl Pts',(-0.152947307129394,5.83910093911992,
71.0764883488863));
#58059=CARTESIAN_POINT('Ctrl Pts',(-4.98856151314671,3.03854351384673,71.2352491111322));
#58060=CARTESIAN_POINT('Ctrl Pts',(-5.25849184473667,-2.542981748819,71.3940098733781));
#58061=CARTESIAN_POINT('Ctrl Pts',(-0.71568981729892,-5.79709243857671,
71.5527706356241));
#58062=CARTESIAN_POINT('Ctrl Pts',(4.48213339196102,-3.74552705405491,71.7115313978699));
#58063=CARTESIAN_POINT('Ctrl Pts',(5.57777121235107,1.73405909895161,71.8702921601158));
#58064=CARTESIAN_POINT('Ctrl Pts',(1.56846244395725,5.62658139707268,72.0290529223617));
#58065=CARTESIAN_POINT('Ctrl Pts',(-3.87635106245531,4.36948453442625,72.1878136846075));
#58066=CARTESIAN_POINT('Ctrl Pts',(-5.77340967182392,-0.88669804176993,
72.3465744468535));
#58067=CARTESIAN_POINT('Ctrl Pts',(-2.38646739844469,-5.33134748559404,
72.5053352090994));
#58068=CARTESIAN_POINT('Ctrl Pts',(3.18464273358708,-4.89658486247307,72.6640959713453));
#58069=CARTESIAN_POINT('Ctrl Pts',(5.84107055966092,0.0196817949154431,
72.8228567335911));
#58070=CARTESIAN_POINT('Ctrl Pts',(3.15157219170978,4.91793507240897,72.9816174958371));
#58071=CARTESIAN_POINT('Ctrl Pts',(-2.42234131212014,5.31514395135115,73.1403782580829));
#58072=CARTESIAN_POINT('Ctrl Pts',(-5.77925405571895,0.847770732830903,
73.2991390203289));
#58073=CARTESIAN_POINT('Ctrl Pts',(-3.84681695791018,-4.39550815587048,
73.4578997825747));
#58074=CARTESIAN_POINT('Ctrl Pts',(1.60634452233207,-5.61588371777435,73.6166605448206));
#58075=CARTESIAN_POINT('Ctrl Pts',(5.58933042930359,-1.6964309617693,73.7754213070665));
#58076=CARTESIAN_POINT('Ctrl Pts',(4.45679039905553,3.77564722860532,73.9341820693123));
#58077=CARTESIAN_POINT('Ctrl Pts',(-0.754740338843374,5.79213774671418,
74.0929428315583));
#58078=CARTESIAN_POINT('Ctrl Pts',(-5.2755096647891,2.50748687587913,74.2517035938041));
#58079=CARTESIAN_POINT('Ctrl Pts',(-4.96797140297887,-3.07209257594453,
74.4104643560501));
#58080=CARTESIAN_POINT('Ctrl Pts',(-0.113593964499922,-5.83999906397405,
74.5692251182959));
#58081=CARTESIAN_POINT('Ctrl Pts',(4.84474814006207,-3.26296002356047,74.7279858805419));
#58082=CARTESIAN_POINT('Ctrl Pts',(5.36902876208054,2.30043969882727,74.8867466427877));
#58083=CARTESIAN_POINT('Ctrl Pts',(0.979410261924092,5.75840674100279,75.0455074050336));
#58084=CARTESIAN_POINT('Ctrl Pts',(-4.30659442642138,3.94610404098849,75.2042681672795));
#58085=CARTESIAN_POINT('Ctrl Pts',(-5.65107234906636,-1.477793612656,75.3630289295254));
#58086=CARTESIAN_POINT('Ctrl Pts',(-1.82351624359326,-5.54916941220397,
75.5217896917713));
#58087=CARTESIAN_POINT('Ctrl Pts',(3.6729776280452,-4.54177586411616,75.6805504540171));
#58088=CARTESIAN_POINT('Ctrl Pts',(5.80785018193428,0.622389685160801,75.8393112162631));
#58089=CARTESIAN_POINT('Ctrl Pts',(2.62720084622344,5.21692518343825,75.9980719785088));
#58090=CARTESIAN_POINT('Ctrl Pts',(-2.95794295284595,5.0367714007783,76.1568327407549));
#58091=CARTESIAN_POINT('Ctrl Pts',(-5.83588700992668,0.246810581940319,
76.3155935030007));
#58092=CARTESIAN_POINT('Ctrl Pts',(-3.37264901603277,-4.76903882041673,
76.4743542652466));
#58093=CARTESIAN_POINT('Ctrl Pts',(2.17734037623983,-5.42011822214095,76.6331150274925));
#58094=CARTESIAN_POINT('Ctrl Pts',(5.73456134845009,-1.110539867295,76.7918757897384));
#58095=CARTESIAN_POINT('Ctrl Pts',(4.04333661010157,4.21543849598137,76.9506365519843));
#58096=CARTESIAN_POINT('Ctrl Pts',(-1.34847329913683,5.68331878549001,77.1093973142302));
#58097=CARTESIAN_POINT('Ctrl Pts',(-5.50611925535187,1.94965212328559,77.2681580764761));
#58098=CARTESIAN_POINT('Ctrl Pts',(-4.62439668246642,-3.56839571504929,
77.4269188387219));
#58099=CARTESIAN_POINT('Ctrl Pts',(0.489714988248199,-5.82053879690483,
77.5856796009679));
#58100=CARTESIAN_POINT('Ctrl Pts',(5.15562454317905,-2.74554698116043,77.7444403632137));
#58101=CARTESIAN_POINT('Ctrl Pts',(5.1029490355901,2.8422532955665,77.9032011254596));
#58102=CARTESIAN_POINT('Ctrl Pts',(0.379898699021361,5.82873653843356,78.0619618877055));
#58103=CARTESIAN_POINT('Ctrl Pts',(-4.69084653104859,3.48058206025056,78.2207226499513));
#58104=CARTESIAN_POINT('Ctrl Pts',(-5.46838573213,-2.05310743523703,78.3794834121973));
#58105=CARTESIAN_POINT('Ctrl Pts',(-1.24109127714898,-5.70773029301263,
78.5382441744431));
#58106=CARTESIAN_POINT('Ctrl Pts',(4.12208782430557,-4.13846404173107,78.6970049366891));
#58107=CARTESIAN_POINT('Ctrl Pts',(5.71260623814347,1.21845091157291,78.8557656989349));
#58108=CARTESIAN_POINT('Ctrl Pts',(2.07477292900298,5.46020237253759,79.0145264611808));
#58109=CARTESIAN_POINT('Ctrl Pts',(-3.46195593952531,4.70460983810283,79.1732872234267));
#58110=CARTESIAN_POINT('Ctrl Pts',(-5.83019698537905,-0.356785324342241,
79.3320479856726));
#58111=CARTESIAN_POINT('Ctrl Pts',(-2.86246366452812,-5.09163965979981,
79.4908087479185));
#58112=CARTESIAN_POINT('Ctrl Pts',(2.72508383719022,-5.16646985244982,79.6495695101644));
#58113=CARTESIAN_POINT('Ctrl Pts',(5.81855137234204,-0.512789024261698,
79.8083302724102));
#58114=CARTESIAN_POINT('Ctrl Pts',(3.58670296156134,4.61021198227599,79.9670910346562));
#58115=CARTESIAN_POINT('Ctrl Pts',(-1.92780555690993,5.51380616187509,80.1258517969019));
#58116=CARTESIAN_POINT('Ctrl Pts',(-5.67792754410753,1.37099652072606,80.2846125591481));
#58117=CARTESIAN_POINT('Ctrl Pts',(-4.23143680838723,-4.02659101382961,
80.4433733213938));
#58118=CARTESIAN_POINT('Ctrl Pts',(1.08779414529793,-5.73891945869655,80.6021340836398));
#58119=CARTESIAN_POINT('Ctrl Pts',(5.41144267008512,-2.19881351740198,80.7608948458856));
#58120=CARTESIAN_POINT('Ctrl Pts',(4.7823735685733,3.3537137186807,80.9196556081314));
#58121=CARTESIAN_POINT('Ctrl Pts',(-0.223669902459649,5.83681971885304,
81.0784163703775));
#58122=CARTESIAN_POINT('Ctrl Pts',(-5.02500384656033,2.97789002445559,81.2371771326232));
#58123=CARTESIAN_POINT('Ctrl Pts',(-5.22730077976831,-2.60649558135874,
81.3959378948693));
#58124=CARTESIAN_POINT('Ctrl Pts',(-0.645412368928784,-5.8053368142863,
81.5546986571149));
#58125=CARTESIAN_POINT('Ctrl Pts',(4.52717715552302,-3.69095646919078,81.713459419361));
#58126=CARTESIAN_POINT('Ctrl Pts',(5.5563558643626,1.80149997964642,81.8722201816067));
#58127=CARTESIAN_POINT('Ctrl Pts',(1.5001879620707,5.64516861688714,82.0309809438528));
#58128=CARTESIAN_POINT('Ctrl Pts',(-3.92899778126385,4.3222065071854,82.1897417060986));
#58129=CARTESIAN_POINT('Ctrl Pts',(-5.76224475326896,-0.956571031279116,
82.3485024683446));
#58130=CARTESIAN_POINT('Ctrl Pts',(-2.32170929618077,-5.35986552417092,
82.5072632305903));
#58131=CARTESIAN_POINT('Ctrl Pts',(3.24372538638481,-4.8576474063222,82.6660239928364));
#58132=CARTESIAN_POINT('Ctrl Pts',(5.8404035909078,0.0904380659057711,82.8247847550821));
#58133=CARTESIAN_POINT('Ctrl Pts',(3.09176588514392,4.95575172494502,82.9835455173283));
#58134=CARTESIAN_POINT('Ctrl Pts',(-2.48655011745873,5.28541028426119,83.1423062795738));
#58135=CARTESIAN_POINT('Ctrl Pts',(-5.78910003705706,0.777699419312094,
83.30106704182));
#58136=CARTESIAN_POINT('Ctrl Pts',(-3.79328774359228,-4.44178477631751,
83.4598278040656));
#58137=CARTESIAN_POINT('Ctrl Pts',(1.67425538991496,-5.59601365552512,83.6185885663117));
#58138=CARTESIAN_POINT('Ctrl Pts',(5.60947262352764,-1.6285964822938,83.7773493285575));
#58139=CARTESIAN_POINT('Ctrl Pts',(4.41072194085603,3.82935538285094,83.9361100908034));
#58140=CARTESIAN_POINT('Ctrl Pts',(-0.8248423466062,5.78257678649102,84.0948708530494));
#58141=CARTESIAN_POINT('Ctrl Pts',(-5.30551223554587,2.44338323992171,84.253631615295));
#58142=CARTESIAN_POINT('Ctrl Pts',(-4.9303644901222,-3.13202323158636,84.4123923775413));
#58143=CARTESIAN_POINT('Ctrl Pts',(-0.0428938145929691,-5.84099457038411,
84.5711531397868));
#58144=CARTESIAN_POINT('Ctrl Pts',(4.88402085037918,-3.20394034224944,84.729913902033));
#58145=CARTESIAN_POINT('Ctrl Pts',(5.3405737125575,2.36513442508082,84.8886746642787));
#58146=CARTESIAN_POINT('Ctrl Pts',(0.90995364228369,5.77018558745976,85.0474354265247));
#58147=CARTESIAN_POINT('Ctrl Pts',(-4.35479260506382,3.89299956501012,85.2061961887705));
#58148=CARTESIAN_POINT('Ctrl Pts',(-5.63139114508318,-1.54490255601334,
85.3649569510165));
#58149=CARTESIAN_POINT('Ctrl Pts',(-1.75878919991609,-5.5732440393258,85.5237177132622));
#58150=CARTESIAN_POINT('Ctrl Pts',(3.73289035077776,-4.49219002151886,85.6824784755083));
#58151=CARTESIAN_POINT('Ctrl Pts',(5.44619302579455,-0.180386406182261,
85.814779110713));
#58152=CARTESIAN_POINT('Ctrl Pts',(4.18934532924144,2.98339184141738,85.9206196188771));
#58153=CARTESIAN_POINT('Ctrl Pts',(2.90742207776985,4.07986902565238,85.973539872959));
#58154=CARTESIAN_POINT('Ctrl Pts',(2.16917135428672,4.4405021828327,86.));
#58155=CARTESIAN_POINT('Ctrl Pts',(2.75898463274055,-3.86904481704483,25.7806068977079));
#58156=CARTESIAN_POINT('Ctrl Pts',(3.40222835107826,-3.41035291299081,25.8070670247489));
#58157=CARTESIAN_POINT('Ctrl Pts',(4.44488144388779,-2.1678284260566,25.8599872788309));
#58158=CARTESIAN_POINT('Ctrl Pts',(5.13713708894935,1.03153993625474,25.9658277869948));
#58159=CARTESIAN_POINT('Ctrl Pts',(2.83087052930385,4.85053885500829,26.0981284221998));
#58160=CARTESIAN_POINT('Ctrl Pts',(-2.54870530784567,5.00827073567408,26.2568891844456));
#58161=CARTESIAN_POINT('Ctrl Pts',(-5.58537388969466,0.575612517731738,
26.4156499466916));
#58162=CARTESIAN_POINT('Ctrl Pts',(-3.51540226351445,-4.38046981539479,
26.5744107089373));
#58163=CARTESIAN_POINT('Ctrl Pts',(1.77471175523205,-5.32917482126994,26.7331714711833));
#58164=CARTESIAN_POINT('Ctrl Pts',(5.43912643226927,-1.39953709723575,26.8919322334291));
#58165=CARTESIAN_POINT('Ctrl Pts',(4.12623242092013,3.81051993270251,27.0506929956751));
#58166=CARTESIAN_POINT('Ctrl Pts',(-0.963505012884285,5.53332322688231,
27.2094537579209));
#58167=CARTESIAN_POINT('Ctrl Pts',(-5.17120987535828,2.19172929477075,27.3682145201668));
#58168=CARTESIAN_POINT('Ctrl Pts',(-4.64617167900849,-3.15573394561846,
27.5269752824127));
#58169=CARTESIAN_POINT('Ctrl Pts',(0.131240194292791,-5.61500874158838,
27.6857360446586));
#58170=CARTESIAN_POINT('Ctrl Pts',(4.78850808778552,-2.93523740776727,27.8444968069045));
#58171=CARTESIAN_POINT('Ctrl Pts',(5.06320222551221,2.43094313930505,28.0032575691504));
#58172=CARTESIAN_POINT('Ctrl Pts',(0.703891137995956,5.57225534640277,28.1620183313963));
#58173=CARTESIAN_POINT('Ctrl Pts',(-4.29963849958627,3.61366660379846,28.3207790936422));
#58174=CARTESIAN_POINT('Ctrl Pts',(-5.36800979937294,-1.65225881189325,
28.4795398558881));
#58175=CARTESIAN_POINT('Ctrl Pts',(-1.52341343958394,-5.40598721644804,
28.638300618134));
#58176=CARTESIAN_POINT('Ctrl Pts',(3.7154568469317,-4.21199061529042,28.7970613803798));
#58177=CARTESIAN_POINT('Ctrl Pts',(5.55382784322941,0.836948256968893,28.9558221426258));
#58178=CARTESIAN_POINT('Ctrl Pts',(2.30916579364752,5.11988662236081,29.1145829048716));
#58179=CARTESIAN_POINT('Ctrl Pts',(-3.04891524119282,4.71694830830577,29.2733436671175));
#58180=CARTESIAN_POINT('Ctrl Pts',(-5.61653596054952,-0.00308515054028371,
29.4321044293634));
#58181=CARTESIAN_POINT('Ctrl Pts',(-3.04373138672984,-4.72029500001125,
29.5908651916093));
#58182=CARTESIAN_POINT('Ctrl Pts',(2.31478911232886,-5.11734667454166,29.7496259538552));
#58183=CARTESIAN_POINT('Ctrl Pts',(5.55474391583396,-0.830846365132238,
29.908386716101));
#58184=CARTESIAN_POINT('Ctrl Pts',(3.71082741246647,4.21606991826224,30.067147478347));
#58185=CARTESIAN_POINT('Ctrl Pts',(-1.52935168579825,5.40431022984286,30.2259082405928));
#58186=CARTESIAN_POINT('Ctrl Pts',(-5.36982140744797,1.64636074283387,30.3846690028388));
#58187=CARTESIAN_POINT('Ctrl Pts',(-4.29566655320965,-3.61838838505691,
30.5434297650846));
#58188=CARTESIAN_POINT('Ctrl Pts',(0.710013543128747,-5.57147793767643,
30.7021905273306));
#58189=CARTESIAN_POINT('Ctrl Pts',(5.06586755727536,-2.42538069880583,30.8609512895764));
#58190=CARTESIAN_POINT('Ctrl Pts',(4.78528484399858,2.94049903987215,31.0197120518223));
#58191=CARTESIAN_POINT('Ctrl Pts',(0.125063273099813,5.61514423852442,31.1784728140682));
#58192=CARTESIAN_POINT('Ctrl Pts',(-4.64962002546522,3.15063791327663,31.3372335763141));
#58193=CARTESIAN_POINT('Ctrl Pts',(-5.16882905222222,-2.19742846769609,
31.49599433856));
#58194=CARTESIAN_POINT('Ctrl Pts',(-0.957367846451143,-5.5343411937037,
31.6547551008058));
#58195=CARTESIAN_POINT('Ctrl Pts',(4.13030565557618,-3.80605581058243,31.8135158630518));
#58196=CARTESIAN_POINT('Ctrl Pts',(5.4377972597899,1.40564810787321,31.9722766252976));
#58197=CARTESIAN_POINT('Ctrl Pts',(1.76845071216457,5.33085994192234,32.1310373875435));
#58198=CARTESIAN_POINT('Ctrl Pts',(-3.51943594526451,4.37710592388724,32.2897981497894));
#58199=CARTESIAN_POINT('Ctrl Pts',(-5.58622732301659,-0.582709136130893,
32.4485589120353));
#58200=CARTESIAN_POINT('Ctrl Pts',(-2.54033282120867,-5.00921099567965,
32.6073196742812));
#58201=CARTESIAN_POINT('Ctrl Pts',(2.83055187404587,-4.8511299436403,32.7660804365271));
#58202=CARTESIAN_POINT('Ctrl Pts',(5.61082903384082,-0.253146587487778,
32.9248411987729));
#58203=CARTESIAN_POINT('Ctrl Pts',(3.25590407686029,4.57652425799672,33.0836019610189));
#58204=CARTESIAN_POINT('Ctrl Pts',(-2.07892374414776,5.217620310809,33.2423627232647));
#58205=CARTESIAN_POINT('Ctrl Pts',(-5.51105705295918,1.08339088088132,33.4011234855107));
#58206=CARTESIAN_POINT('Ctrl Pts',(-3.8993026094728,-4.0423909758343,33.5598842477566));
#58207=CARTESIAN_POINT('Ctrl Pts',(1.28121268795212,-5.46845313502624,33.7186450100024));
#58208=CARTESIAN_POINT('Ctrl Pts',(5.28912299821215,-1.88961994896626,33.8774057722484));
#58209=CARTESIAN_POINT('Ctrl Pts',(4.45626638214284,3.41865113358054,34.0361665344941));
#58210=CARTESIAN_POINT('Ctrl Pts',(-0.455101345292619,5.59806827461589,
34.1949272967401));
#58211=CARTESIAN_POINT('Ctrl Pts',(-4.94994642026466,2.65396233550082,34.353688058986));
#58212=CARTESIAN_POINT('Ctrl Pts',(-4.91444933332838,-2.71913099939964,
34.5124488212319));
#58213=CARTESIAN_POINT('Ctrl Pts',(-0.381098102720512,-5.60359258671175,
34.6712095834778));
#58214=CARTESIAN_POINT('Ctrl Pts',(4.50104575229031,-3.35947507470101,34.8299703457236));
#58215=CARTESIAN_POINT('Ctrl Pts',(5.26369504857235,1.95933664217838,34.9887311079696));
#58216=CARTESIAN_POINT('Ctrl Pts',(1.20884985474224,5.48490361541909,35.1474918702154));
#58217=CARTESIAN_POINT('Ctrl Pts',(-3.95237165094757,3.99051926126589,35.3062526324614));
#58218=CARTESIAN_POINT('Ctrl Pts',(-5.49626189492614,-1.15611021279586,
35.4650133947072));
#58219=CARTESIAN_POINT('Ctrl Pts',(-2.00980536716273,-5.24463230626054,
35.6237741569531));
#58220=CARTESIAN_POINT('Ctrl Pts',(3.31608642293227,-4.53310671365589,35.782534919199));
#58221=CARTESIAN_POINT('Ctrl Pts',(5.60699462758102,0.327256608834102,35.9412956814449));
#58222=CARTESIAN_POINT('Ctrl Pts',(2.76621008118667,4.88810468673588,36.1000564436907));
#58223=CARTESIAN_POINT('Ctrl Pts',(-2.60629442649681,4.97521004623518,36.2588172059367));
#58224=CARTESIAN_POINT('Ctrl Pts',(-5.59343866475058,0.508851201650464,
36.4175779681825));
#58225=CARTESIAN_POINT('Ctrl Pts',(-3.46129698321598,-4.42322380574711,
36.5763387304285));
#58226=CARTESIAN_POINT('Ctrl Pts',(1.83872942405087,-5.30702927699456,36.7350994926743));
#58227=CARTESIAN_POINT('Ctrl Pts',(5.4558944977048,-1.33367944861663,36.8938602549202));
#58228=CARTESIAN_POINT('Ctrl Pts',(4.07965827459196,3.86029454890444,37.0526210171661));
#58229=CARTESIAN_POINT('Ctrl Pts',(-1.03040581621204,5.52120906103586,37.211381779412));
#58230=CARTESIAN_POINT('Ctrl Pts',(-5.1974110298633,2.12894439298054,37.3701425416579));
#58231=CARTESIAN_POINT('Ctrl Pts',(-4.60758691199661,-3.21179521298375,
37.5289033039038));
#58232=CARTESIAN_POINT('Ctrl Pts',(0.199241488304119,-5.61300173446314,
37.6876640661497));
#58233=CARTESIAN_POINT('Ctrl Pts',(4.82371799259843,-2.87701761719148,37.8464248283956));
#58234=CARTESIAN_POINT('Ctrl Pts',(5.03338044768208,2.49210090298119,38.0051855906414));
#58235=CARTESIAN_POINT('Ctrl Pts',(0.636339370439441,5.58037255453223,38.1639463528873));
#58236=CARTESIAN_POINT('Ctrl Pts',(-4.34309893586852,3.56131678947628,38.3227071151332));
#58237=CARTESIAN_POINT('Ctrl Pts',(-5.34760043438529,-1.71716488314614,
38.4814678773791));
#58238=CARTESIAN_POINT('Ctrl Pts',(-1.45781467077047,-5.4240448032289,38.640228639625));
#58239=CARTESIAN_POINT('Ctrl Pts',(3.76620760906239,-4.16667323979076,38.7989894018709));
#58240=CARTESIAN_POINT('Ctrl Pts',(5.54328164477202,0.904164945395139,38.9577501641167));
#58241=CARTESIAN_POINT('Ctrl Pts',(2.2469749974438,5.14748375447756,39.1165109263627));
#58242=CARTESIAN_POINT('Ctrl Pts',(-3.10583180228996,4.67966819952357,39.2752716886085));
#58243=CARTESIAN_POINT('Ctrl Pts',(-5.61608646770029,-0.0711226339607316,
39.4340324508545));
#58244=CARTESIAN_POINT('Ctrl Pts',(-2.98632725227654,-4.75681986037505,
39.5927932131003));
#58245=CARTESIAN_POINT('Ctrl Pts',(2.37660988298438,-5.08893025161958,39.7515539753462));
#58246=CARTESIAN_POINT('Ctrl Pts',(5.56440105884388,-0.763496233183334,
39.9103147375921));
#58247=CARTESIAN_POINT('Ctrl Pts',(3.65948241880601,4.26071285915838,40.069075499838));
#58248=CARTESIAN_POINT('Ctrl Pts',(-1.59470631126904,5.3853873976295,40.2278362620839));
#58249=CARTESIAN_POINT('Ctrl Pts',(-5.38937111433215,1.58119089099016,40.3865970243298));
#58250=CARTESIAN_POINT('Ctrl Pts',(-4.25151885307432,-3.67015981718801,
40.5453577865757));
#58251=CARTESIAN_POINT('Ctrl Pts',(0.777453326851397,-5.56246815418439,
40.7041185488216));
#58252=CARTESIAN_POINT('Ctrl Pts',(5.09487647442165,-2.36383572866916,40.8628793110675));
#58253=CARTESIAN_POINT('Ctrl Pts',(4.74931304757294,2.9982513600266,41.0216400733133));
#58254=CARTESIAN_POINT('Ctrl Pts',(0.0570332499295138,5.61624722124574,
41.1804008355593));
#58255=CARTESIAN_POINT('Ctrl Pts',(-4.6874451201527,3.09408207507567,41.3391615978051));
#58256=CARTESIAN_POINT('Ctrl Pts',(-5.14183053639566,-2.25988149617119,
41.497922360051));
#58257=CARTESIAN_POINT('Ctrl Pts',(-0.89025558647059,-5.5455324931431,41.6566831222969));
#58258=CARTESIAN_POINT('Ctrl Pts',(4.17610846940334,-3.75574276189485,41.8154438845428));
#58259=CARTESIAN_POINT('Ctrl Pts',(5.4203704931852,1.47141746569594,41.9742046467887));
#58260=CARTESIAN_POINT('Ctrl Pts',(1.70374387423147,5.35189148365012,42.1329654090346));
#58261=CARTESIAN_POINT('Ctrl Pts',(-3.57220117995318,4.33415094011377,42.2917261712804));
#58262=CARTESIAN_POINT('Ctrl Pts',(-5.57875859993888,-0.65033693217899,
42.4504869335264));
#58263=CARTESIAN_POINT('Ctrl Pts',(-2.47946574386026,-5.03961657934126,
42.6092476957722));
#58264=CARTESIAN_POINT('Ctrl Pts',(2.88910989726652,-4.81648519599765,42.7680084580182));
#58265=CARTESIAN_POINT('Ctrl Pts',(5.61348391140414,-0.185159439821055,
42.926769220264));
#58266=CARTESIAN_POINT('Ctrl Pts',(3.200225983726,4.61562989144849,43.0855299825099));
#58267=CARTESIAN_POINT('Ctrl Pts',(-2.14197651643363,5.19205375981362,43.2442907447558));
#58268=CARTESIAN_POINT('Ctrl Pts',(-5.52377668122861,1.01655143385025,43.4030515070017));
#58269=CARTESIAN_POINT('Ctrl Pts',(-3.8500477014075,-4.08932981534074,43.5618122692476));
#58270=CARTESIAN_POINT('Ctrl Pts',(1.34736253598006,-5.45253150732624,43.7205730314935));
#58271=CARTESIAN_POINT('Ctrl Pts',(5.31162542471411,-1.82540981406326,43.8793337937394));
#58272=CARTESIAN_POINT('Ctrl Pts',(4.41452647903867,3.47238269889917,44.0380945559852));
#58273=CARTESIAN_POINT('Ctrl Pts',(-0.522881943720034,5.59214450051854,
44.1968553182311));
#58274=CARTESIAN_POINT('Ctrl Pts',(-4.98173283994925,2.59380484098539,44.355616080477));
#58275=CARTESIAN_POINT('Ctrl Pts',(-4.88114967204592,-2.77846423781803,
44.5143768427229));
#58276=CARTESIAN_POINT('Ctrl Pts',(-0.313189227628139,-5.60779797687521,
44.6731376049688));
#58277=CARTESIAN_POINT('Ctrl Pts',(4.54141156440446,-3.30470371507665,44.8318983672147));
#58278=CARTESIAN_POINT('Ctrl Pts',(5.23957377347164,2.02295633024942,44.9906591294605));
#58279=CARTESIAN_POINT('Ctrl Pts',(1.14231802019273,5.49914495012552,45.1494198917065));
#58280=CARTESIAN_POINT('Ctrl Pts',(-4.00042207772478,3.94234813807709,45.3081806539523));
#58281=CARTESIAN_POINT('Ctrl Pts',(-5.48185369562519,-1.22260611053129,
45.4669414161983));
#58282=CARTESIAN_POINT('Ctrl Pts',(-1.94612536588803,-5.26859390179156,
45.6257021784441));
#58283=CARTESIAN_POINT('Ctrl Pts',(3.37075634388315,-4.492603622836,45.7844629406901));
#58284=CARTESIAN_POINT('Ctrl Pts',(5.60261888663935,0.395154720103479,45.9432237029359));
#58285=CARTESIAN_POINT('Ctrl Pts',(2.70679349012103,4.92125539304622,46.1019844651818));
#58286=CARTESIAN_POINT('Ctrl Pts',(-2.66637198863979,4.94327280856975,46.2607452274277));
#58287=CARTESIAN_POINT('Ctrl Pts',(-5.59919237800458,0.441055955456253,
46.4195059896736));
#58288=CARTESIAN_POINT('Ctrl Pts',(-3.40746087346144,-4.46482878032041,
46.5782667519195));
#58289=CARTESIAN_POINT('Ctrl Pts',(1.90288290472123,-5.28436583637694,46.7370275141654));
#58290=CARTESIAN_POINT('Ctrl Pts',(5.47165012418784,-1.26748986592512,46.8957882764113));
#58291=CARTESIAN_POINT('Ctrl Pts',(4.03259601626857,3.90943154580342,47.0545490386571));
#58292=CARTESIAN_POINT('Ctrl Pts',(-1.09721314298891,5.50832179167125,47.2133098009031));
#58293=CARTESIAN_POINT('Ctrl Pts',(-5.22281931897105,2.06582767992164,47.3720705631488));
#58294=CARTESIAN_POINT('Ctrl Pts',(-4.56834172113761,-3.26737502602034,
47.5308313253949));
#58295=CARTESIAN_POINT('Ctrl Pts',(0.267221761695801,-5.61017630487886,
47.6895920876407));
#58296=CARTESIAN_POINT('Ctrl Pts',(4.85821572583019,-2.81837286444571,47.8483528498866));
#58297=CARTESIAN_POINT('Ctrl Pts',(5.00282226155327,2.5528915098482,48.0071136121325));
#58298=CARTESIAN_POINT('Ctrl Pts',(0.568693050307066,5.58767159524255,48.1658743743783));
#58299=CARTESIAN_POINT('Ctrl Pts',(-4.38592141153559,3.50844395901968,48.3246351366243));
#58300=CARTESIAN_POINT('Ctrl Pts',(-5.32640662782695,-1.78181875531413,
48.4833958988701));
#58301=CARTESIAN_POINT('Ctrl Pts',(-1.39200180112221,-5.44130651842186,
48.6421566611161));
#58302=CARTESIAN_POINT('Ctrl Pts',(3.81640559321821,-4.12074434899823,48.8009174233619));
#58303=CARTESIAN_POINT('Ctrl Pts',(5.53192201501862,0.971248918403669,48.9596781856079));
#58304=CARTESIAN_POINT('Ctrl Pts',(2.18445443391585,5.17432550849803,49.1184389478537));
#58305=CARTESIAN_POINT('Ctrl Pts',(-3.16229257013621,4.64170134138436,49.2771997100997));
#58306=CARTESIAN_POINT('Ctrl Pts',(-5.61481282051529,-0.139149675977844,
49.4359604723455));
#58307=CARTESIAN_POINT('Ctrl Pts',(-2.92848487086811,-4.79264665950293,
49.5947212345914));
#58308=CARTESIAN_POINT('Ctrl Pts',(2.43808188433272,-5.05976702695259,49.7534819968373));
#58309=CARTESIAN_POINT('Ctrl Pts',(5.57324162681136,-0.696034058739029,
49.9122427590832));
#58310=CARTESIAN_POINT('Ctrl Pts',(3.60760039555022,4.30473054066965,50.0710035213291));
#58311=CARTESIAN_POINT('Ctrl Pts',(-1.65982691330743,5.36567425955101,50.229764283575));
#58312=CARTESIAN_POINT('Ctrl Pts',(-5.40812993103286,1.515788999437,50.3885250458208));
#58313=CARTESIAN_POINT('Ctrl Pts',(-4.20674724239739,-3.7213926533396,50.5472858080668));
#58314=CARTESIAN_POINT('Ctrl Pts',(0.844779019247828,-5.55264207836113,
50.7060465703126));
#58315=CARTESIAN_POINT('Ctrl Pts',(5.12313771836632,-2.30194386560584,50.8648073325585));
#58316=CARTESIAN_POINT('Ctrl Pts',(4.71264428935673,3.05556368674283,51.0235680948044));
#58317=CARTESIAN_POINT('Ctrl Pts',(-0.0110051428662697,5.61652601957635,
51.1823288570503));
#58318=CARTESIAN_POINT('Ctrl Pts',(-4.7245823321816,3.03707218027256,51.3410896192961));
#58319=CARTESIAN_POINT('Ctrl Pts',(-5.11407745683792,-2.32200288699436,
51.4998503815421));
#58320=CARTESIAN_POINT('Ctrl Pts',(-0.82301268146625,-5.55590998558236,
51.6586111437879));
#58321=CARTESIAN_POINT('Ctrl Pts',(4.22129843923301,-3.70487855788512,51.8173719060339));
#58322=CARTESIAN_POINT('Ctrl Pts',(5.40214828710646,1.53697089297761,51.9761326682797));
#58323=CARTESIAN_POINT('Ctrl Pts',(1.63878701185215,5.37213763520004,52.1348934305256));
#58324=CARTESIAN_POINT('Ctrl Pts',(-3.62444219405034,4.29055991960671,52.2936541927716));
#58325=CARTESIAN_POINT('Ctrl Pts',(-5.57047119392959,-0.717869291269865,
52.4524149550173));
#58326=CARTESIAN_POINT('Ctrl Pts',(-2.41823480486641,-5.06928259917325,
52.6111757172634));
#58327=CARTESIAN_POINT('Ctrl Pts',(2.94724394355444,-4.78113362906013,52.7699364795091));
#58328=CARTESIAN_POINT('Ctrl Pts',(5.6153150100958,-0.117145120002924,52.9286972417552));
#58329=CARTESIAN_POINT('Ctrl Pts',(3.14407825736721,4.65405818112524,53.0874580040009));
#58330=CARTESIAN_POINT('Ctrl Pts',(-2.20471495362471,5.16572527482943,53.2462187662469));
#58331=CARTESIAN_POINT('Ctrl Pts',(-5.53568569516419,0.949562807876645,
53.4049795284926));
#58332=CARTESIAN_POINT('Ctrl Pts',(-3.80022779876814,-4.13566854561846,
53.5637402907387));
#58333=CARTESIAN_POINT('Ctrl Pts',(1.41331465853004,-5.43580972052295,53.7225010529844));
#58334=CARTESIAN_POINT('Ctrl Pts',(5.33334837008319,-1.76093180023503,53.8812618152305));
#58335=CARTESIAN_POINT('Ctrl Pts',(4.37213874408905,3.52560469199021,54.0400225774763));
#58336=CARTESIAN_POINT('Ctrl Pts',(-0.590585809212258,5.58540007910849,
54.1987833397222));
#58337=CARTESIAN_POINT('Ctrl Pts',(-5.01278819024406,2.53326670555979,54.3575441019681));
#58338=CARTESIAN_POINT('Ctrl Pts',(-4.8471337019555,-2.83738973655626,54.516304864214));
#58339=CARTESIAN_POINT('Ctrl Pts',(-0.245234392010581,-5.61118042257805,
54.6750656264598));
#58340=CARTESIAN_POINT('Ctrl Pts',(4.58111092428449,-3.2494473901187,54.8338263887058));
#58341=CARTESIAN_POINT('Ctrl Pts',(5.21468359081919,2.08627914944017,54.9925871509516));
#58342=CARTESIAN_POINT('Ctrl Pts',(1.07561855045193,5.51257928520504,55.1513479131975));
#58343=CARTESIAN_POINT('Ctrl Pts',(-4.04788544248539,3.89359847522351,55.3101086754434));
#58344=CARTESIAN_POINT('Ctrl Pts',(-5.46664103418928,-1.28892259079655,
55.4688694376893));
#58345=CARTESIAN_POINT('Ctrl Pts',(-1.88215977067859,-5.29178233106645,
55.6276301999352));
#58346=CARTESIAN_POINT('Ctrl Pts',(3.42493160627594,-4.45144124234838,55.7863909621811));
#58347=CARTESIAN_POINT('Ctrl Pts',(5.59742096126865,0.46299484241015,55.9451517244269));
#58348=CARTESIAN_POINT('Ctrl Pts',(2.64697967705877,4.95368390503328,56.1039124866729));
#58349=CARTESIAN_POINT('Ctrl Pts',(-2.72605826064226,4.91061014552488,56.2626732489187));
#58350=CARTESIAN_POINT('Ctrl Pts',(-5.60412440966974,0.373195984292183,
56.4214340111647));
#58351=CARTESIAN_POINT('Ctrl Pts',(-3.35312471875849,-4.5057785411845,56.5801947734105));
#58352=CARTESIAN_POINT('Ctrl Pts',(1.96675713728871,-5.26092691497154,56.7389555356564));
#58353=CARTESIAN_POINT('Ctrl Pts',(5.48660278591027,-1.20111427907158,56.8977162979024));
#58354=CARTESIAN_POINT('Ctrl Pts',(3.9849419744025,3.95799483354801,57.0564770601482));
#58355=CARTESIAN_POINT('Ctrl Pts',(-1.1638594537159,5.49462617597814,57.2152378223941));
#58356=CARTESIAN_POINT('Ctrl Pts',(-5.24746115924365,2.00240780661117,57.37399858464));
#58357=CARTESIAN_POINT('Ctrl Pts',(-4.52842612604344,-3.32247535170916,
57.5327593468859));
#58358=CARTESIAN_POINT('Ctrl Pts',(0.335162820288752,-5.60652758181426,
57.6915201091317));
#58359=CARTESIAN_POINT('Ctrl Pts',(4.89200051581106,-2.75931451542811,57.8502808713777));
#58360=CARTESIAN_POINT('Ctrl Pts',(4.97152991116165,2.61330747983713,58.0090416336235));
#58361=CARTESIAN_POINT('Ctrl Pts',(0.500963274458718,5.59415064503912,58.1678023958695));
#58362=CARTESIAN_POINT('Ctrl Pts',(-4.42810025315133,3.45505626434493,58.3265631581152));
#58363=CARTESIAN_POINT('Ctrl Pts',(-5.30443117099388,-1.84621114554552,
58.4853239203613));
#58364=CARTESIAN_POINT('Ctrl Pts',(-1.325984655183,-5.45776972177896,58.644084682607));
#58365=CARTESIAN_POINT('Ctrl Pts',(3.86604351978,-4.07421073889346,58.802845444853));
#58366=CARTESIAN_POINT('Ctrl Pts',(5.51975057560345,1.03819036061473,58.9616062070988));
#58367=CARTESIAN_POINT('Ctrl Pts',(2.12161330165796,5.20040793015086,59.1203669693448));
#58368=CARTESIAN_POINT('Ctrl Pts',(-3.21828927148705,4.60305331348437,59.2791277315906));
#58369=CARTESIAN_POINT('Ctrl Pts',(-5.61271519944128,-0.207156297777243,
59.4378884938366));
#58370=CARTESIAN_POINT('Ctrl Pts',(-2.8702127342488,-4.82777013764157,59.5966492560824));
#58371=CARTESIAN_POINT('Ctrl Pts',(2.49919609711769,-5.02986128137743,59.7554100183283));
#58372=CARTESIAN_POINT('Ctrl Pts',(5.58126432146331,-0.6284697412833,59.9141707805742));
#58373=CARTESIAN_POINT('Ctrl Pts',(3.55518895686721,4.34811650289146,60.0729315428202));
#58374=CARTESIAN_POINT('Ctrl Pts',(-1.72470393571439,5.34517370867209,60.2316923050659));
#58375=CARTESIAN_POINT('Ctrl Pts',(-5.42609510456254,1.45016466581917,60.3904530673119));
#58376=CARTESIAN_POINT('Ctrl Pts',(-4.161358291482,-3.7720793750479,60.5492138295578));
#58377=CARTESIAN_POINT('Ctrl Pts',(0.911980740306919,-5.54200115220642,
60.7079745918037));
#58378=CARTESIAN_POINT('Ctrl Pts',(5.15064714175253,-2.23971419223624,60.8667353540495));
#58379=CARTESIAN_POINT('Ctrl Pts',(4.67528395050075,3.11242760942936,61.0254961162954));
#58380=CARTESIAN_POINT('Ctrl Pts',(-0.0790419206570804,5.61598059260596,
61.1842568785413));
#58381=CARTESIAN_POINT('Ctrl Pts',(-4.76102621166261,2.97961659506878,61.3430176407873));
#58382=CARTESIAN_POINT('Ctrl Pts',(-5.08557388631535,-2.38378352384928,
61.5017784030331));
#58383=CARTESIAN_POINT('Ctrl Pts',(-0.75564899933528,-5.56547214812468,
61.660539165279));
#58384=CARTESIAN_POINT('Ctrl Pts',(4.26586893343571,-3.65347066287608,61.8192999275249));
#58385=CARTESIAN_POINT('Ctrl Pts',(5.38313331566308,1.60229876975119,61.9780606897708));
#58386=CARTESIAN_POINT('Ctrl Pts',(1.5735896574475,5.39159542544895,62.1368214520167));
#58387=CARTESIAN_POINT('Ctrl Pts',(-3.67615132118597,4.24633925934925,62.2955822142625));
#58388=CARTESIAN_POINT('Ctrl Pts',(-5.56136632116585,-0.785296303028447,
62.4543429765086));
#58389=CARTESIAN_POINT('Ctrl Pts',(-2.3566489898686,-5.09820470168657,62.6131037387542));
#58390=CARTESIAN_POINT('Ctrl Pts',(3.00494548173707,-4.7450804306709,62.7718645010003));
#58391=CARTESIAN_POINT('Ctrl Pts',(5.61632206120212,-0.0491136091362308,
62.930625263246));
#58392=CARTESIAN_POINT('Ctrl Pts',(3.08746913746389,4.69180348767462,63.0893860254921));
#58393=CARTESIAN_POINT('Ctrl Pts',(-2.26712984885402,5.13863871956213,63.2481467877378));
#58394=CARTESIAN_POINT('Ctrl Pts',(-5.54678234711784,0.882434833542929,
63.4069075499838));
#58395=CARTESIAN_POINT('Ctrl Pts',(-3.74985021262651,-4.18140036645774,
63.5656683122296));
#58396=CARTESIAN_POINT('Ctrl Pts',(1.47905937712676,-5.41829022853902,63.7244290744757));
#58397=CARTESIAN_POINT('Ctrl Pts',(5.35428864647665,-1.69619536963139,63.8831898367214));
#58398=CARTESIAN_POINT('Ctrl Pts',(4.32910939769494,3.57830930252506,64.0419505989674));
#58399=CARTESIAN_POINT('Ctrl Pts',(-0.658203006225538,5.57783600012977,
64.2007113612132));
#58400=CARTESIAN_POINT('Ctrl Pts',(-5.04310791377582,2.47235681319663,64.3594721234592));
#58401=CARTESIAN_POINT('Ctrl Pts',(-4.81240641490144,-2.89589884829624,
64.518232885705));
#58402=CARTESIAN_POINT('Ctrl Pts',(-0.177243568241342,-5.61373942744627,
64.676993647951));
#58403=CARTESIAN_POINT('Ctrl Pts',(4.62013800604848,-3.19371420869404,64.8357544101967));
#58404=CARTESIAN_POINT('Ctrl Pts',(5.18902815324987,2.14929580712564,64.9945151724427));
#58405=CARTESIAN_POINT('Ctrl Pts',(1.00876123366836,5.52520464916871,65.1532759346885));
#58406=CARTESIAN_POINT('Ctrl Pts',(-4.09475477997962,3.84427742671915,65.3120366969346));
#58407=CARTESIAN_POINT('Ctrl Pts',(-5.45062614307688,-1.35504992164687,
65.4707974591803));
#58408=CARTESIAN_POINT('Ctrl Pts',(-1.81791796848671,-5.31419419118279,
65.6295582214263));
#58409=CARTESIAN_POINT('Ctrl Pts',(3.47860425988976,-4.40962561277309,65.7883189836721));
#58410=CARTESIAN_POINT('Ctrl Pts',(5.59140161426455,0.530767020214592,65.947079745918));
#58411=CARTESIAN_POINT('Ctrl Pts',(2.58677741967834,4.98538546381227,66.1058405081639));
#58412=CARTESIAN_POINT('Ctrl Pts',(-2.78534448354271,4.87722685034708,66.2646012704098));
#58413=CARTESIAN_POINT('Ctrl Pts',(-5.6082340359703,0.305281246610254,66.4233620326558));
#58414=CARTESIAN_POINT('Ctrl Pts',(-3.29829649293878,-4.54606707896127,
66.5821227949015));
#58415=CARTESIAN_POINT('Ctrl Pts',(2.03034274820855,-5.23671595244054,66.7408835571475));
#58416=CARTESIAN_POINT('Ctrl Pts',(5.50075028856868,-1.13456242867458,66.8996443193933));
#58417=CARTESIAN_POINT('Ctrl Pts',(3.93670314222528,4.00597728547496,67.0584050816393));
#58418=CARTESIAN_POINT('Ctrl Pts',(-1.23033496804577,5.48012422378831,67.2171658438851));
#58419=CARTESIAN_POINT('Ctrl Pts',(-5.27133293449043,1.93869407991674,67.375926606131));
#58420=CARTESIAN_POINT('Ctrl Pts',(-4.48784598432852,-3.37708810407645,
67.534687368377));
#58421=CARTESIAN_POINT('Ctrl Pts',(0.403054693731489,-5.60205610071956,
67.6934481306228));
#58422=CARTESIAN_POINT('Ctrl Pts',(4.92506740462245,-2.69985123695237,67.8522088928687));
#58423=CARTESIAN_POINT('Ctrl Pts',(4.93950798866025,2.67333994690335,68.0109696551146));
#58424=CARTESIAN_POINT('Ctrl Pts',(0.433159982240225,5.59980875312125,68.1697304173605));
#58425=CARTESIAN_POINT('Ctrl Pts',(-4.46962927096998,3.40116154009715,68.3284911796064));
#58426=CARTESIAN_POINT('Ctrl Pts',(-5.28167728878481,-1.91033260425587,
68.4872519418522));
#58427=CARTESIAN_POINT('Ctrl Pts',(-1.25977292097022,-5.47343199732475,
68.6460127040982));
#58428=CARTESIAN_POINT('Ctrl Pts',(3.9151141043812,-4.02707923828464,68.804773466344));
#58429=CARTESIAN_POINT('Ctrl Pts',(5.50676911268545,1.10497944837047,68.96353422859));
#58430=CARTESIAN_POINT('Ctrl Pts',(2.05846082260739,5.22572719184021,69.1222949908358));
#58431=CARTESIAN_POINT('Ctrl Pts',(-3.27381368882556,4.56372978742243,69.2810557530818));
#58432=CARTESIAN_POINT('Ctrl Pts',(-5.60979391230414,-0.27513251938597,
69.4398165153275));
#58433=CARTESIAN_POINT('Ctrl Pts',(-2.81151939385567,-4.86218514042,69.5985772775736));
#58434=CARTESIAN_POINT('Ctrl Pts',(2.55994355282749,-4.99921740356275,69.7573380398193));
#58435=CARTESIAN_POINT('Ctrl Pts',(5.58846796546901,-0.560813195881055,
69.9160988020653));
#58436=CARTESIAN_POINT('Ctrl Pts',(3.50225579413674,4.39086437893307,70.074859564311));
#58437=CARTESIAN_POINT('Ctrl Pts',(-1.78932785778569,5.32388875344897,70.2336203265571));
#58438=CARTESIAN_POINT('Ctrl Pts',(-5.4432639985316,1.38432752050883,70.3923810888029));
#58439=CARTESIAN_POINT('Ctrl Pts',(-4.11535866115752,-3.82221254403565,
70.5511418510488));
#58440=CARTESIAN_POINT('Ctrl Pts',(0.979048628174891,-5.53054693727633,
70.7099026132948));
#58441=CARTESIAN_POINT('Ctrl Pts',(5.17740070757192,-2.17715584076599,70.8686633755405));
#58442=CARTESIAN_POINT('Ctrl Pts',(4.63723751363544,3.16883478330451,71.0274241377865));
#58443=CARTESIAN_POINT('Ctrl Pts',(-0.14706709904452,5.61461102037593,71.1861849000324));
#58444=CARTESIAN_POINT('Ctrl Pts',(-4.79677141045583,2.92172375107252,71.3449456622783));
#58445=CARTESIAN_POINT('Ctrl Pts',(-5.05632400772744,-2.44521434042637,
71.5037064245242));
#58446=CARTESIAN_POINT('Ctrl Pts',(-0.688174425699173,-5.57421757752254,
71.6624671867701));
#58447=CARTESIAN_POINT('Ctrl Pts',(4.30981341129062,-3.60152662097726,71.8212279490159));
#58448=CARTESIAN_POINT('Ctrl Pts',(5.36332836930242,1.66739150914959,71.9799887112618));
#58449=CARTESIAN_POINT('Ctrl Pts',(1.50816137873041,5.41026199896583,72.1387494735078));
#58450=CARTESIAN_POINT('Ctrl Pts',(-3.72732097304471,4.20149544872403,72.2975102357535));
#58451=CARTESIAN_POINT('Ctrl Pts',(-5.55144531778782,-0.85260807253943,
72.4562709979996));
#58452=CARTESIAN_POINT('Ctrl Pts',(-2.29471733658639,-5.12637864256223,
72.6150317602453));
#58453=CARTESIAN_POINT('Ctrl Pts',(3.06220604411272,-4.70833089163749,72.7737925224914));
#58454=CARTESIAN_POINT('Ctrl Pts',(5.61650491693822,0.0189251091536447,
72.9325532847371));
#58455=CARTESIAN_POINT('Ctrl Pts',(3.03040693140542,4.72886027197227,73.0913140469831));
#58456=CARTESIAN_POINT('Ctrl Pts',(-2.32921204273454,5.11079806896419,73.2500748092289));
#58457=CARTESIAN_POINT('Ctrl Pts',(-5.55706500865567,0.815177361880478,
73.4088355714748));
#58458=CARTESIAN_POINT('Ctrl Pts',(-3.69892233589434,-4.22651856671307,
73.5675963337208));
#58459=CARTESIAN_POINT('Ctrl Pts',(1.54458704373152,-5.39997560236016,73.7263570959665));
#58460=CARTESIAN_POINT('Ctrl Pts',(5.37444318090863,-1.63121002232468,73.8851178582126));
#58461=CARTESIAN_POINT('Ctrl Pts',(4.28544475441368,3.63048879610115,74.0438786204583));
#58462=CARTESIAN_POINT('Ctrl Pts',(-0.725723611935015,5.56945337361106,
74.2026393827042));
#58463=CARTESIAN_POINT('Ctrl Pts',(-5.07268756112454,2.41108410242379,74.3614001449502));
#58464=CARTESIAN_POINT('Ctrl Pts',(-4.77697290711372,-2.9539829868247,74.5201609071961));
#58465=CARTESIAN_POINT('Ctrl Pts',(-0.109226733975009,-5.61547461594591,
74.6789216694419));
#58466=CARTESIAN_POINT('Ctrl Pts',(4.65848708247156,-3.13751234964793,74.8376824316879));
#58467=CARTESIAN_POINT('Ctrl Pts',(5.16261122569953,2.21199705561036,74.9964431939337));
#58468=CARTESIAN_POINT('Ctrl Pts',(0.94175588115421,5.53701918924425,75.1552039561797));
#58469=CARTESIAN_POINT('Ctrl Pts',(-4.14102321213148,3.79439223042856,75.3139647184255));
#58470=CARTESIAN_POINT('Ctrl Pts',(-5.43381137247341,-1.42097839889528,
75.4727254806715));
#58471=CARTESIAN_POINT('Ctrl Pts',(-1.75340938679805,-5.33582619319972,
75.6314862429172));
#58472=CARTESIAN_POINT('Ctrl Pts',(3.53176642826186,-4.36716287055454,75.7902470051633));
#58473=CARTESIAN_POINT('Ctrl Pts',(5.58456172896637,0.598461307948863,75.949007767409));
#58474=CARTESIAN_POINT('Ctrl Pts',(2.52619555266178,5.0163554171789,76.107768529655));
#58475=CARTESIAN_POINT('Ctrl Pts',(-2.84422195708685,4.8431278220354,76.2665292919008));
#58476=CARTESIAN_POINT('Ctrl Pts',(-5.61152065381861,0.23732170889948,76.4252900541468));
#58477=CARTESIAN_POINT('Ctrl Pts',(-3.24298424204541,-4.58568848130712,
76.5840508163926));
#58478=CARTESIAN_POINT('Ctrl Pts',(2.09363040629115,-5.21173650174305,76.7428115786384));
#58479=CARTESIAN_POINT('Ctrl Pts',(5.51409055601673,-1.06784408121947,76.9015723408844));
#58480=CARTESIAN_POINT('Ctrl Pts',(3.88788659878658,4.05337186015841,77.0603331031303));
#58481=CARTESIAN_POINT('Ctrl Pts',(-1.29662993069554,5.46481806326361,77.2190938653762));
#58482=CARTESIAN_POINT('Ctrl Pts',(-5.29443114152808,1.8746958498288,77.377854627622));
#58483=CARTESIAN_POINT('Ctrl Pts',(-4.44660725112929,-3.43120526869962,
77.5366153898679));
#58484=CARTESIAN_POINT('Ctrl Pts',(0.470887418890042,-5.59676251778467,
77.6953761521139));
#58485=CARTESIAN_POINT('Ctrl Pts',(4.95741153969778,-2.63999175525599,77.8541369143597));
#58486=CARTESIAN_POINT('Ctrl Pts',(4.90676119326682,2.73298010128111,78.0128976766056));
#58487=CARTESIAN_POINT('Ctrl Pts',(0.365293123785983,5.60464508916152,78.1716584388516));
#58488=CARTESIAN_POINT('Ctrl Pts',(-4.51050237060752,3.34676769532807,78.3304192010974));
#58489=CARTESIAN_POINT('Ctrl Pts',(-5.25814832033228,-1.9741737216199,78.4891799633432));
#58490=CARTESIAN_POINT('Ctrl Pts',(-1.19337631505721,-5.48829104661996,
78.6479407255893));
#58491=CARTESIAN_POINT('Ctrl Pts',(3.96361014591247,-3.97935676372049,78.806701487835));
#58492=CARTESIAN_POINT('Ctrl Pts',(5.49297953129461,1.17160638037103,78.9654622500811));
#58493=CARTESIAN_POINT('Ctrl Pts',(1.99500626439154,5.25027957796405,79.1242230123267));
#58494=CARTESIAN_POINT('Ctrl Pts',(-3.32885767394246,4.52373653392658,79.2829837745728));
#58495=CARTESIAN_POINT('Ctrl Pts',(-5.60604938780277,-0.34306836529208,
79.4417445368186));
#58496=CARTESIAN_POINT('Ctrl Pts',(-2.75241346293775,-4.89588661743591,
79.6005052990645));
#58497=CARTESIAN_POINT('Ctrl Pts',(2.62031533677199,-4.96783989049817,79.7592660613105));
#58498=CARTESIAN_POINT('Ctrl Pts',(5.59485150169351,-0.493074351131619,
79.9180268235562));
#58499=CARTESIAN_POINT('Ctrl Pts',(3.44880867530152,4.43296789554331,80.0767875858023));
#58500=CARTESIAN_POINT('Ctrl Pts',(-1.85368919596017,5.30182251744854,80.235548348048));
#58501=CARTESIAN_POINT('Ctrl Pts',(-5.45963409340325,1.31828722510949,80.3943091102941));
#58502=CARTESIAN_POINT('Ctrl Pts',(-4.06875510187306,-3.87178480326137,
80.5530698725397));
#58503=CARTESIAN_POINT('Ctrl Pts',(1.04597284064243,-5.51828111447312,80.7118306347859));
#58504=CARTESIAN_POINT('Ctrl Pts',(5.20339448972971,-2.11427799164205,80.8705913970315));
#58505=CARTESIAN_POINT('Ctrl Pts',(4.59851056209243,3.2247769306293,81.0293521592777));
#58506=CARTESIAN_POINT('Ctrl Pts',(-0.215070695363695,5.6124175038425,81.1881129215234));
#58507=CARTESIAN_POINT('Ctrl Pts',(-4.8318126828924,2.86340214411448,81.3468736837694));
#58508=CARTESIAN_POINT('Ctrl Pts',(-5.02633211360974,-2.50628632185673,
81.5056344460153));
#58509=CARTESIAN_POINT('Ctrl Pts',(-0.62059886223198,-5.58214499018382,
81.664395208261));
#58510=CARTESIAN_POINT('Ctrl Pts',(4.35312542352183,-3.54905405536124,81.823155970507));
#58511=CARTESIAN_POINT('Ctrl Pts',(5.34273635521072,1.73223955954653,81.9819167327528));
#58512=CARTESIAN_POINT('Ctrl Pts',(1.44251177575087,5.42813461502377,82.1406774949988));
#58513=CARTESIAN_POINT('Ctrl Pts',(-3.77794363750813,4.15603507125568,82.2994382572446));
#58514=CARTESIAN_POINT('Ctrl Pts',(-5.54070964539341,-0.919794726960242,
82.4581990194906));
#58515=CARTESIAN_POINT('Ctrl Pts',(-2.23244892259243,-5.15380027738969,
82.6169597817364));
#58516=CARTESIAN_POINT('Ctrl Pts',(3.11901720681907,-4.6708904238858,82.7757205439823));
#58517=CARTESIAN_POINT('Ctrl Pts',(5.61586359044797,0.0869610864393738,
82.9344813062282));
#58518=CARTESIAN_POINT('Ctrl Pts',(2.97289993650437,4.765223026495,83.0932420684742));
#58519=CARTESIAN_POINT('Ctrl Pts',(-2.39095227805809,5.08220754164499,83.2520028307198));
#58520=CARTESIAN_POINT('Ctrl Pts',(-5.56653245165825,0.747800008209614,
83.4107635929661));
#58521=CARTESIAN_POINT('Ctrl Pts',(-3.64745110432035,-4.27101603744643,
83.5695243552116));
#58522=CARTESIAN_POINT('Ctrl Pts',(1.60988701191321,-5.38086946399345,83.7282851174578));
#58523=CARTESIAN_POINT('Ctrl Pts',(5.39381098887153,-1.56598350543525,83.8870458797035));
#58524=CARTESIAN_POINT('Ctrl Pts',(4.24114744292764,3.68213208808317,84.0458066419495));
#58525=CARTESIAN_POINT('Ctrl Pts',(-0.793130479779808,5.56025999380927,
84.2045674041954));
#58526=CARTESIAN_POINT('Ctrl Pts',(-5.10153665384735,2.3494449931422,84.3633281664411));
#58527=CARTESIAN_POINT('Ctrl Pts',(-4.74081182862427,-3.01160955008047,
84.5220889286872));
#58528=CARTESIAN_POINT('Ctrl Pts',(-0.0412447201429887,-5.61643184914312,
84.680849690933));
#58529=CARTESIAN_POINT('Ctrl Pts',(4.6962499152168,-3.08076173742818,84.8396104531789));
#58530=CARTESIAN_POINT('Ctrl Pts',(5.13525015825041,2.27420453014635,84.9983712154247));
#58531=CARTESIAN_POINT('Ctrl Pts',(0.874969588857335,5.54834518648496,85.1571319776707));
#58532=CARTESIAN_POINT('Ctrl Pts',(-4.1873683648852,3.74332940771524,85.3158927399165));
#58533=CARTESIAN_POINT('Ctrl Pts',(-5.41488683153288,-1.48550727360877,
85.4746535021625));
#58534=CARTESIAN_POINT('Ctrl Pts',(-1.69117083731324,-5.35897524785026,
85.6334142644083));
#58535=CARTESIAN_POINT('Ctrl Pts',(3.58937574805651,-4.3194834039373,85.7921750266543));
#58536=CARTESIAN_POINT('Ctrl Pts',(5.23680883419176,-0.173451275228434,
85.9244756618591));
#58537=CARTESIAN_POINT('Ctrl Pts',(4.02828187061023,2.86869243836803,86.0303161700231));
#58538=CARTESIAN_POINT('Ctrl Pts',(2.79564340622479,3.92301449006468,86.083236424105));
#58539=CARTESIAN_POINT('Ctrl Pts',(2.08577545033815,4.26978275451652,86.109696551146));
#58540=CARTESIAN_POINT('Ctrl Pts',(2.64867169498355,-3.71434815979776,25.890303448854));
#58541=CARTESIAN_POINT('Ctrl Pts',(3.26619649360659,-3.27399620981999,25.916763575895));
#58542=CARTESIAN_POINT('Ctrl Pts',(4.26716101578614,-2.08115178444252,25.9696838299769));
#58543=CARTESIAN_POINT('Ctrl Pts',(4.93173808918078,0.990295704796579,26.0755243381408));
#58544=CARTESIAN_POINT('Ctrl Pts',(2.71768336588486,4.65659895971115,26.2078249733458));
#58545=CARTESIAN_POINT('Ctrl Pts',(-2.44680000302844,4.80802422056935,26.3665857355916));
#58546=CARTESIAN_POINT('Ctrl Pts',(-5.36205296397033,0.552597707469077,
26.5253464978375));
#58547=CARTESIAN_POINT('Ctrl Pts',(-3.3748453548303,-4.20532476806197,26.6841072600834));
#58548=CARTESIAN_POINT('Ctrl Pts',(1.70375316232487,-5.11609754516703,26.8428680223293));
#58549=CARTESIAN_POINT('Ctrl Pts',(5.22165294276351,-1.34357917457709,27.0016287845752));
#58550=CARTESIAN_POINT('Ctrl Pts',(3.96125258927572,3.65816328556149,27.1603895468211));
#58551=CARTESIAN_POINT('Ctrl Pts',(-0.924981032991848,5.31208345139673,
27.319150309067));
#58552=CARTESIAN_POINT('Ctrl Pts',(-4.96444853774918,2.10409702077966,27.4779110713129));
#58553=CARTESIAN_POINT('Ctrl Pts',(-4.46040303022669,-3.02955771462767,
27.6366718335588));
#58554=CARTESIAN_POINT('Ctrl Pts',(0.125992795951784,-5.39050292069155,
27.7954325958046));
#58555=CARTESIAN_POINT('Ctrl Pts',(4.59704837888827,-2.8178773262279,27.9541933580506));
#58556=CARTESIAN_POINT('Ctrl Pts',(4.86075937558651,2.33374633870135,28.1129541202964));
#58557=CARTESIAN_POINT('Ctrl Pts',(0.67574734249545,5.34945894155921,28.2717148825423));
#58558=CARTESIAN_POINT('Ctrl Pts',(-4.12772534408922,3.46918077578477,28.4304756447882));
#58559=CARTESIAN_POINT('Ctrl Pts',(-5.15337977793343,-1.58619627522226,
28.5892364070341));
#58560=CARTESIAN_POINT('Ctrl Pts',(-1.46250254869165,-5.18983873767588,
28.74799716928));
#58561=CARTESIAN_POINT('Ctrl Pts',(3.56690112283287,-4.04358189961183,28.9067579315259));
#58562=CARTESIAN_POINT('Ctrl Pts',(5.3317682282855,0.803484416727951,29.0655186937718));
#58563=CARTESIAN_POINT('Ctrl Pts',(2.2168380367468,4.91517735084379,29.2242794560177));
#58564=CARTESIAN_POINT('Ctrl Pts',(-2.92700996008437,4.52834978587781,29.3830402182635));
#58565=CARTESIAN_POINT('Ctrl Pts',(-5.39196907660498,-0.00296179645705061,
29.5418009805095));
#58566=CARTESIAN_POINT('Ctrl Pts',(-2.92203337252994,-4.5315626662565,29.7005617427553));
#58567=CARTESIAN_POINT('Ctrl Pts',(2.22223651734922,-4.91273895817748,29.8593225050013));
#58568=CARTESIAN_POINT('Ctrl Pts',(5.33264767340791,-0.797626497839672,
30.0180832672471));
#58569=CARTESIAN_POINT('Ctrl Pts',(3.56245678780991,4.04749809913968,30.176844029493));
#58570=CARTESIAN_POINT('Ctrl Pts',(-1.46820336502753,5.18822880230289,30.3356047917389));
#58571=CARTESIAN_POINT('Ctrl Pts',(-5.15511895218379,1.58053402963151,30.4943655539848));
#58572=CARTESIAN_POINT('Ctrl Pts',(-4.12391220870013,-3.47371376528387,
30.6531263162307));
#58573=CARTESIAN_POINT('Ctrl Pts',(0.681624954493375,-5.34871261609428,
30.8118870784765));
#58574=CARTESIAN_POINT('Ctrl Pts',(4.86331813894988,-2.32840630217865,30.9706478407225));
#58575=CARTESIAN_POINT('Ctrl Pts',(4.59395401058964,2.82292858162795,31.1294086029683));
#58576=CARTESIAN_POINT('Ctrl Pts',(0.120062847618306,5.39063300003123,31.2881693652142));
#58577=CARTESIAN_POINT('Ctrl Pts',(-4.46371350087791,3.02466543778803,31.4469301274601));
#58578=CARTESIAN_POINT('Ctrl Pts',(-4.96216290745751,-2.10956832273333,
31.605690889706));
#58579=CARTESIAN_POINT('Ctrl Pts',(-0.919089249897086,-5.31306071668268,
31.7644516519519));
#58580=CARTESIAN_POINT('Ctrl Pts',(3.96516296311825,-3.65387765317291,31.9232124141978));
#58581=CARTESIAN_POINT('Ctrl Pts',(5.22037691480677,1.34944584766767,32.0819731764437));
#58582=CARTESIAN_POINT('Ctrl Pts',(1.69774245557567,5.11771528936226,32.2407339386896));
#58583=CARTESIAN_POINT('Ctrl Pts',(-3.37871775721717,4.20209537558378,32.3994947009355));
#58584=CARTESIAN_POINT('Ctrl Pts',(-5.36287227432698,-0.559410580603594,
32.5582554631813));
#58585=CARTESIAN_POINT('Ctrl Pts',(-2.43876227490629,-4.80892688600382,
32.7170162254272));
#58586=CARTESIAN_POINT('Ctrl Pts',(2.71737745147233,-4.65716641474905,32.8757769876731));
#58587=CARTESIAN_POINT('Ctrl Pts',(5.38649033088843,-0.24302498571551,33.034537749919));
#58588=CARTESIAN_POINT('Ctrl Pts',(3.12572272698597,4.39354033353968,33.1932985121649));
#58589=CARTESIAN_POINT('Ctrl Pts',(-1.99580179309791,5.00900333710248,33.3520592744107));
#58590=CARTESIAN_POINT('Ctrl Pts',(-5.29070754957905,1.04007348454996,33.5108200366567));
#58591=CARTESIAN_POINT('Ctrl Pts',(-3.74339614991909,-3.88076339052093,
33.6695807989025));
#58592=CARTESIAN_POINT('Ctrl Pts',(1.22998574967103,-5.24980707112582,33.8283415611485));
#58593=CARTESIAN_POINT('Ctrl Pts',(5.07764712075832,-1.81406696279143,33.9871023233943));
#58594=CARTESIAN_POINT('Ctrl Pts',(4.2780907481768,3.28196264128657,34.1458630856403));
#58595=CARTESIAN_POINT('Ctrl Pts',(-0.436904953119544,5.37423978720491,
34.3046238478861));
#58596=CARTESIAN_POINT('Ctrl Pts',(-4.75203189588531,2.54784852158155,34.463384610132));
#58597=CARTESIAN_POINT('Ctrl Pts',(-4.71795409483259,-2.61041153603965,
34.6221453723779));
#58598=CARTESIAN_POINT('Ctrl Pts',(-0.36586059440485,-5.3795432198188,34.7809061346238));
#58599=CARTESIAN_POINT('Ctrl Pts',(4.32107969737961,-3.22515262853255,34.9396668968697));
#58600=CARTESIAN_POINT('Ctrl Pts',(5.05323586102427,1.88099616195643,35.0984276591155));
#58601=CARTESIAN_POINT('Ctrl Pts',(1.16051621156039,5.265599809247,35.2571884213615));
#58602=CARTESIAN_POINT('Ctrl Pts',(-3.79434332315281,3.83096567127432,35.4159491836074));
#58603=CARTESIAN_POINT('Ctrl Pts',(-5.27650394879067,-1.10988526741874,
35.5747099458532));
#58604=CARTESIAN_POINT('Ctrl Pts',(-1.92944698758358,-5.03493530748322,
35.7334707080991));
#58605=CARTESIAN_POINT('Ctrl Pts',(3.18349879238559,-4.3518587600376,35.892231470345));
#58606=CARTESIAN_POINT('Ctrl Pts',(5.38280923632674,0.314171853851074,36.0509922325909));
#58607=CARTESIAN_POINT('Ctrl Pts',(2.65560824713265,4.69266279059105,36.2097529948368));
#58608=CARTESIAN_POINT('Ctrl Pts',(-2.50208652644733,4.77628540213074,36.3685137570827));
#58609=CARTESIAN_POINT('Ctrl Pts',(-5.36979528379463,0.488505720103176,
36.5272745193286));
#58610=CARTESIAN_POINT('Ctrl Pts',(-3.32290337488047,-4.24636931856435,
36.6860352815745));
#58611=CARTESIAN_POINT('Ctrl Pts',(1.76521120212947,-5.09483744984206,36.8447960438204));
#58612=CARTESIAN_POINT('Ctrl Pts',(5.23775056787229,-1.28035472318811,37.0035568060662));
#58613=CARTESIAN_POINT('Ctrl Pts',(3.91654062472413,3.70594775507185,37.1623175683121));
#58614=CARTESIAN_POINT('Ctrl Pts',(-0.98920693046264,5.30045364824194,37.321078330558));
#58615=CARTESIAN_POINT('Ctrl Pts',(-4.98960208717089,2.04382245807619,37.4798390928039));
#58616=CARTESIAN_POINT('Ctrl Pts',(-4.42336100432008,-3.08337747509074,
37.6385998550498));
#58617=CARTESIAN_POINT('Ctrl Pts',(0.191275183005581,-5.38857616006331,
37.7973606172957));
#58618=CARTESIAN_POINT('Ctrl Pts',(4.63085048026802,-2.761985347144,37.9561213795416));
#58619=CARTESIAN_POINT('Ctrl Pts',(4.83212996681944,2.39245882142244,38.1148821417875));
#58620=CARTESIAN_POINT('Ctrl Pts',(0.610896508406062,5.35725159801683,38.2736429040334));
#58621=CARTESIAN_POINT('Ctrl Pts',(-4.16944809457737,3.41892407272547,38.4324036662793));
#58622=CARTESIAN_POINT('Ctrl Pts',(-5.13378644395327,-1.64850719631984,
38.5911644285251));
#58623=CARTESIAN_POINT('Ctrl Pts',(-1.39952662627435,-5.20717432498527,
38.7499251907711));
#58624=CARTESIAN_POINT('Ctrl Pts',(3.61562270886826,-4.00007645621339,38.9086859530169));
#58625=CARTESIAN_POINT('Ctrl Pts',(5.32164370022099,0.868013569211233,39.0674467152629));
#58626=CARTESIAN_POINT('Ctrl Pts',(2.15713382540813,4.94167106227405,39.2262074775087));
#58627=CARTESIAN_POINT('Ctrl Pts',(-2.98165081692889,4.49256025383564,39.3849682397546));
#58628=CARTESIAN_POINT('Ctrl Pts',(-5.39153755590251,-0.0682789259528612,
39.5437290020005));
#58629=CARTESIAN_POINT('Ctrl Pts',(-2.8669244370552,-4.56662714710238,39.7024897642464));
#58630=CARTESIAN_POINT('Ctrl Pts',(2.28158549793223,-4.88545871378134,39.8612505264922));
#58631=CARTESIAN_POINT('Ctrl Pts',(5.3419186932756,-0.732969237328121,40.0200112887382));
#58632=CARTESIAN_POINT('Ctrl Pts',(3.51316472950203,4.09035607396464,40.1787720509841));
#58633=CARTESIAN_POINT('Ctrl Pts',(-1.53094490572569,5.17006256481187,40.3375328132299));
#58634=CARTESIAN_POINT('Ctrl Pts',(-5.17388699991225,1.517969874726,40.4962935754758));
#58635=CARTESIAN_POINT('Ctrl Pts',(-4.08152967334293,-3.52341521170266,
40.6550543377217));
#58636=CARTESIAN_POINT('Ctrl Pts',(0.746368282217007,-5.34006307226206,
40.8138150999676));
#58637=CARTESIAN_POINT('Ctrl Pts',(4.89116718777592,-2.26932209473684,40.9725758622135));
#58638=CARTESIAN_POINT('Ctrl Pts',(4.55942048043523,2.87837178123751,41.1313366244594));
#58639=CARTESIAN_POINT('Ctrl Pts',(0.054752880088232,5.39169188201243,41.2900973867052));
#58640=CARTESIAN_POINT('Ctrl Pts',(-4.50002622856399,2.97037088099662,41.4488581489512));
#58641=CARTESIAN_POINT('Ctrl Pts',(-4.93624387774355,-2.16952428146721,
41.607618911197));
#58642=CARTESIAN_POINT('Ctrl Pts',(-0.854660350479725,-5.32380455255023,
41.766379673443));
#58643=CARTESIAN_POINT('Ctrl Pts',(4.00913443548347,-3.60557627941182,41.9251404356888));
#58644=CARTESIAN_POINT('Ctrl Pts',(5.20364692548634,1.41258553840574,42.0839011979347));
#58645=CARTESIAN_POINT('Ctrl Pts',(1.63562280181919,5.13790592348729,42.2426619601806));
#58646=CARTESIAN_POINT('Ctrl Pts',(-3.42937327082192,4.16085786801338,42.4014227224264));
#58647=CARTESIAN_POINT('Ctrl Pts',(-5.3557021744363,-0.62433440332485,42.5601834846724));
#58648=CARTESIAN_POINT('Ctrl Pts',(-2.38032885595355,-4.83811675819748,
42.7189442469182));
#58649=CARTESIAN_POINT('Ctrl Pts',(2.77359413958947,-4.62390687376719,42.8777050091642));
#58650=CARTESIAN_POINT('Ctrl Pts',(5.38903905804413,-0.177756179390683,
43.03646577141));
#58651=CARTESIAN_POINT('Ctrl Pts',(3.07227082023542,4.43108239999738,43.195226533656));
#58652=CARTESIAN_POINT('Ctrl Pts',(-2.05633351598682,4.9844590177336,43.3539872959018));
#58653=CARTESIAN_POINT('Ctrl Pts',(-5.30291860685286,0.975906490156919,
43.5127480581477));
#58654=CARTESIAN_POINT('Ctrl Pts',(-3.6961106089692,-3.92582546666328,43.6715088203936));
#58655=CARTESIAN_POINT('Ctrl Pts',(1.29349071741166,-5.23452204049296,43.8302695826395));
#58656=CARTESIAN_POINT('Ctrl Pts',(5.09924982902894,-1.75242415230585,43.9890303448854));
#58657=CARTESIAN_POINT('Ctrl Pts',(4.23801973850483,3.33354584856425,44.1477911071313));
#58658=CARTESIAN_POINT('Ctrl Pts',(-0.501975468697378,5.36855286434462,
44.3065518693772));
#58659=CARTESIAN_POINT('Ctrl Pts',(-4.78254739390742,2.4900963140943,44.4653126316231));
#58660=CARTESIAN_POINT('Ctrl Pts',(-4.68598585940108,-2.66737244379737,
44.624073393869));
#58661=CARTESIAN_POINT('Ctrl Pts',(-0.300666931069113,-5.38358046517354,
44.7828341561148));
#58662=CARTESIAN_POINT('Ctrl Pts',(4.35983155656832,-3.1725712012164,44.9415949183607));
#58663=CARTESIAN_POINT('Ctrl Pts',(5.03007903084552,1.94207213354316,45.1003556806066));
#58664=CARTESIAN_POINT('Ctrl Pts',(1.0966445303283,5.27927173031827,45.2591164428526));
#58665=CARTESIAN_POINT('Ctrl Pts',(-3.84047254178868,3.78472058205141,45.4178772050983));
#58666=CARTESIAN_POINT('Ctrl Pts',(-5.26267183489948,-1.17372244870432,
45.5766379673443));
#58667=CARTESIAN_POINT('Ctrl Pts',(-1.86831311430597,-5.05793884258687,
45.7353987295902));
#58668=CARTESIAN_POINT('Ctrl Pts',(3.23598283686748,-4.3129751109803,45.8941594918361));
#58669=CARTESIAN_POINT('Ctrl Pts',(5.37860845135706,0.379355183735526,46.052920254082));
#58670=CARTESIAN_POINT('Ctrl Pts',(2.59856731943033,4.72448802674167,46.2116810163278));
#58671=CARTESIAN_POINT('Ctrl Pts',(-2.55976199751136,4.745625116308,46.3704417785738));
#58672=CARTESIAN_POINT('Ctrl Pts',(-5.37531894538233,0.423421142422616,
46.5292025408196));
#58673=CARTESIAN_POINT('Ctrl Pts',(-3.27121980318429,-4.28631079457517,
46.6879633030656));
#58674=CARTESIAN_POINT('Ctrl Pts',(1.82679962359794,-5.07308016530974,46.8467240653114));
#58675=CARTESIAN_POINT('Ctrl Pts',(5.25287623454225,-1.21681160950152,47.0054848275573));
#58676=CARTESIAN_POINT('Ctrl Pts',(3.87136006443976,3.75312009931705,47.1642455898032));
#58677=CARTESIAN_POINT('Ctrl Pts',(-1.05334308887091,5.28808165269453,47.3230063520491));
#58678=CARTESIAN_POINT('Ctrl Pts',(-5.01399447246331,1.98322935096872,47.4817671142949));
#58679=CARTESIAN_POINT('Ctrl Pts',(-4.38568496040199,-3.13673503129295,
47.6405278765409));
#58680=CARTESIAN_POINT('Ctrl Pts',(0.256537389910642,-5.38586370009625,
47.7992886387868));
#58681=CARTESIAN_POINT('Ctrl Pts',(4.66396888494043,-2.70568539722266,47.9580494010326));
#58682=CARTESIAN_POINT('Ctrl Pts',(4.80279359368822,2.45081882742566,48.1168101632785));
#58683=CARTESIAN_POINT('Ctrl Pts',(0.545954902252042,5.3642587999782,48.2755709255244));
#58684=CARTESIAN_POINT('Ctrl Pts',(-4.21055839213486,3.36816526537215,48.4343316877703));
#58685=CARTESIAN_POINT('Ctrl Pts',(-5.11344003285917,-1.71057600205014,
48.5930924500163));
#58686=CARTESIAN_POINT('Ctrl Pts',(-1.33634516345125,-5.22374586217178,
48.751853212262));
#58687=CARTESIAN_POINT('Ctrl Pts',(3.66381361874176,-3.9559839478389,48.910613974508));
#58688=CARTESIAN_POINT('Ctrl Pts',(5.31073826441816,0.932415312659234,49.0693747367539));
#58689=CARTESIAN_POINT('Ctrl Pts',(2.09711303188655,4.96743959801509,49.2281354989997));
#58690=CARTESIAN_POINT('Ctrl Pts',(-3.03585410457926,4.45611143084931,49.3868962612457));
#58691=CARTESIAN_POINT('Ctrl Pts',(-5.39031483316305,-0.133586031525688,
49.5456570234915));
#58692=CARTESIAN_POINT('Ctrl Pts',(-2.81139477712564,-4.60102147740992,
49.7044177857375));
#58693=CARTESIAN_POINT('Ctrl Pts',(2.34059965410881,-4.85746152713764,49.8631785479833));
#58694=CARTESIAN_POINT('Ctrl Pts',(5.35040578735549,-0.668204414134744,
50.0219393102293));
#58695=CARTESIAN_POINT('Ctrl Pts',(3.46335711374174,4.13261378925387,50.180700072475));
#58696=CARTESIAN_POINT('Ctrl Pts',(-1.59346177998899,5.15113762038552,50.339460834721));
#58697=CARTESIAN_POINT('Ctrl Pts',(-5.19189577974993,1.45518295779302,50.4982215969668));
#58698=CARTESIAN_POINT('Ctrl Pts',(-4.03854817336226,-3.57259959691384,
50.6569823592128));
#58699=CARTESIAN_POINT('Ctrl Pts',(0.811002080346741,-5.33062987404959,
50.8157431214586));
#58700=CARTESIAN_POINT('Ctrl Pts',(4.91829845774134,-2.2099048642455,50.9745038837045));
#58701=CARTESIAN_POINT('Ctrl Pts',(4.5242178552285,2.93339257973907,51.1332646459504));
#58702=CARTESIAN_POINT('Ctrl Pts',(-0.0105651224232033,5.3919595331034,
51.2920254081963));
#58703=CARTESIAN_POINT('Ctrl Pts',(-4.53567857731733,2.91564042222309,51.4507861704422));
#58704=CARTESIAN_POINT('Ctrl Pts',(-4.90960045414457,-2.22916186247211,
51.6095469326881));
#58705=CARTESIAN_POINT('Ctrl Pts',(-0.790106029640123,-5.33376711999718,
51.7683076949339));
#58706=CARTESIAN_POINT('Ctrl Pts',(4.05251756729386,-3.55674578726275,51.92706845718));
#58707=CARTESIAN_POINT('Ctrl Pts',(5.18615330087962,1.47551793218919,52.0858292194257));
#58708=CARTESIAN_POINT('Ctrl Pts',(1.57326312038517,5.15734256981952,52.2445899816717));
#58709=CARTESIAN_POINT('Ctrl Pts',(-3.47952552383355,4.11900975447104,52.4033507439175));
#58710=CARTESIAN_POINT('Ctrl Pts',(-5.34774612514876,-0.689166604960497,
52.5621115061635));
#58711=CARTESIAN_POINT('Ctrl Pts',(-2.32154612369557,-4.86659663666414,
52.7208722684093));
#58712=CARTESIAN_POINT('Ctrl Pts',(2.82940380271352,-4.58996877436295,52.8796330306552));
#58713=CARTESIAN_POINT('Ctrl Pts',(5.39079694361469,-0.112461287343052,
53.0383937929012));
#58714=CARTESIAN_POINT('Ctrl Pts',(3.01836805768307,4.46797420502795,53.1971545551469));
#58715=CARTESIAN_POINT('Ctrl Pts',(-2.11656347189292,4.95918322890829,53.355915317393));
#58716=CARTESIAN_POINT('Ctrl Pts',(-5.31435146071946,0.911596281467614,
53.5146760796387));
#58717=CARTESIAN_POINT('Ctrl Pts',(-3.64828266371651,-3.97031142784319,
53.6734368418848));
#58718=CARTESIAN_POINT('Ctrl Pts',(1.35680586536473,-5.21846884365023,53.8321976041305));
#58719=CARTESIAN_POINT('Ctrl Pts',(5.1201042222894,-1.69052417354231,53.9909583663765));
#58720=CARTESIAN_POINT('Ctrl Pts',(4.19732679935496,3.38463985792481,54.1497191286223));
#58721=CARTESIAN_POINT('Ctrl Pts',(-0.56697231936563,5.36207810624853,54.3084798908682));
#58722=CARTESIAN_POINT('Ctrl Pts',(-4.81236105300778,2.43197868492519,54.4672406531142));
#58723=CARTESIAN_POINT('Ctrl Pts',(-4.65332995545485,-2.72394191459784,
54.6260014153599));
#58724=CARTESIAN_POINT('Ctrl Pts',(-0.235429144855458,-5.3868276699918,
54.784762177606));
#58725=CARTESIAN_POINT('Ctrl Pts',(4.39794361039255,-3.11952419901562,54.9435229398517));
#58726=CARTESIAN_POINT('Ctrl Pts',(5.00618403647253,2.002863106007,55.1022837020977));
#58727=CARTESIAN_POINT('Ctrl Pts',(1.03261191649043,5.29216891816187,55.2610444643436));
#58728=CARTESIAN_POINT('Ctrl Pts',(-3.88603817100542,3.73792008501059,55.4198052265894));
#58729=CARTESIAN_POINT('Ctrl Pts',(-5.24806742381559,-1.23738738619803,
55.5785659888354));
#58730=CARTESIAN_POINT('Ctrl Pts',(-1.80690506604304,-5.08020012506836,
55.7373267510812));
#58731=CARTESIAN_POINT('Ctrl Pts',(3.287992000806,-4.27345853274282,55.8960875133271));
#58732=CARTESIAN_POINT('Ctrl Pts',(5.37361835549403,0.444482843239534,56.054848275573));
#58733=CARTESIAN_POINT('Ctrl Pts',(2.54114505192401,4.7556199441838,56.2136090378189));
#58734=CARTESIAN_POINT('Ctrl Pts',(-2.61706182345312,4.71426840990844,56.3723698000648));
#58735=CARTESIAN_POINT('Ctrl Pts',(-5.38005377881171,0.358274427681354,
56.5311305623107));
#58736=CARTESIAN_POINT('Ctrl Pts',(-3.21905617991939,-4.32562325439461,
56.6898913245565));
#58737=CARTESIAN_POINT('Ctrl Pts',(1.88811996218651,-5.05057840616592,56.8486520868024));
#58738=CARTESIAN_POINT('Ctrl Pts',(5.26723104152409,-1.15308992868801,57.0074128490484));
#58739=CARTESIAN_POINT('Ctrl Pts',(3.82561138199176,3.79974167311562,57.1661736112942));
#58740=CARTESIAN_POINT('Ctrl Pts',(-1.11732466916059,5.27493363106322,57.3249343735401));
#58741=CARTESIAN_POINT('Ctrl Pts',(-5.03765105397079,1.92234520491603,57.4836951357861));
#58742=CARTESIAN_POINT('Ctrl Pts',(-4.34736531713187,-3.18963227156913,
57.6424558980318));
#58743=CARTESIAN_POINT('Ctrl Pts',(0.321761949948743,-5.38236086452793,
57.8012166602778));
#58744=CARTESIAN_POINT('Ctrl Pts',(4.69640285208957,-2.64898838791747,57.9599774225237));
#58745=CARTESIAN_POINT('Ctrl Pts',(4.77275241050502,2.50881917571891,58.1187381847696));
#58746=CARTESIAN_POINT('Ctrl Pts',(0.480933177205712,5.37047879685782,58.2774989470154));
#58747=CARTESIAN_POINT('Ctrl Pts',(-4.25105079016747,3.31691217970165,58.4362597092614));
#58748=CARTESIAN_POINT('Ctrl Pts',(-5.09234322434225,-1.77239378071924,
58.5950204715072));
#58749=CARTESIAN_POINT('Ctrl Pts',(-1.27296759194985,-5.23955081455291,
58.7537812337532));
#58750=CARTESIAN_POINT('Ctrl Pts',(3.71146686389641,-3.91131089874422,58.912541995999));
#58751=CARTESIAN_POINT('Ctrl Pts',(5.29905347767321,0.996680224142156,59.071302758245));
#58752=CARTESIAN_POINT('Ctrl Pts',(2.03678448698746,4.99247916189982,59.2300635204907));
#58753=CARTESIAN_POINT('Ctrl Pts',(-3.08961188058148,4.41900867342512,59.3888242827367));
#58754=CARTESIAN_POINT('Ctrl Pts',(-5.38830108161851,-0.198873533345728,
59.5475850449826));
#58755=CARTESIAN_POINT('Ctrl Pts',(-2.7554525449587,-4.63474060772737,59.7063458072284));
#58756=CARTESIAN_POINT('Ctrl Pts',(2.39927032724118,-4.82875150792175,59.8651065694744));
#58757=CARTESIAN_POINT('Ctrl Pts',(5.35810770928357,-0.603341531930828,
60.0238673317202));
#58758=CARTESIAN_POINT('Ctrl Pts',(3.4130412502586,4.17426504339022,60.1826280939662));
#58759=CARTESIAN_POINT('Ctrl Pts',(-1.65574481370544,5.13145674641463,60.341388856212));
#58760=CARTESIAN_POINT('Ctrl Pts',(-5.20914264878242,1.39218249273314,60.500149618458));
#58761=CARTESIAN_POINT('Ctrl Pts',(-3.99497401635973,-3.62125970306563,
60.6589103807038));
#58762=CARTESIAN_POINT('Ctrl Pts',(0.875516863905577,-5.32041440580089,
60.8176711429497));
#58763=CARTESIAN_POINT('Ctrl Pts',(4.94470796731371,-2.15016333017309,60.9764319051956));
#58764=CARTESIAN_POINT('Ctrl Pts',(4.48835130096483,2.98798290282324,61.1351926674415));
#58765=CARTESIAN_POINT('Ctrl Pts',(-0.0758815745026817,5.39143591402955,
61.2939534296874));
#58766=CARTESIAN_POINT('Ctrl Pts',(-4.57066531515243,2.86048209316173,61.4527141919332));
#58767=CARTESIAN_POINT('Ctrl Pts',(-4.88223654658481,-2.2884723139309,61.6114749541792));
#58768=CARTESIAN_POINT('Ctrl Pts',(-0.725435760725668,-5.34294695701698,
61.770235716425));
#58769=CARTESIAN_POINT('Ctrl Pts',(4.09530599207347,-3.50739334260129,61.9289964786709));
#58770=CARTESIAN_POINT('Ctrl Pts',(5.16789860817661,1.53823379368774,62.0877572409168));
#58771=CARTESIAN_POINT('Ctrl Pts',(1.51067256255815,5.17602237603069,62.2465180031627));
#58772=CARTESIAN_POINT('Ctrl Pts',(-3.52916715640777,4.07655717616831,62.4052787654086));
#58773=CARTESIAN_POINT('Ctrl Pts',(-5.33900529401489,-0.75389767138361,
62.5640395276545));
#58774=CARTESIAN_POINT('Ctrl Pts',(-2.26242270449944,-4.89436234198102,
62.7228002899004));
#58775=CARTESIAN_POINT('Ctrl Pts',(2.88479825077521,-4.5553570969531,62.8815610521463));
#58776=CARTESIAN_POINT('Ctrl Pts',(5.39176372963048,-0.0471498915993996,
63.0403218143921));
#58777=CARTESIAN_POINT('Ctrl Pts',(2.96402234956039,4.50421033475823,63.1990825766381));
#58778=CARTESIAN_POINT('Ctrl Pts',(-2.17648282206887,4.93317967984907,63.3578433388838));
#58779=CARTESIAN_POINT('Ctrl Pts',(-5.32500443340729,0.847152296006667,
63.5166041011299));
#58780=CARTESIAN_POINT('Ctrl Pts',(-3.59991933291304,-4.01421474574488,
63.6753648633757));
#58781=CARTESIAN_POINT('Ctrl Pts',(1.41992190203103,-5.20164983640472,63.8341256256216));
#58782=CARTESIAN_POINT('Ctrl Pts',(5.14020724015703,-1.62837611032391,63.9928863878675));
#58783=CARTESIAN_POINT('Ctrl Pts',(4.15601790241685,3.43523717132127,64.1516471501133));
#58784=CARTESIAN_POINT('Ctrl Pts',(-0.631885966835028,5.35481646308756,
64.3104079123593));
#58785=CARTESIAN_POINT('Ctrl Pts',(-4.84146849803133,2.3735041628375,64.4691686746051));
#58786=CARTESIAN_POINT('Ctrl Pts',(-4.61999117524849,-2.7801116468701,64.6279294368511));
#58787=CARTESIAN_POINT('Ctrl Pts',(-0.170156809410319,-5.38928435774618,
64.7866901990969));
#58788=CARTESIAN_POINT('Ctrl Pts',(4.43541026590754,-3.06601940657889,64.9454509613428));
#58789=CARTESIAN_POINT('Ctrl Pts',(4.98155438449627,2.06336015827155,65.1042117235887));
#58790=CARTESIAN_POINT('Ctrl Pts',(0.968427766834154,5.30428948011521,65.2629724858346));
#58791=CARTESIAN_POINT('Ctrl Pts',(-3.93103352404596,3.69057104812572,65.4217332480805));
#58792=CARTESIAN_POINT('Ctrl Pts',(-5.23269285873673,-1.30087073706907,
65.5804940103263));
#58793=CARTESIAN_POINT('Ctrl Pts',(-1.74523185442701,-5.10171588808409,
65.7392547725724));
#58794=CARTESIAN_POINT('Ctrl Pts',(3.33951865185531,-4.23331482438371,65.8980155348181));
#58795=CARTESIAN_POINT('Ctrl Pts',(5.36783968103429,0.50954527487755,66.0567762970641));
#58796=CARTESIAN_POINT('Ctrl Pts',(2.48334987133277,4.78605397430791,66.2155370593099));
#58797=CARTESIAN_POINT('Ctrl Pts',(-2.67397759552212,4.68221988452942,66.3742978215559));
#58798=CARTESIAN_POINT('Ctrl Pts',(-5.38399908924589,0.29307513616095,66.5330585838017));
#58799=CARTESIAN_POINT('Ctrl Pts',(-3.16642016009836,-4.36430092891852,
66.6918193460477));
#58800=CARTESIAN_POINT('Ctrl Pts',(1.94916321913439,-5.0273354745442,66.8505801082934));
#58801=CARTESIAN_POINT('Ctrl Pts',(5.2808128822496,-1.08919903190536,67.0093408705395));
#58802=CARTESIAN_POINT('Ctrl Pts',(3.77930129100008,3.84580563475087,67.1681016327852));
#58803=CARTESIAN_POINT('Ctrl Pts',(-1.18114228203367,5.26101151282039,67.3268623950312));
#58804=CARTESIAN_POINT('Ctrl Pts',(-5.06056836008944,1.86117895466771,67.485623157277));
#58805=CARTESIAN_POINT('Ctrl Pts',(-4.30840769791819,-3.24206143324834,
67.644383919523));
#58806=CARTESIAN_POINT('Ctrl Pts',(0.386939291414611,-5.37806816739956,
67.8031446817688));
#58807=CARTESIAN_POINT('Ctrl Pts',(4.72814762203013,-2.59190263951545,67.9619054440148));
#58808=CARTESIAN_POINT('Ctrl Pts',(4.74201082581408,2.56645135475007,68.1206662062606));
#58809=CARTESIAN_POINT('Ctrl Pts',(0.415840875206383,5.37591067587102,68.2794269685066));
#58810=CARTESIAN_POINT('Ctrl Pts',(-4.29091934641509,3.26517233710519,68.4381877307524));
#58811=CARTESIAN_POINT('Ctrl Pts',(-5.07049911435956,-1.83395146056701,
68.5969484929983));
#58812=CARTESIAN_POINT('Ctrl Pts',(-1.20940321242992,-5.25458686275155,
68.7557092552442));
#58813=CARTESIAN_POINT('Ctrl Pts',(3.75857545121767,-3.86606386470014,68.9144700174901));
#58814=CARTESIAN_POINT('Ctrl Pts',(5.28659105472879,1.06079887278309,69.073230779736));
#58815=CARTESIAN_POINT('Ctrl Pts',(1.97615704392586,5.01678607937179,69.2319915419818));
#58816=CARTESIAN_POINT('Ctrl Pts',(-3.14291625598096,4.38125742639343,69.3907523042277));
#58817=CARTESIAN_POINT('Ctrl Pts',(-5.38549659678694,-0.264131850470941,
69.5495130664737));
#58818=CARTESIAN_POINT('Ctrl Pts',(-2.69910595007792,-4.66777958977181,
69.7082738287194));
#58819=CARTESIAN_POINT('Ctrl Pts',(2.45758890740704,-4.79933286932947,69.8670345909655));
#58820=CARTESIAN_POINT('Ctrl Pts',(5.36502332880251,-0.538390109345589,
70.0257953532112));
#58821=CARTESIAN_POINT('Ctrl Pts',(3.36222452290666,4.21530372405138,70.1845561154571));
#58822=CARTESIAN_POINT('Ctrl Pts',(-1.7177848668387,5.11102283106786,70.3433168777031));
#58823=CARTESIAN_POINT('Ctrl Pts',(-5.22562507603134,1.32897772486576,70.5020776399489));
#58824=CARTESIAN_POINT('Ctrl Pts',(-3.95081359684368,-3.66938838928662,
70.6608384021949));
#58825=CARTESIAN_POINT('Ctrl Pts',(0.939903165347853,-5.3094181666361,70.8195991644408));
#58826=CARTESIAN_POINT('Ctrl Pts',(4.97039184089704,-2.09010625959075,70.9783599266866));
#58827=CARTESIAN_POINT('Ctrl Pts',(4.45182608106173,3.0421347393591,71.1371206889325));
#58828=CARTESIAN_POINT('Ctrl Pts',(-0.141186890959645,5.39012110163196,
71.2958814511784));
#58829=CARTESIAN_POINT('Ctrl Pts',(-4.60498130776496,2.80490398829831,71.4546422134243));
#58830=CARTESIAN_POINT('Ctrl Pts',(-4.85415617071822,-2.34744693203373,
71.6134029756702));
#58831=CARTESIAN_POINT('Ctrl Pts',(-0.660659034099426,-5.35134271646838,
71.7721637379161));
#58832=CARTESIAN_POINT('Ctrl Pts',(4.13749343062021,-3.4575261878996,71.9309245001619));
#58833=CARTESIAN_POINT('Ctrl Pts',(5.14888552625377,1.60072391934755,72.0896852624079));
#58834=CARTESIAN_POINT('Ctrl Pts',(1.44786031350356,5.19394260085899,72.2484460246537));
#58835=CARTESIAN_POINT('Ctrl Pts',(-3.57829088363412,4.03350636302179,72.4072067868997));
#58836=CARTESIAN_POINT('Ctrl Pts',(-5.32948096375172,-0.818518103308924,
72.5659675491455));
#58837=CARTESIAN_POINT('Ctrl Pts',(-2.20296727472809,-4.92140979953042,
72.7247283113914));
#58838=CARTESIAN_POINT('Ctrl Pts',(2.93976935463837,-4.52007692080191,72.8834890736374));
#58839=CARTESIAN_POINT('Ctrl Pts',(5.39193927421552,0.0181684233918482,
73.0422498358832));
#58840=CARTESIAN_POINT('Ctrl Pts',(2.90924167110106,4.53978547153557,73.201010598129));
#58841=CARTESIAN_POINT('Ctrl Pts',(-2.23608277334895,4.90645218657722,73.359771360375));
#58842=CARTESIAN_POINT('Ctrl Pts',(-5.33487596159239,0.782583990930051,
73.5185321226207));
#58843=CARTESIAN_POINT('Ctrl Pts',(-3.5510277138785,-4.05752897755565,73.6772928848669));
#58844=CARTESIAN_POINT('Ctrl Pts',(1.48282956513097,-5.18406748694598,73.8360536471125));
#58845=CARTESIAN_POINT('Ctrl Pts',(5.15955593251365,-1.56598908288006,73.9948144093587));
#58846=CARTESIAN_POINT('Ctrl Pts',(4.11409910977184,3.48533036359696,74.1535751716043));
#58847=CARTESIAN_POINT('Ctrl Pts',(-0.696706885026663,5.34676900050795,
74.3123359338504));
#58848=CARTESIAN_POINT('Ctrl Pts',(-4.86986545745996,2.31468132896846,74.4710966960961));
#58849=CARTESIAN_POINT('Ctrl Pts',(-4.58597441124858,-2.83587339770487,
74.6298574583422));
#58850=CARTESIAN_POINT('Ctrl Pts',(-0.104859503450096,-5.39095016791776,
74.7886182205879));
#58851=CARTESIAN_POINT('Ctrl Pts',(4.47222602488106,-3.01206467573539,74.9473789828339));
#58852=CARTESIAN_POINT('Ctrl Pts',(4.95619368931852,2.12355441239345,75.1061397450797));
#58853=CARTESIAN_POINT('Ctrl Pts',(0.904101500384337,5.31563163748572,75.2649005073256));
#58854=CARTESIAN_POINT('Ctrl Pts',(-3.97545199784159,3.64268041986863,75.4236612695716));
#58855=CARTESIAN_POINT('Ctrl Pts',(-5.21655039588045,-1.36416318513457,
75.5824220318174));
#58856=CARTESIAN_POINT('Ctrl Pts',(-1.68330253000285,-5.12248297419546,
75.7411827940633));
#58857=CARTESIAN_POINT('Ctrl Pts',(3.39055522847852,-4.19254987699292,75.8999435563093));
#58858=CARTESIAN_POINT('Ctrl Pts',(5.36127327599845,0.574532930736923,76.058704318555));
#58859=CARTESIAN_POINT('Ctrl Pts',(2.42519025910013,4.81578565091957,76.217465080801));
#58860=CARTESIAN_POINT('Ctrl Pts',(-2.73050096132775,4.64948424329249,76.3762258430469));
#58861=CARTESIAN_POINT('Ctrl Pts',(-5.38715429771053,0.227832835858649,
76.5349866052928));
#58862=CARTESIAN_POINT('Ctrl Pts',(-3.11331946805805,-4.40233814219751,
76.6937473675387));
#58863=CARTESIAN_POINT('Ctrl Pts',(2.00992043634247,-5.00335478134514,76.8525081297845));
#58864=CARTESIAN_POINT('Ctrl Pts',(5.29361976358337,-1.02514829514396,77.0112688920305));
#58865=CARTESIAN_POINT('Ctrl Pts',(3.73243658747159,3.89130522433545,77.1700296542762));
#58866=CARTESIAN_POINT('Ctrl Pts',(-1.24478656225425,5.2463173410372,77.3287904165223));
#58867=CARTESIAN_POINT('Ctrl Pts',(-5.0827430277043,1.79973957637201,77.4875511787681));
#58868=CARTESIAN_POINT('Ctrl Pts',(-4.26881781979216,-3.29401482234996,
77.646311941014));
#58869=CARTESIAN_POINT('Ctrl Pts',(0.452059849531884,-5.3729862386645,77.8050727032599));
#58870=CARTESIAN_POINT('Ctrl Pts',(4.75919853621651,-2.53443652935156,77.9638334655057));
#58871=CARTESIAN_POINT('Ctrl Pts',(4.71057335094352,2.62370690699572,78.1225942277518));
#58872=CARTESIAN_POINT('Ctrl Pts',(0.350687548550617,5.38055363988948,78.2813549899974));
#58873=CARTESIAN_POINT('Ctrl Pts',(-4.33015821016646,3.21295333040559,78.4401157522436));
#58874=CARTESIAN_POINT('Ctrl Pts',(-5.04791090853454,-1.89524000800277,
78.5988765144892));
#58875=CARTESIAN_POINT('Ctrl Pts',(-1.14566135296546,-5.26885180022729,
78.7576372767353));
#58876=CARTESIAN_POINT('Ctrl Pts',(3.80513246751939,-3.82024948570991,78.916398038981));
#58877=CARTESIAN_POINT('Ctrl Pts',(5.27335282444574,1.12476184916915,79.0751588012271));
#58878=CARTESIAN_POINT('Ctrl Pts',(1.91523959978009,5.0403567833905,79.2339195634728));
#58879=CARTESIAN_POINT('Ctrl Pts',(-3.19575940835959,4.34286322975033,79.3926803257188));
#58880=CARTESIAN_POINT('Ctrl Pts',(-5.3819017902265,-0.329351406241924,
79.5514410879647));
#58881=CARTESIAN_POINT('Ctrl Pts',(-2.64236326134738,-4.70013357507201,
79.7102018502106));
#58882=CARTESIAN_POINT('Ctrl Pts',(2.51554683635375,-4.76920992854652,79.8689626124565));
#58883=CARTESIAN_POINT('Ctrl Pts',(5.37115163104497,-0.473359678001532,
80.0277233747023));
#58884=CARTESIAN_POINT('Ctrl Pts',(3.31091438904171,4.25572380881061,80.1864841369483));
#58885=CARTESIAN_POINT('Ctrl Pts',(-1.77957283501041,5.089838873022,80.3452448991941));
#58886=CARTESIAN_POINT('Ctrl Pts',(-5.24134064269895,1.26557792949291,80.50400566144));
#58887=CARTESIAN_POINT('Ctrl Pts',(-3.9060733953589,-3.71697859269313,80.6627664236859));
#58888=CARTESIAN_POINT('Ctrl Pts',(1.00415153598694,-5.29764277024969,80.8215271859318));
#58889=CARTESIAN_POINT('Ctrl Pts',(4.99534630937428,-2.02974246588212,80.9802879481777));
#58890=CARTESIAN_POINT('Ctrl Pts',(4.41464755561157,3.0958401425779,81.1390487104235));
#58891=CARTESIAN_POINT('Ctrl Pts',(-0.206471488267744,5.38801528883197,
81.2978094726694));
#58892=CARTESIAN_POINT('Ctrl Pts',(-4.63862151922447,2.74891426377335,81.4565702349153));
#58893=CARTESIAN_POINT('Ctrl Pts',(-4.82536344745119,-2.40607706235473,
81.6153309971613));
#58894=CARTESIAN_POINT('Ctrl Pts',(-0.595785355535171,-5.35895316608133,
81.7740917594071));
#58895=CARTESIAN_POINT('Ctrl Pts',(4.17907369152063,-3.4071516415317,81.932852521653));
#58896=CARTESIAN_POINT('Ctrl Pts',(5.12911684605883,1.66297913944664,82.0916132838989));
#58897=CARTESIAN_POINT('Ctrl Pts',(1.38483558943104,5.2111006131604,82.2503740461447));
#58898=CARTESIAN_POINT('Ctrl Pts',(-3.62688949375241,3.98986363532597,82.4091348083908));
#58899=CARTESIAN_POINT('Ctrl Pts',(-5.31917453751786,-0.883018422641366,
82.5678955706364));
#58900=CARTESIAN_POINT('Ctrl Pts',(-2.1431885490041,-4.94773503060847,82.7266563328826));
#58901=CARTESIAN_POINT('Ctrl Pts',(2.99430902725335,-4.48413344144938,82.8854170951283));
#58902=CARTESIAN_POINT('Ctrl Pts',(5.39132358998814,0.0834841069729651,
83.0441778573743));
#58903=CARTESIAN_POINT('Ctrl Pts',(2.85403398786483,4.57469432804498,83.20293861962));
#58904=CARTESIAN_POINT('Ctrl Pts',(-2.29535443865746,4.87900479902879,83.3616993818661));
#58905=CARTESIAN_POINT('Ctrl Pts',(-5.34396486625942,0.717900597107141,
83.5204601441119));
#58906=CARTESIAN_POINT('Ctrl Pts',(-3.50161446504842,-4.10024729857536,
83.6792209063577));
#58907=CARTESIAN_POINT('Ctrl Pts',(1.54551863391146,-5.16572527246177,83.8379816686037));
#58908=CARTESIAN_POINT('Ctrl Pts',(5.17814935421542,-1.50337052857669,83.9967424308496));
#58909=CARTESIAN_POINT('Ctrl Pts',(4.07157294499926,3.5349087933154,84.1555031930955));
#58910=CARTESIAN_POINT('Ctrl Pts',(-0.761418612953421,5.33794320112753,
84.3142639553413));
#58911=CARTESIAN_POINT('Ctrl Pts',(-4.89756107214883,2.25550674636269,84.4730247175872));
#58912=CARTESIAN_POINT('Ctrl Pts',(-4.55125916712634,-2.89119586857457,
84.6317854798332));
#58913=CARTESIAN_POINT('Ctrl Pts',(-0.0395956256930076,-5.39186912790212,
84.7905462420789));
#58914=CARTESIAN_POINT('Ctrl Pts',(4.50847898005441,-2.95758313260692,84.949307004325));
#58915=CARTESIAN_POINT('Ctrl Pts',(4.92992660394334,2.18327463521188,85.1080677665708));
#58916=CARTESIAN_POINT('Ctrl Pts',(0.83998553543098,5.32650478551015,85.2668285288166));
#58917=CARTESIAN_POINT('Ctrl Pts',(-4.0199441247066,3.59365925042037,85.4255892910627));
#58918=CARTESIAN_POINT('Ctrl Pts',(-5.19838251798258,-1.4261119912042,85.5843500533084));
#58919=CARTESIAN_POINT('Ctrl Pts',(-1.62355247471041,-5.1447064563747,85.7431108155544));
#58920=CARTESIAN_POINT('Ctrl Pts',(3.44586114533526,-4.14677678635576,85.9018715778002));
#58921=CARTESIAN_POINT('Ctrl Pts',(5.02742464258896,-0.1665161442746,86.0341722130051));
#58922=CARTESIAN_POINT('Ctrl Pts',(3.86721841197903,2.75399303531867,86.1400127211691));
#58923=CARTESIAN_POINT('Ctrl Pts',(2.68386473467973,3.76615995447699,86.192932975251));
#58924=CARTESIAN_POINT('Ctrl Pts',(2.00237954638958,4.09906332620035,86.219393102292));
#58925=CARTESIAN_POINT('Ctrl Pts',(2.53835875722654,-3.55965150255068,26.));
#58926=CARTESIAN_POINT('Ctrl Pts',(3.13016463613492,-3.13763950664917,26.026460127041));
#58927=CARTESIAN_POINT('Ctrl Pts',(4.08944058768451,-1.99447514282845,26.079380381123));
#58928=CARTESIAN_POINT('Ctrl Pts',(4.72633908941221,0.949051473338421,26.1852208892869));
#58929=CARTESIAN_POINT('Ctrl Pts',(2.60449620246589,4.46265906441401,26.3175215244918));
#58930=CARTESIAN_POINT('Ctrl Pts',(-2.34489469821123,4.60777770546463,26.4762822867377));
#58931=CARTESIAN_POINT('Ctrl Pts',(-5.13873203824598,0.529582897206408,
26.6350430489835));
#58932=CARTESIAN_POINT('Ctrl Pts',(-3.23428844614615,-4.03017972072915,
26.7938038112295));
#58933=CARTESIAN_POINT('Ctrl Pts',(1.63279456941769,-4.90302026906412,26.9525645734753));
#58934=CARTESIAN_POINT('Ctrl Pts',(5.00417945325775,-1.28762125191842,27.1113253357213));
#58935=CARTESIAN_POINT('Ctrl Pts',(3.79627275763131,3.50580663842047,27.2700860979671));
#58936=CARTESIAN_POINT('Ctrl Pts',(-0.886457053099411,5.09084367591115,
27.428846860213));
#58937=CARTESIAN_POINT('Ctrl Pts',(-4.75768720014009,2.01646474678857,27.5876076224589));
#58938=CARTESIAN_POINT('Ctrl Pts',(-4.27463438144488,-2.90338148363688,
27.7463683847048));
#58939=CARTESIAN_POINT('Ctrl Pts',(0.12074539761077,-5.16599709979471,27.9051291469506));
#58940=CARTESIAN_POINT('Ctrl Pts',(4.40558866999103,-2.70051724468854,28.0638899091966));
#58941=CARTESIAN_POINT('Ctrl Pts',(4.65831652566081,2.23654953809766,28.2226506714425));
#58942=CARTESIAN_POINT('Ctrl Pts',(0.647603546994949,5.12666253671564,28.3814114336883));
#58943=CARTESIAN_POINT('Ctrl Pts',(-3.95581218859218,3.32469494777108,28.5401721959342));
#58944=CARTESIAN_POINT('Ctrl Pts',(-4.93874975649391,-1.52013373855127,
28.6989329581801));
#58945=CARTESIAN_POINT('Ctrl Pts',(-1.40159165779937,-4.9736902589037,28.857693720426));
#58946=CARTESIAN_POINT('Ctrl Pts',(3.41834539873403,-3.87517318393326,29.0164544826719));
#58947=CARTESIAN_POINT('Ctrl Pts',(5.10970861334159,0.770020576487015,29.1752152449178));
#58948=CARTESIAN_POINT('Ctrl Pts',(2.12451027984608,4.71046807932676,29.3339760071637));
#58949=CARTESIAN_POINT('Ctrl Pts',(-2.80510467897592,4.33975126344986,29.4927367694096));
#58950=CARTESIAN_POINT('Ctrl Pts',(-5.16740219266045,-0.00283844237382118,
29.6514975316555));
#58951=CARTESIAN_POINT('Ctrl Pts',(-2.80033535833003,-4.34283033250174,
29.8102582939013));
#58952=CARTESIAN_POINT('Ctrl Pts',(2.12968392236957,-4.70813124181331,29.9690190561473));
#58953=CARTESIAN_POINT('Ctrl Pts',(5.11055143098187,-0.764406630547101,
30.1277798183931));
#58954=CARTESIAN_POINT('Ctrl Pts',(3.41408616315334,3.87892628001712,30.286540580639));
#58955=CARTESIAN_POINT('Ctrl Pts',(-1.4070550442568,4.97214737476293,30.4453013428849));
#58956=CARTESIAN_POINT('Ctrl Pts',(-4.94041649691963,1.51470731642915,30.6040621051308));
#58957=CARTESIAN_POINT('Ctrl Pts',(-3.95215786419059,-3.32903914551084,
30.7628228673767));
#58958=CARTESIAN_POINT('Ctrl Pts',(0.653236365857992,-5.12594729451212,
30.9215836296226));
#58959=CARTESIAN_POINT('Ctrl Pts',(4.6607687206244,-2.23143190555148,31.0803443918685));
#58960=CARTESIAN_POINT('Ctrl Pts',(4.4026231771807,2.70535812338375,31.2391051541143));
#58961=CARTESIAN_POINT('Ctrl Pts',(0.115062422136807,5.16612176153803,31.3978659163603));
#58962=CARTESIAN_POINT('Ctrl Pts',(-4.27780697629061,2.89869296229943,31.5566266786061));
#58963=CARTESIAN_POINT('Ctrl Pts',(-4.7554967626928,-2.02170817777057,31.715387440852));
#58964=CARTESIAN_POINT('Ctrl Pts',(-0.880810653343035,-5.09178023966167,
31.8741482030979));
#58965=CARTESIAN_POINT('Ctrl Pts',(3.80002027066033,-3.5016994957634,32.0329089653438));
#58966=CARTESIAN_POINT('Ctrl Pts',(5.00295656982363,1.29324358746212,32.1916697275897));
#58967=CARTESIAN_POINT('Ctrl Pts',(1.62703419898677,4.90457063680218,32.3504304898356));
#58968=CARTESIAN_POINT('Ctrl Pts',(-3.23799956916984,4.02708482728032,32.5091912520815));
#58969=CARTESIAN_POINT('Ctrl Pts',(-5.13951722563736,-0.536112025076297,
32.6679520143274));
#58970=CARTESIAN_POINT('Ctrl Pts',(-2.33719172860392,-4.60864277632799,
32.8267127765732));
#58971=CARTESIAN_POINT('Ctrl Pts',(2.60420302889879,-4.4632028858578,32.9854735388192));
#58972=CARTESIAN_POINT('Ctrl Pts',(5.16215162793603,-0.232903383943239,
33.144234301065));
#58973=CARTESIAN_POINT('Ctrl Pts',(2.99554137711165,4.21055640908263,33.302995063311));
#58974=CARTESIAN_POINT('Ctrl Pts',(-1.91267984204806,4.80038636339596,33.4617558255568));
#58975=CARTESIAN_POINT('Ctrl Pts',(-5.07035804619892,0.996756088218607,
33.6205165878027));
#58976=CARTESIAN_POINT('Ctrl Pts',(-3.58748969036538,-3.71913580520757,
33.7792773500486));
#58977=CARTESIAN_POINT('Ctrl Pts',(1.17875881138994,-5.0311610072254,33.9380381122944));
#58978=CARTESIAN_POINT('Ctrl Pts',(4.86617124330449,-1.73851397661661,34.0967988745404));
#58979=CARTESIAN_POINT('Ctrl Pts',(4.09991511421076,3.14527414899259,34.2555596367862));
#58980=CARTESIAN_POINT('Ctrl Pts',(-0.418708560946466,5.15041129979394,
34.4143203990322));
#58981=CARTESIAN_POINT('Ctrl Pts',(-4.55411737150595,2.44173470766227,34.5730811612781));
#58982=CARTESIAN_POINT('Ctrl Pts',(-4.5214588563368,-2.50169207267966,34.7318419235239));
#58983=CARTESIAN_POINT('Ctrl Pts',(-0.350623086089188,-5.15549385292585,
34.8906026857698));
#58984=CARTESIAN_POINT('Ctrl Pts',(4.14111364246891,-3.09083018236409,35.0493634480157));
#58985=CARTESIAN_POINT('Ctrl Pts',(4.84277667347619,1.80265568173448,35.2081242102616));
#58986=CARTESIAN_POINT('Ctrl Pts',(1.11218256837853,5.0462960030749,35.3668849725075));
#58987=CARTESIAN_POINT('Ctrl Pts',(-3.63631499535807,3.67141208128276,35.5256457347534));
#58988=CARTESIAN_POINT('Ctrl Pts',(-5.05674600265519,-1.06366032204162,
35.6844064969993));
#58989=CARTESIAN_POINT('Ctrl Pts',(-1.84908860800444,-4.8252383087059,35.8431672592452));
#58990=CARTESIAN_POINT('Ctrl Pts',(3.05091116183891,-4.17061080641931,36.0019280214911));
#58991=CARTESIAN_POINT('Ctrl Pts',(5.15862384507246,0.301087098868051,36.1606887837369));
#58992=CARTESIAN_POINT('Ctrl Pts',(2.54500641307862,4.49722089444621,36.3194495459828));
#58993=CARTESIAN_POINT('Ctrl Pts',(-2.39787862639785,4.5773607580263,36.4782103082287));
#58994=CARTESIAN_POINT('Ctrl Pts',(-5.14615190283867,0.468160238555881,
36.6369710704746));
#58995=CARTESIAN_POINT('Ctrl Pts',(-3.18450976654496,-4.06951483138158,
36.7957318327205));
#58996=CARTESIAN_POINT('Ctrl Pts',(1.69169298020808,-4.88264562268956,36.9544925949664));
#58997=CARTESIAN_POINT('Ctrl Pts',(5.01960663803976,-1.22702999775959,37.1132533572123));
#58998=CARTESIAN_POINT('Ctrl Pts',(3.75342297485632,3.55160096123927,37.2720141194582));
#58999=CARTESIAN_POINT('Ctrl Pts',(-0.94800804471325,5.07969823544803,37.430774881704));
#59000=CARTESIAN_POINT('Ctrl Pts',(-4.78179314447847,1.95870052317183,37.58953564395));
#59001=CARTESIAN_POINT('Ctrl Pts',(-4.23913509664356,-2.95495973719773,
37.7482964061958));
#59002=CARTESIAN_POINT('Ctrl Pts',(0.183308877707052,-5.16415058566349,
37.9070571684418));
#59003=CARTESIAN_POINT('Ctrl Pts',(4.43798296793759,-2.64695307709652,38.0658179306876));
#59004=CARTESIAN_POINT('Ctrl Pts',(4.63087948595682,2.29281673986369,38.2245786929335));
#59005=CARTESIAN_POINT('Ctrl Pts',(0.585453646372677,5.13413064150142,38.3833394551794));
#59006=CARTESIAN_POINT('Ctrl Pts',(-3.99579725328622,3.27653135597467,38.5421002174253));
#59007=CARTESIAN_POINT('Ctrl Pts',(-4.91997245352125,-1.57984950949354,
38.7008609796712));
#59008=CARTESIAN_POINT('Ctrl Pts',(-1.34123858177823,-4.99030384674165,
38.8596217419171));
#59009=CARTESIAN_POINT('Ctrl Pts',(3.46503780867414,-3.83347967263602,39.0183825041629));
#59010=CARTESIAN_POINT('Ctrl Pts',(5.10000575566994,0.831862193027325,39.1771432664089));
#59011=CARTESIAN_POINT('Ctrl Pts',(2.06729265337245,4.73585837007054,39.3359040286547));
#59012=CARTESIAN_POINT('Ctrl Pts',(-2.85746983156782,4.30545230814772,39.4946647909006));
#59013=CARTESIAN_POINT('Ctrl Pts',(-5.16698864410473,-0.0654352179449955,
39.6534255531465));
#59014=CARTESIAN_POINT('Ctrl Pts',(-2.74752162183386,-4.3764344338297,39.8121863153924));
#59015=CARTESIAN_POINT('Ctrl Pts',(2.18656111288008,-4.68198717594309,39.9709470776383));
#59016=CARTESIAN_POINT('Ctrl Pts',(5.11943632770732,-0.702442241472902,
40.1297078398842));
#59017=CARTESIAN_POINT('Ctrl Pts',(3.36684704019806,3.9199992887709,40.2884686021301));
#59018=CARTESIAN_POINT('Ctrl Pts',(-1.46718350018236,4.95473773199425,40.4472293643759));
#59019=CARTESIAN_POINT('Ctrl Pts',(-4.95840288549236,1.45474885846183,40.6059901266218));
#59020=CARTESIAN_POINT('Ctrl Pts',(-3.91154049361154,-3.37667060621731,
40.7647508888677));
#59021=CARTESIAN_POINT('Ctrl Pts',(0.715283237582617,-5.11765799033974,
40.9235116511136));
#59022=CARTESIAN_POINT('Ctrl Pts',(4.6874579011302,-2.17480846080452,41.0822724133595));
#59023=CARTESIAN_POINT('Ctrl Pts',(4.36952791329752,2.75849220244841,41.2410331756054));
#59024=CARTESIAN_POINT('Ctrl Pts',(0.052472510246957,5.16713654277911,41.3997939378513));
#59025=CARTESIAN_POINT('Ctrl Pts',(-4.3126073369753,2.84665968691757,41.5585547000972));
#59026=CARTESIAN_POINT('Ctrl Pts',(-4.73065721909144,-2.07916706676323,
41.7173154623431));
#59027=CARTESIAN_POINT('Ctrl Pts',(-0.819065114488867,-5.10207661195736,
41.8760762245889));
#59028=CARTESIAN_POINT('Ctrl Pts',(3.8421604015636,-3.45540979692878,42.0348369868349));
#59029=CARTESIAN_POINT('Ctrl Pts',(4.98692335778749,1.35375361111553,42.1935977490807));
#59030=CARTESIAN_POINT('Ctrl Pts',(1.56750172940691,4.92392036332446,42.3523585113267));
#59031=CARTESIAN_POINT('Ctrl Pts',(-3.28654536169065,3.98756479591298,42.5111192735724));
#59032=CARTESIAN_POINT('Ctrl Pts',(-5.13264574893371,-0.59833187447071,
42.6698800358185));
#59033=CARTESIAN_POINT('Ctrl Pts',(-2.28119196804685,-4.63661693705371,
42.8286407980642));
#59034=CARTESIAN_POINT('Ctrl Pts',(2.65807838191241,-4.43132855153674,42.9874015603103));
#59035=CARTESIAN_POINT('Ctrl Pts',(5.1645942046841,-0.170352918960309,43.146162322556));
#59036=CARTESIAN_POINT('Ctrl Pts',(2.94431565674484,4.24653490854626,43.304923084802));
#59037=CARTESIAN_POINT('Ctrl Pts',(-1.97069051554003,4.77686427565358,43.4636838470478));
#59038=CARTESIAN_POINT('Ctrl Pts',(-5.0820605324771,0.935261546463589,43.6224446092938));
#59039=CARTESIAN_POINT('Ctrl Pts',(-3.54217351653091,-3.76232111798581,
43.7812053715396));
#59040=CARTESIAN_POINT('Ctrl Pts',(1.23961889884326,-5.01651257365967,43.9399661337855));
#59041=CARTESIAN_POINT('Ctrl Pts',(4.88687423334376,-1.67943849054845,44.0987268960314));
#59042=CARTESIAN_POINT('Ctrl Pts',(4.06151299797099,3.19470899822934,44.2574876582773));
#59043=CARTESIAN_POINT('Ctrl Pts',(-0.481068993674721,5.1449612281707,44.4162484205232));
#59044=CARTESIAN_POINT('Ctrl Pts',(-4.5833619478656,2.38638778720321,44.5750091827691));
#59045=CARTESIAN_POINT('Ctrl Pts',(-4.49082204675623,-2.55628064977671,
44.733769945015));
#59046=CARTESIAN_POINT('Ctrl Pts',(-0.288144634510089,-5.15936295347187,
44.8925307072609));
#59047=CARTESIAN_POINT('Ctrl Pts',(4.17825154873217,-3.04043868735616,45.0512914695067));
#59048=CARTESIAN_POINT('Ctrl Pts',(4.8205842882194,1.86118793683688,45.2100522317526));
#59049=CARTESIAN_POINT('Ctrl Pts',(1.05097104046387,5.05939851051103,45.3688129939986));
#59050=CARTESIAN_POINT('Ctrl Pts',(-3.68052300585259,3.62709302602572,45.5275737562444));
#59051=CARTESIAN_POINT('Ctrl Pts',(-5.04348997417376,-1.12483878687734,
45.6863345184903));
#59052=CARTESIAN_POINT('Ctrl Pts',(-1.79050086272392,-4.84728378338218,
45.8450952807362));
#59053=CARTESIAN_POINT('Ctrl Pts',(3.1012093298518,-4.13334659912459,46.0038560429821));
#59054=CARTESIAN_POINT('Ctrl Pts',(5.15459801607478,0.363555647367575,46.162616805228));
#59055=CARTESIAN_POINT('Ctrl Pts',(2.49034114873962,4.52772066043712,46.3213775674739));
#59056=CARTESIAN_POINT('Ctrl Pts',(-2.45315200638293,4.54797742404625,46.4801383297198));
#59057=CARTESIAN_POINT('Ctrl Pts',(-5.15144551276008,0.405786329388982,
46.6388990919657));
#59058=CARTESIAN_POINT('Ctrl Pts',(-3.13497873290715,-4.10779280882992,
46.7976598542116));
#59059=CARTESIAN_POINT('Ctrl Pts',(1.75071634247466,-4.86179449424254,46.9564206164574));
#59060=CARTESIAN_POINT('Ctrl Pts',(5.03410234489664,-1.16613335307792,47.1151813787034));
#59061=CARTESIAN_POINT('Ctrl Pts',(3.71012411261097,3.59680865283067,47.2739421409492));
#59062=CARTESIAN_POINT('Ctrl Pts',(-1.00947303475291,5.06784151371782,47.4327029031951));
#59063=CARTESIAN_POINT('Ctrl Pts',(-4.80516962595556,1.90063102201579,47.5914636654409));
#59064=CARTESIAN_POINT('Ctrl Pts',(-4.20302819966638,-3.00609503656556,
47.750224427687));
#59065=CARTESIAN_POINT('Ctrl Pts',(0.245853018125491,-5.16155109531365,
47.9089851899327));
#59066=CARTESIAN_POINT('Ctrl Pts',(4.46972204405066,-2.59299792999961,48.0677459521787));
#59067=CARTESIAN_POINT('Ctrl Pts',(4.60276492582317,2.34874614500311,48.2265067144246));
#59068=CARTESIAN_POINT('Ctrl Pts',(0.523216754197009,5.14084600471386,48.3852674766704));
#59069=CARTESIAN_POINT('Ctrl Pts',(-4.03519537273411,3.22788657172462,48.5440282389163));
#59070=CARTESIAN_POINT('Ctrl Pts',(-4.9004734378914,-1.63933324878614,48.7027890011622));
#59071=CARTESIAN_POINT('Ctrl Pts',(-1.2806885257803,-5.00618520592171,48.8615497634081));
#59072=CARTESIAN_POINT('Ctrl Pts',(3.51122164426531,-3.79122354667958,49.020310525654));
#59073=CARTESIAN_POINT('Ctrl Pts',(5.0895545138177,0.893581706914796,49.1790712878999));
#59074=CARTESIAN_POINT('Ctrl Pts',(2.00977162985725,4.76055368753214,49.3378320501457));
#59075=CARTESIAN_POINT('Ctrl Pts',(-2.90941563902232,4.27052152031426,49.4965928123917));
#59076=CARTESIAN_POINT('Ctrl Pts',(-5.1658168458108,-0.128022387073527,
49.6553535746375));
#59077=CARTESIAN_POINT('Ctrl Pts',(-2.69430468338317,-4.40939629531691,
49.8141143368835));
#59078=CARTESIAN_POINT('Ctrl Pts',(2.2431174238849,-4.6551560273227,49.9728750991294));
#59079=CARTESIAN_POINT('Ctrl Pts',(5.12756994789964,-0.640374769530455,
50.1316358613752));
#59080=CARTESIAN_POINT('Ctrl Pts',(3.31911383193326,3.96049703783808,50.2903966236212));
#59081=CARTESIAN_POINT('Ctrl Pts',(-1.52709664667054,4.93660098122003,50.4491573858669));
#59082=CARTESIAN_POINT('Ctrl Pts',(-4.975661628467,1.39457691614903,50.607918148113));
#59083=CARTESIAN_POINT('Ctrl Pts',(-3.87034910432713,-3.42380654048809,
50.7666789103588));
#59084=CARTESIAN_POINT('Ctrl Pts',(0.777225141445664,-5.10861766973804,
50.9254396726047));
#59085=CARTESIAN_POINT('Ctrl Pts',(4.71345919711634,-2.11786586288516,51.0842004348506));
#59086=CARTESIAN_POINT('Ctrl Pts',(4.33579142110028,2.81122147273531,51.2429611970965));
#59087=CARTESIAN_POINT('Ctrl Pts',(-0.0101251019801382,5.16739304663044,
51.4017219593423));
#59088=CARTESIAN_POINT('Ctrl Pts',(-4.34677482245307,2.79420866417363,51.5604827215882));
#59089=CARTESIAN_POINT('Ctrl Pts',(-4.7051234514512,-2.13632083794987,51.7192434838341));
#59090=CARTESIAN_POINT('Ctrl Pts',(-0.757199377814005,-5.111624254412,51.87800424608));
#59091=CARTESIAN_POINT('Ctrl Pts',(3.88373669535471,-3.40861301664037,52.0367650083259));
#59092=CARTESIAN_POINT('Ctrl Pts',(4.97015831465276,1.41406497140078,52.1955257705718));
#59093=CARTESIAN_POINT('Ctrl Pts',(1.50773922891819,4.94254750443899,52.3542865328176));
#59094=CARTESIAN_POINT('Ctrl Pts',(-3.33460885361675,3.94745958933536,52.5130472950636));
#59095=CARTESIAN_POINT('Ctrl Pts',(-5.12502105636793,-0.660463918651125,
52.6718080573094));
#59096=CARTESIAN_POINT('Ctrl Pts',(-2.22485744252472,-4.66391067415503,
52.8305688195554));
#59097=CARTESIAN_POINT('Ctrl Pts',(2.71156366187259,-4.39880391966578,52.9893295818012));
#59098=CARTESIAN_POINT('Ctrl Pts',(5.16627887713359,-0.107777454683187,
53.1480903440472));
#59099=CARTESIAN_POINT('Ctrl Pts',(2.89265785799892,4.28189022893068,53.306851106293));
#59100=CARTESIAN_POINT('Ctrl Pts',(-2.02841199016113,4.75264118298715,53.4656118685389));
#59101=CARTESIAN_POINT('Ctrl Pts',(-5.09301722627474,0.873629755058583,
53.6243726307848));
#59102=CARTESIAN_POINT('Ctrl Pts',(-3.49633752866489,-3.80495431006791,
53.7831333930307));
#59103=CARTESIAN_POINT('Ctrl Pts',(1.30029707219943,-5.00112796677752,53.9418941552766));
#59104=CARTESIAN_POINT('Ctrl Pts',(4.90686007449561,-1.62011654684958,54.1006549175225));
#59105=CARTESIAN_POINT('Ctrl Pts',(4.02251485462088,3.2436750238594,54.2594156797684));
#59106=CARTESIAN_POINT('Ctrl Pts',(-0.543358829519001,5.13875613338857,
54.4181764420142));
#59107=CARTESIAN_POINT('Ctrl Pts',(-4.61193391577151,2.33069066429059,54.5769372042602));
#59108=CARTESIAN_POINT('Ctrl Pts',(-4.4595262089542,-2.61049409263942,54.735697966506));
#59109=CARTESIAN_POINT('Ctrl Pts',(-0.22562389770033,-5.16247491740555,
54.8944587287519));
#59110=CARTESIAN_POINT('Ctrl Pts',(4.21477629650059,-2.98960100791253,55.0532194909978));
#59111=CARTESIAN_POINT('Ctrl Pts',(4.79768448212587,1.91944706257383,55.2119802532437));
#59112=CARTESIAN_POINT('Ctrl Pts',(0.989605282528937,5.07175855111871,55.3707410154895));
#59113=CARTESIAN_POINT('Ctrl Pts',(-3.72419089952545,3.58224169479765,55.5295017777355));
#59114=CARTESIAN_POINT('Ctrl Pts',(-5.0294938134419,-1.1858521815995,55.6882625399813));
#59115=CARTESIAN_POINT('Ctrl Pts',(-1.7316503614075,-4.86861791907028,55.8470233022273));
#59116=CARTESIAN_POINT('Ctrl Pts',(3.15105239533607,-4.09547582313724,56.0057840644731));
#59117=CARTESIAN_POINT('Ctrl Pts',(5.14981574971942,0.425970844068908,56.1645448267191));
#59118=CARTESIAN_POINT('Ctrl Pts',(2.43531042678924,4.55755598333432,56.3233055889649));
#59119=CARTESIAN_POINT('Ctrl Pts',(-2.50806538626398,4.517926674292,56.4820663512109));
#59120=CARTESIAN_POINT('Ctrl Pts',(-5.1559831479537,0.343352871070528,56.6408271134567));
#59121=CARTESIAN_POINT('Ctrl Pts',(-3.08498764108028,-4.14546796760472,
56.7995878757026));
#59122=CARTESIAN_POINT('Ctrl Pts',(1.8094827870843,-4.8402298973603,56.9583486379485));
#59123=CARTESIAN_POINT('Ctrl Pts',(5.04785929713791,-1.10506557830443,57.1171094001944));
#59124=CARTESIAN_POINT('Ctrl Pts',(3.66628078958101,3.64148851268323,57.2758701624403));
#59125=CARTESIAN_POINT('Ctrl Pts',(-1.07078988460527,5.05524108614831,57.4346309246862));
#59126=CARTESIAN_POINT('Ctrl Pts',(-4.82784094869794,1.84228260322088,57.593391686932));
#59127=CARTESIAN_POINT('Ctrl Pts',(-4.16630450822031,-3.05678919142909,
57.7521524491779));
#59128=CARTESIAN_POINT('Ctrl Pts',(0.308361079608735,-5.1581941472416,57.9109132114238));
#59129=CARTESIAN_POINT('Ctrl Pts',(4.50080518836808,-2.53866226040682,58.0696739736697));
#59130=CARTESIAN_POINT('Ctrl Pts',(4.57397490984839,2.40433087160068,58.2284347359156));
#59131=CARTESIAN_POINT('Ctrl Pts',(0.460903079952699,5.14680694867653,58.3871954981615));
#59132=CARTESIAN_POINT('Ctrl Pts',(-4.07400132718361,3.17876809505837,58.5459562604074));
#59133=CARTESIAN_POINT('Ctrl Pts',(-4.88025527769062,-1.69857641589297,
58.7047170226532));
#59134=CARTESIAN_POINT('Ctrl Pts',(-1.21995052871669,-5.02133190732686,
58.8634777848992));
#59135=CARTESIAN_POINT('Ctrl Pts',(3.55689020801282,-3.74841105859499,59.022238547145));
#59136=CARTESIAN_POINT('Ctrl Pts',(5.07835637974298,0.955170087669591,59.1809993093909));
#59137=CARTESIAN_POINT('Ctrl Pts',(1.95195567231696,4.78455039364876,59.3397600716368));
#59138=CARTESIAN_POINT('Ctrl Pts',(-2.96093448967591,4.23496403336588,59.4985208338827));
#59139=CARTESIAN_POINT('Ctrl Pts',(-5.16388696379574,-0.190590768914221,
59.6572815961286));
#59140=CARTESIAN_POINT('Ctrl Pts',(-2.6406923556686,-4.44171107781315,59.8160423583745));
#59141=CARTESIAN_POINT('Ctrl Pts',(2.29934455736468,-4.62764173446609,59.9748031206204));
#59142=CARTESIAN_POINT('Ctrl Pts',(5.13495109710383,-0.578213322578349,
60.1335638828663));
#59143=CARTESIAN_POINT('Ctrl Pts',(3.27089354364999,4.00041358388897,60.2923246451122));
#59144=CARTESIAN_POINT('Ctrl Pts',(-1.58678569169648,4.91773978415717,60.451085407358));
#59145=CARTESIAN_POINT('Ctrl Pts',(-4.99219019300232,1.33420031964711,60.6098461696039));
#59146=CARTESIAN_POINT('Ctrl Pts',(-3.82858974123746,-3.47044003108337,
60.7686069318499));
#59147=CARTESIAN_POINT('Ctrl Pts',(0.839052987504236,-5.09882765939536,
60.9273676940957));
#59148=CARTESIAN_POINT('Ctrl Pts',(4.73876879287487,-2.06061246810993,61.0861284563416));
#59149=CARTESIAN_POINT('Ctrl Pts',(4.30141865142892,2.86353819621711,61.2448892185875));
#59150=CARTESIAN_POINT('Ctrl Pts',(-0.0727212283482856,5.16689123545314,
61.4036499808334));
#59151=CARTESIAN_POINT('Ctrl Pts',(-4.38030441864225,2.74134759125467,61.5624107430792));
#59152=CARTESIAN_POINT('Ctrl Pts',(-4.67889920685427,-2.19316110401252,
61.7211715053253));
#59153=CARTESIAN_POINT('Ctrl Pts',(-0.695222522116061,-5.12042176590928,
61.879932267571));
#59154=CARTESIAN_POINT('Ctrl Pts',(3.92474305071123,-3.3613160223265,62.038693029817));
#59155=CARTESIAN_POINT('Ctrl Pts',(4.95266390069012,1.47416881762428,62.1974537920629));
#59156=CARTESIAN_POINT('Ctrl Pts',(1.4477554676688,4.96044932661243,62.3562145543087));
#59157=CARTESIAN_POINT('Ctrl Pts',(-3.38218299162958,3.90677509298738,62.5149753165547));
#59158=CARTESIAN_POINT('Ctrl Pts',(-5.11664426686392,-0.722499039738782,
62.6737360788005));
#59159=CARTESIAN_POINT('Ctrl Pts',(-2.16819641913028,-4.69051998227545,
62.8324968410464));
#59160=CARTESIAN_POINT('Ctrl Pts',(2.76465101981334,-4.3656337632353,62.9912576032923));
#59161=CARTESIAN_POINT('Ctrl Pts',(5.16720539805885,-0.0451861740625634,
63.1500183655382));
#59162=CARTESIAN_POINT('Ctrl Pts',(2.8405755616569,4.31661718184185,63.308779127784));
#59163=CARTESIAN_POINT('Ctrl Pts',(-2.08583579528372,4.72772064013601,63.46753989003));
#59164=CARTESIAN_POINT('Ctrl Pts',(-5.10322651969674,0.811869758470405,
63.6263006522758));
#59165=CARTESIAN_POINT('Ctrl Pts',(-3.44998845319957,-3.847029125032,63.7850614145218));
#59166=CARTESIAN_POINT('Ctrl Pts',(1.36078442693529,-4.98500944427043,63.9438221767676));
#59167=CARTESIAN_POINT('Ctrl Pts',(4.92612583383742,-1.56055685101642,64.1025829390136));
#59168=CARTESIAN_POINT('Ctrl Pts',(3.98292640713875,3.29216504011747,64.2613437012594));
#59169=CARTESIAN_POINT('Ctrl Pts',(-0.605568927444514,5.13179692604536,
64.4201044635054));
#59170=CARTESIAN_POINT('Ctrl Pts',(-4.63982908228685,2.27465151247837,64.5788652257511));
#59171=CARTESIAN_POINT('Ctrl Pts',(-4.42757593559553,-2.66432444544396,
64.7376259879972));
#59172=CARTESIAN_POINT('Ctrl Pts',(-0.163070050579303,-5.16482928804609,
64.8963867502428));
#59173=CARTESIAN_POINT('Ctrl Pts',(4.25068252576661,-2.93832460446375,65.0551475124889));
#59174=CARTESIAN_POINT('Ctrl Pts',(4.77408061574266,1.97742450941745,65.2139082747347));
#59175=CARTESIAN_POINT('Ctrl Pts',(0.928094299999949,5.08337431106172,65.3726690369806));
#59176=CARTESIAN_POINT('Ctrl Pts',(-3.76731226811231,3.53686466953228,65.5314297992265));
#59177=CARTESIAN_POINT('Ctrl Pts',(-5.01475957439658,-1.24669155249126,
65.6901905614724));
#59178=CARTESIAN_POINT('Ctrl Pts',(-1.67254574036732,-4.88923758498539,
65.8489513237183));
#59179=CARTESIAN_POINT('Ctrl Pts',(3.20043304382085,-4.05700403599433,66.0077120859643));
#59180=CARTESIAN_POINT('Ctrl Pts',(5.14427774780404,0.488323529540513,66.16647284821));
#59181=CARTESIAN_POINT('Ctrl Pts',(2.3799223229872,4.58672248480354,66.3252336104561));
#59182=CARTESIAN_POINT('Ctrl Pts',(-2.56261070750152,4.48721291871176,66.4839943727018));
#59183=CARTESIAN_POINT('Ctrl Pts',(-5.15976414252148,0.280869025711643,
66.6427551349478));
#59184=CARTESIAN_POINT('Ctrl Pts',(-3.03454382725794,-4.18253477887576,
66.8015158971936));
#59185=CARTESIAN_POINT('Ctrl Pts',(1.86798369006022,-4.81795499664787,66.9602766594396));
#59186=CARTESIAN_POINT('Ctrl Pts',(5.06087547593053,-1.04383563513614,67.1190374216854));
#59187=CARTESIAN_POINT('Ctrl Pts',(3.62189943977487,3.68563398402679,67.2777981839313));
#59188=CARTESIAN_POINT('Ctrl Pts',(-1.13194959602156,5.04189880185246,67.4365589461772));
#59189=CARTESIAN_POINT('Ctrl Pts',(-4.84980378568845,1.78366382941869,67.5953197084231));
#59190=CARTESIAN_POINT('Ctrl Pts',(-4.12896941150786,-3.10703476242022,
67.754080470669));
#59191=CARTESIAN_POINT('Ctrl Pts',(0.370823889097725,-5.15408023407956,
67.9128412329148));
#59192=CARTESIAN_POINT('Ctrl Pts',(4.53122783943781,-2.48395404207855,68.0716019951608));
#59193=CARTESIAN_POINT('Ctrl Pts',(4.5445136629679,2.45956276259679,68.2303627574067));
#59194=CARTESIAN_POINT('Ctrl Pts',(0.398521768172548,5.15201259862078,68.3891235196525));
#59195=CARTESIAN_POINT('Ctrl Pts',(-4.11220942186021,3.12918313411324,68.5478842818985));
#59196=CARTESIAN_POINT('Ctrl Pts',(-4.85932093993431,-1.75757031687816,
68.7066450441443));
#59197=CARTESIAN_POINT('Ctrl Pts',(-1.15903350388962,-5.03574172817834,
68.8654058063903));
#59198=CARTESIAN_POINT('Ctrl Pts',(3.60203679805415,-3.70504849111566,69.0241665686361));
#59199=CARTESIAN_POINT('Ctrl Pts',(5.06641299677213,1.01661829719571,69.182927330882));
#59200=CARTESIAN_POINT('Ctrl Pts',(1.89385326524434,4.80784496690336,69.3416880931279));
#59201=CARTESIAN_POINT('Ctrl Pts',(-3.01201882313635,4.19878506536444,69.5004488553738));
#59202=CARTESIAN_POINT('Ctrl Pts',(-5.16119928126974,-0.25313118155592,
69.6592096176196));
#59203=CARTESIAN_POINT('Ctrl Pts',(-2.58669250630018,-4.47337403912361,
69.8179703798655));
#59204=CARTESIAN_POINT('Ctrl Pts',(2.35523426198658,-4.5994483350962,69.9767311421114));
#59205=CARTESIAN_POINT('Ctrl Pts',(5.14157869213602,-0.51596702281012,70.1354919043573));
#59206=CARTESIAN_POINT('Ctrl Pts',(3.22219325167658,4.03974306916968,70.2942526666032));
#59207=CARTESIAN_POINT('Ctrl Pts',(-1.6462418758917,4.89815690868675,70.4530134288491));
#59208=CARTESIAN_POINT('Ctrl Pts',(-5.00798615353109,1.2736279292227,70.611774191095));
#59209=CARTESIAN_POINT('Ctrl Pts',(-3.78626853252985,-3.51656423453759,
70.7705349533408));
#59210=CARTESIAN_POINT('Ctrl Pts',(0.900757702520816,-5.08828939599587,
70.9292957155868));
#59211=CARTESIAN_POINT('Ctrl Pts',(4.76338297422217,-2.00305667841551,71.0880564778326));
#59212=CARTESIAN_POINT('Ctrl Pts',(4.26641464848803,2.9154346954137,71.2468172400786));
#59213=CARTESIAN_POINT('Ctrl Pts',(-0.135306682874774,5.16563118288797,
71.4055780023244));
#59214=CARTESIAN_POINT('Ctrl Pts',(-4.41319120507407,2.6880842255241,71.5643387645703));
#59215=CARTESIAN_POINT('Ctrl Pts',(-4.65198833370899,-2.24967952364111,
71.7230995268162));
#59216=CARTESIAN_POINT('Ctrl Pts',(-0.63314364249968,-5.12846785541421,
71.8818602890621));
#59217=CARTESIAN_POINT('Ctrl Pts',(3.9651734499498,-3.31352575482195,72.040621051308));
#59218=CARTESIAN_POINT('Ctrl Pts',(4.93444268320512,1.53405632954553,72.1993818135539));
#59219=CARTESIAN_POINT('Ctrl Pts',(1.38755924827672,4.97762320275213,72.3581425757998));
#59220=CARTESIAN_POINT('Ctrl Pts',(-3.42926079422353,3.86551727731956,72.5169033380456));
#59221=CARTESIAN_POINT('Ctrl Pts',(-5.10751660971561,-0.784428134078424,
72.6756641002916));
#59222=CARTESIAN_POINT('Ctrl Pts',(-2.1112172128698,-4.71644095649861,72.8344248625374));
#59223=CARTESIAN_POINT('Ctrl Pts',(2.81733266516402,-4.33182294996633,72.9931856247833));
#59224=CARTESIAN_POINT('Ctrl Pts',(5.16737363149282,0.0174117376300544,
73.1519463870293));
#59225=CARTESIAN_POINT('Ctrl Pts',(2.78807641079671,4.35071067109887,73.3107071492751));
#59226=CARTESIAN_POINT('Ctrl Pts',(-2.14295350396336,4.70210630419026,73.469467911521));
#59227=CARTESIAN_POINT('Ctrl Pts',(-5.11268691452911,0.749990619979619,
73.6282286737669));
#59228=CARTESIAN_POINT('Ctrl Pts',(-3.40313309186266,-3.88853938839824,
73.7869894360128));
#59229=CARTESIAN_POINT('Ctrl Pts',(1.42107208653042,-4.9681593715318,73.9457501982587));
#59230=CARTESIAN_POINT('Ctrl Pts',(4.94466868411869,-1.50076814343543,74.1045109605046));
#59231=CARTESIAN_POINT('Ctrl Pts',(3.94275346512999,3.34017193109278,74.2632717227505));
#59232=CARTESIAN_POINT('Ctrl Pts',(-0.667690158118302,5.12408462740484,
74.4220324849963));
#59233=CARTESIAN_POINT('Ctrl Pts',(-4.6670433537954,2.21827855551313,74.5807932472423));
#59234=CARTESIAN_POINT('Ctrl Pts',(-4.39497591538344,-2.71776380858505,
74.7395540094881));
#59235=CARTESIAN_POINT('Ctrl Pts',(-0.100492272925181,-5.16642571988962,
74.898314771734));
#59236=CARTESIAN_POINT('Ctrl Pts',(4.28596496729055,-2.88661700182285,75.0570755339799));
#59237=CARTESIAN_POINT('Ctrl Pts',(4.74977615293751,2.03511176917654,75.2158362962258));
#59238=CARTESIAN_POINT('Ctrl Pts',(0.866447119614458,5.09424408572719,75.3745970584717));
#59239=CARTESIAN_POINT('Ctrl Pts',(-3.8098807835517,3.4909686093087,75.5333578207175));
#59240=CARTESIAN_POINT('Ctrl Pts',(-4.99928941928749,-1.30734797137385,
75.6921185829635));
#59241=CARTESIAN_POINT('Ctrl Pts',(-1.61319567320764,-4.90913975519121,
75.8508793452094));
#59242=CARTESIAN_POINT('Ctrl Pts',(3.24934402869518,-4.01793688343129,76.0096401074552));
#59243=CARTESIAN_POINT('Ctrl Pts',(5.13798482303055,0.550604553524979,76.1684008697012));
#59244=CARTESIAN_POINT('Ctrl Pts',(2.32418496553848,4.61521588466023,76.3271616319469));
#59245=CARTESIAN_POINT('Ctrl Pts',(-2.61677996556865,4.45584066454958,76.485922394193));
#59246=CARTESIAN_POINT('Ctrl Pts',(-5.16278794160245,0.218343962817818,
76.6446831564387));
#59247=CARTESIAN_POINT('Ctrl Pts',(-2.98365469407069,-4.21898780308791,
76.8034439186847));
#59248=CARTESIAN_POINT('Ctrl Pts',(1.92621046639379,-4.79497306094723,76.9622046809306));
#59249=CARTESIAN_POINT('Ctrl Pts',(5.07314897115,-0.982452509068445,77.1209654431764));
#59250=CARTESIAN_POINT('Ctrl Pts',(3.5769865761566,3.7292385885125,77.2797262054224));
#59251=CARTESIAN_POINT('Ctrl Pts',(-1.19294319381297,5.02781661881079,77.4384869676682));
#59252=CARTESIAN_POINT('Ctrl Pts',(-4.87105491388051,1.72478330291522,77.5972477299142));
#59253=CARTESIAN_POINT('Ctrl Pts',(-4.09102838845504,-3.1568243760003,77.75600849216));
#59254=CARTESIAN_POINT('Ctrl Pts',(0.433232280173729,-5.14920995954434,
77.9147692544059));
#59255=CARTESIAN_POINT('Ctrl Pts',(4.56098553273524,-2.42888130344712,78.0735300166518));
#59256=CARTESIAN_POINT('Ctrl Pts',(4.51438550862023,2.51443371271033,78.2322907788977));
#59257=CARTESIAN_POINT('Ctrl Pts',(0.336081973315249,5.15646219061744,78.3910515411436));
#59258=CARTESIAN_POINT('Ctrl Pts',(-4.1498140497254,3.0791389654831,78.5498123033895));
#59259=CARTESIAN_POINT('Ctrl Pts',(-4.8376734967368,-1.81630629438564,78.7085730656354));
#59260=CARTESIAN_POINT('Ctrl Pts',(-1.0979463908737,-5.04941255383462,78.8673338278812));
#59261=CARTESIAN_POINT('Ctrl Pts',(3.64665478912629,-3.66114220769932,79.0260945901272));
#59262=CARTESIAN_POINT('Ctrl Pts',(5.05372611759689,1.07791731796727,79.184855352373));
#59263=CARTESIAN_POINT('Ctrl Pts',(1.83547293516864,4.83043398881696,79.3436161146189));
#59264=CARTESIAN_POINT('Ctrl Pts',(-3.06266114277673,4.16198992557408,79.5023768768648));
#59265=CARTESIAN_POINT('Ctrl Pts',(-5.15775419265022,-0.315634447191765,
79.6611376391107));
#59266=CARTESIAN_POINT('Ctrl Pts',(-2.53231305975701,-4.50438053270811,
79.8198984013567));
#59267=CARTESIAN_POINT('Ctrl Pts',(2.41077833593552,-4.57057996659486,79.9786591636024));
#59268=CARTESIAN_POINT('Ctrl Pts',(5.14745176039643,-0.453645004871452,
80.1374199258484));
#59269=CARTESIAN_POINT('Ctrl Pts',(3.1730201027819,4.07847972207792,80.2961806880942));
#59270=CARTESIAN_POINT('Ctrl Pts',(-1.70545647406065,4.87785522859546,80.4549414503402));
#59271=CARTESIAN_POINT('Ctrl Pts',(-5.02304719199465,1.21286863387634,80.613702212586));
#59272=CARTESIAN_POINT('Ctrl Pts',(-3.74339168884474,-3.56217238212488,
80.7724629748319));
#59273=CARTESIAN_POINT('Ctrl Pts',(0.962330231331446,-5.07700442602626,
80.9312237370778));
#59274=CARTESIAN_POINT('Ctrl Pts',(4.78729812901886,-1.94520694012218,81.0899844993237));
#59275=CARTESIAN_POINT('Ctrl Pts',(4.2307845491307,2.96690335452649,81.2487452615696));
#59276=CARTESIAN_POINT('Ctrl Pts',(-0.19787228117179,5.16361307382143,81.4075060238155));
#59277=CARTESIAN_POINT('Ctrl Pts',(-4.44543035555655,2.63442638343223,81.5662667860614));
#59278=CARTESIAN_POINT('Ctrl Pts',(-4.62439478129263,-2.30586780285272,
81.7250275483072));
#59279=CARTESIAN_POINT('Ctrl Pts',(-0.57097184883837,-5.13576134197884,
81.8837883105532));
#59280=CARTESIAN_POINT('Ctrl Pts',(4.00502195951943,-3.26524922770216,82.0425490727989));
#59281=CARTESIAN_POINT('Ctrl Pts',(4.91549733690694,1.59371871934676,82.2013098350451));
#59282=CARTESIAN_POINT('Ctrl Pts',(1.32715940311121,4.99406661129702,82.3600705972907));
#59283=CARTESIAN_POINT('Ctrl Pts',(-3.47583534999669,3.82369219939626,82.5188313595369));
#59284=CARTESIAN_POINT('Ctrl Pts',(-5.09763942964231,-0.846242118322492,
82.6775921217824));
#59285=CARTESIAN_POINT('Ctrl Pts',(-2.05392817541576,-4.74166978382725,
82.8363528840287));
#59286=CARTESIAN_POINT('Ctrl Pts',(2.86960084768762,-4.29737645901297,82.9951136462743));
#59287=CARTESIAN_POINT('Ctrl Pts',(5.16678358952832,0.0800071275065655,
83.1538744085204));
#59288=CARTESIAN_POINT('Ctrl Pts',(2.73516803922529,4.38416562959496,83.312635170766));
#59289=CARTESIAN_POINT('Ctrl Pts',(-2.19975659925683,4.67580205641259,83.4713959330121));
#59290=CARTESIAN_POINT('Ctrl Pts',(-5.1213972808606,0.688001186004659,83.6301566952579));
#59291=CARTESIAN_POINT('Ctrl Pts',(-3.35577782577649,-3.92947855970427,
83.7889174575038));
#59292=CARTESIAN_POINT('Ctrl Pts',(1.4811502559097,-4.9505810809301,83.9476782197498));
#59293=CARTESIAN_POINT('Ctrl Pts',(4.96248771955931,-1.44075755171813,84.1064389819956));
#59294=CARTESIAN_POINT('Ctrl Pts',(3.90199844707087,3.38768549854763,84.2651997442416));
#59295=CARTESIAN_POINT('Ctrl Pts',(-0.729706746127024,5.11562640844579,
84.4239605064874));
#59296=CARTESIAN_POINT('Ctrl Pts',(-4.69358549045032,2.16156849958318,84.5827212687333));
#59297=CARTESIAN_POINT('Ctrl Pts',(-4.36170650562841,-2.77078218706868,
84.7414820309791));
#59298=CARTESIAN_POINT('Ctrl Pts',(-0.0379465312430282,-5.16730640666113,
84.9002427932251));
#59299=CARTESIAN_POINT('Ctrl Pts',(4.32070804489202,-2.83440452778566,85.059003555471));
#59300=CARTESIAN_POINT('Ctrl Pts',(4.72460304963626,2.09234474027741,85.2177643177169));
#59301=CARTESIAN_POINT('Ctrl Pts',(0.805001482004623,5.10466438453535,85.3765250799626));
#59302=CARTESIAN_POINT('Ctrl Pts',(-3.85251988452798,3.44398909312549,85.5352858422087));
#59303=CARTESIAN_POINT('Ctrl Pts',(-4.98187820443228,-1.36671670879964,
85.6940466044544));
#59304=CARTESIAN_POINT('Ctrl Pts',(-1.55593411210757,-4.93043766489916,
85.8528073667005));
#59305=CARTESIAN_POINT('Ctrl Pts',(3.302346542614,-3.9740701687742,86.0115681289462));
#59306=CARTESIAN_POINT('Ctrl Pts',(4.81804045098618,-0.159581013320771,
86.1438687641512));
#59307=CARTESIAN_POINT('Ctrl Pts',(3.70615495334781,2.63929363226931,86.2497092723151));
#59308=CARTESIAN_POINT('Ctrl Pts',(2.57208606313468,3.6093054188893,86.3026295263971));
#59309=CARTESIAN_POINT('Ctrl Pts',(1.91898364244101,3.92834389788417,86.329089653438));
#59310=CARTESIAN_POINT('',(2.16917135428672,4.4405021828327,86.));
#59311=CARTESIAN_POINT('Ctrl Pts',(2.54472701347473,-3.56250531650751,85.9999999999999));
#59312=CARTESIAN_POINT('Ctrl Pts',(2.63513329971733,-3.50700228194743,85.9999999999999));
#59313=CARTESIAN_POINT('Ctrl Pts',(2.72315806304114,-3.44815476600379,86.));
#59314=CARTESIAN_POINT('Ctrl Pts',(2.80858471961567,-3.38601400582831,86.));
#59315=CARTESIAN_POINT('Ctrl Pts',(2.91292188753961,-3.31011742753144,86.));
#59316=CARTESIAN_POINT('Ctrl Pts',(3.01338478767473,-3.22930990203852,85.9999999999999));
#59317=CARTESIAN_POINT('Ctrl Pts',(3.1098984160813,-3.14401909712343,85.9999999999999));
#59318=CARTESIAN_POINT('Ctrl Pts',(3.20859981088314,-3.05679492424881,85.9999999999999));
#59319=CARTESIAN_POINT('Ctrl Pts',(3.30317129552995,-2.96488147836652,85.9999999999999));
#59320=CARTESIAN_POINT('Ctrl Pts',(3.39350543356314,-2.86868861821106,85.9999999999999));
#59321=CARTESIAN_POINT('Ctrl Pts',(3.48531110601377,-2.77092878561846,85.9999999999999));
#59322=CARTESIAN_POINT('Ctrl Pts',(3.57274072745551,-2.66874842101355,86.));
#59323=CARTESIAN_POINT('Ctrl Pts',(3.65564683072142,-2.56253686518592,86.));
#59324=CARTESIAN_POINT('Ctrl Pts',(3.68584784338838,-2.52384614862143,86.));
#59325=CARTESIAN_POINT('Ctrl Pts',(3.71544822227817,-2.48462014936941,86.));
#59326=CARTESIAN_POINT('Ctrl Pts',(3.74443952828415,-2.44487660282335,86.));
#59327=CARTESIAN_POINT('Ctrl Pts',(3.75595083040377,-2.42909601082439,86.));
#59328=CARTESIAN_POINT('Ctrl Pts',(3.76736609971463,-2.41323381819194,86.));
#59329=CARTESIAN_POINT('Ctrl Pts',(3.77868477502221,-2.39729111372332,86.));
#59330=CARTESIAN_POINT('Ctrl Pts',(3.78947724093788,-2.38208959146869,86.));
#59331=CARTESIAN_POINT('Ctrl Pts',(3.80017685936615,-2.36682191965604,86.));
#59332=CARTESIAN_POINT('Ctrl Pts',(3.81078105898287,-2.35149266837476,86.));
#59333=CARTESIAN_POINT('Ctrl Pts',(3.88827217096444,-2.23947282995537,86.));
#59334=CARTESIAN_POINT('Ctrl Pts',(3.96071122105411,-2.12411080348259,86.));
#59335=CARTESIAN_POINT('Ctrl Pts',(4.02800505520053,-2.00585829504273,86.));
#59336=CARTESIAN_POINT('Ctrl Pts',(4.09627718657597,-1.88588666771479,86.));
#59337=CARTESIAN_POINT('Ctrl Pts',(4.15925387587574,-1.76293927819734,86.));
#59338=CARTESIAN_POINT('Ctrl Pts',(4.21680206540741,-1.63744665973299,86.));
#59339=CARTESIAN_POINT('Ctrl Pts',(4.27457311504665,-1.5114680607595,86.));
#59340=CARTESIAN_POINT('Ctrl Pts',(4.32687396830893,-1.38292375176368,86.));
#59341=CARTESIAN_POINT('Ctrl Pts',(4.37352758038542,-1.25221847894515,86.));
#59342=CARTESIAN_POINT('Ctrl Pts',(4.41978765417706,-1.1226157473147,86.));
#59343=CARTESIAN_POINT('Ctrl Pts',(4.46049570285582,-0.990887588742712,
86.));
#59344=CARTESIAN_POINT('Ctrl Pts',(4.49543183958698,-0.857409609773572,
86.));
#59345=CARTESIAN_POINT('Ctrl Pts',(4.5001149290464,-0.839517267492425,86.));
#59346=CARTESIAN_POINT('Ctrl Pts',(4.50469423047283,-0.821593465132248,
86.));
#59347=CARTESIAN_POINT('Ctrl Pts',(4.50916914362169,-0.803639092756939,
86.));
#59348=CARTESIAN_POINT('Ctrl Pts',(4.51380380131252,-0.785043788838134,
86.));
#59349=CARTESIAN_POINT('Ctrl Pts',(4.5183245524103,-0.76642335069997,86.));
#59350=CARTESIAN_POINT('Ctrl Pts',(4.52272974339821,-0.747784414927894,
86.));
#59351=CARTESIAN_POINT('Ctrl Pts',(4.55525927718291,-0.610147728443155,
86.));
#59352=CARTESIAN_POINT('Ctrl Pts',(4.58151477805167,-0.471409643850918,
86.));
#59353=CARTESIAN_POINT('Ctrl Pts',(4.60136007125311,-0.332008493005429,
86.));
#59354=CARTESIAN_POINT('Ctrl Pts',(4.6211606972018,-0.19292110252501,86.));
#59355=CARTESIAN_POINT('Ctrl Pts',(4.63458031267456,-0.0531728409362625,
86.));
#59356=CARTESIAN_POINT('Ctrl Pts',(4.64143733545588,0.0868237683291349,
86.));
#59357=CARTESIAN_POINT('Ctrl Pts',(4.64817665416128,0.224417268832664,86.));
#59358=CARTESIAN_POINT('Ctrl Pts',(4.64857698604029,0.362251427033831,86.));
#59359=CARTESIAN_POINT('Ctrl Pts',(4.64241679650986,0.499945184924937,86.));
#59360=CARTESIAN_POINT('Ctrl Pts',(4.64160900570028,0.518001082655194,86.));
#59361=CARTESIAN_POINT('Ctrl Pts',(4.64068833141729,0.536054571915867,86.));
#59362=CARTESIAN_POINT('Ctrl Pts',(4.63965420661563,0.554104796667351,86.));
#59363=CARTESIAN_POINT('Ctrl Pts',(4.63402930249198,0.65228519372856,86.));
#59364=CARTESIAN_POINT('Ctrl Pts',(4.62504894974127,0.750369112179832,86.));
#59365=CARTESIAN_POINT('Ctrl Pts',(4.61279339604946,0.848217515281527,86.));
#59366=CARTESIAN_POINT('Ctrl Pts',(4.6078781705278,0.887460700883271,86.));
#59367=CARTESIAN_POINT('Ctrl Pts',(4.60243597814028,0.926665987486628,86.));
#59368=CARTESIAN_POINT('Ctrl Pts',(4.59647140132863,0.965824309598894,86.));
#59369=CARTESIAN_POINT('Ctrl Pts',(4.59357119157143,0.984864612281179,86.));
#59370=CARTESIAN_POINT('Ctrl Pts',(4.59054712512505,1.00389559177027,86.));
#59371=CARTESIAN_POINT('Ctrl Pts',(4.58740263898465,1.02289935437782,86.));
#59372=CARTESIAN_POINT('Ctrl Pts',(4.56506277525981,1.15791075145704,86.));
#59373=CARTESIAN_POINT('Ctrl Pts',(4.53662319345842,1.29172741325957,86.));
#59374=CARTESIAN_POINT('Ctrl Pts',(4.50239447214487,1.42398414516775,86.));
#59375=CARTESIAN_POINT('Ctrl Pts',(4.46711335178721,1.56030725329147,86.));
#59376=CARTESIAN_POINT('Ctrl Pts',(4.42568158764605,1.6949737254632,86.));
#59377=CARTESIAN_POINT('Ctrl Pts',(4.3783840316949,1.82758749733868,86.));
#59378=CARTESIAN_POINT('Ctrl Pts',(4.33065091250152,1.96142250957807,86.));
#59379=CARTESIAN_POINT('Ctrl Pts',(4.27694321392572,2.09316762674784,86.));
#59380=CARTESIAN_POINT('Ctrl Pts',(4.21750086301315,2.22240829814259,86.));
#59381=CARTESIAN_POINT('Ctrl Pts',(4.17317829962387,2.31877524464499,86.));
#59382=CARTESIAN_POINT('Ctrl Pts',(4.12566627444568,2.41374969077583,86.));
#59383=CARTESIAN_POINT('Ctrl Pts',(4.07504671027994,2.5071531160556,86.));
#59384=CARTESIAN_POINT('Ctrl Pts',(4.04973692819707,2.55385482869548,86.));
#59385=CARTESIAN_POINT('Ctrl Pts',(4.02365003622111,2.60016367547768,86.));
#59386=CARTESIAN_POINT('Ctrl Pts',(3.99679497172134,2.64605655812716,86.));
#59387=CARTESIAN_POINT('Ctrl Pts',(3.98389889010003,2.66809479826952,86.));
#59388=CARTESIAN_POINT('Ctrl Pts',(3.97082565386207,2.69003710756834,86.));
#59389=CARTESIAN_POINT('Ctrl Pts',(3.95757618483902,2.71188087703549,86.));
#59390=CARTESIAN_POINT('Ctrl Pts',(3.94694273066632,2.72941174722991,86.));
#59391=CARTESIAN_POINT('Ctrl Pts',(3.93620106712467,2.74687039690698,86.));
#59392=CARTESIAN_POINT('Ctrl Pts',(3.92535253208302,2.76425480853107,86.));
#59393=CARTESIAN_POINT('Ctrl Pts',(3.92156948774113,2.770317009536,86.));
#59394=CARTESIAN_POINT('Ctrl Pts',(3.91777342701665,2.77637021666335,86.));
#59395=CARTESIAN_POINT('Ctrl Pts',(3.91396438452183,2.78241437972366,86.));
#59396=CARTESIAN_POINT('Ctrl Pts',(3.83729807392157,2.90406796671591,86.));
#59397=CARTESIAN_POINT('Ctrl Pts',(3.7553768005218,3.02205919675202,86.));
#59398=CARTESIAN_POINT('Ctrl Pts',(3.66851542581977,3.13614597147405,86.));
#59399=CARTESIAN_POINT('Ctrl Pts',(3.58104093093735,3.25103803973578,86.));
#59400=CARTESIAN_POINT('Ctrl Pts',(3.48855596305165,3.36197093402805,86.));
#59401=CARTESIAN_POINT('Ctrl Pts',(3.39133507740585,3.46867352459105,86.));
#59402=CARTESIAN_POINT('Ctrl Pts',(3.34733743007933,3.51696215020099,86.));
#59403=CARTESIAN_POINT('Ctrl Pts',(3.30236924503015,3.56438401262811,86.));
#59404=CARTESIAN_POINT('Ctrl Pts',(3.25645316546651,3.61091188198635,86.));
#59405=CARTESIAN_POINT('Ctrl Pts',(3.23459379362241,3.63306250998163,86.));
#59406=CARTESIAN_POINT('Ctrl Pts',(3.21251956234251,3.65501049805194,86.));
#59407=CARTESIAN_POINT('Ctrl Pts',(3.19023278769809,3.67675278772905,86.));
#59408=CARTESIAN_POINT('Ctrl Pts',(3.1754125274436,3.69121097634916,86.));
#59409=CARTESIAN_POINT('Ctrl Pts',(3.16050000228347,3.70557647179484,86.));
#59410=CARTESIAN_POINT('Ctrl Pts',(3.14550229693264,3.71984252397241,86.));
#59411=CARTESIAN_POINT('Ctrl Pts',(3.03965115782958,3.82052978500174,86.));
#59412=CARTESIAN_POINT('Ctrl Pts',(2.92947196960907,3.91635255577481,86.));
#59413=CARTESIAN_POINT('Ctrl Pts',(2.81526020000344,4.00704611824462,86.));
#59414=CARTESIAN_POINT('Ctrl Pts',(2.7017209514917,4.09720564351275,86.));
#59415=CARTESIAN_POINT('Ctrl Pts',(2.58419598194515,4.18229672829323,86.));
#59416=CARTESIAN_POINT('Ctrl Pts',(2.46293629783775,4.26202671871549,86.));
#59417=CARTESIAN_POINT('Ctrl Pts',(2.3673022580591,4.32490747856343,86.));
#59418=CARTESIAN_POINT('Ctrl Pts',(2.26934437440973,4.38445308888104,86.));
#59419=CARTESIAN_POINT('Ctrl Pts',(2.16917135428672,4.4405021828327,86.));
#59420=CARTESIAN_POINT('Ctrl Pts',(2.17574200330365,4.44486699004439,26.));
#59421=CARTESIAN_POINT('Ctrl Pts',(2.28006508424018,4.38720334283182,26.));
#59422=CARTESIAN_POINT('Ctrl Pts',(2.38197081280219,4.32562977310065,26.));
#59423=CARTESIAN_POINT('Ctrl Pts',(2.48120802246663,4.26013719370393,26.));
#59424=CARTESIAN_POINT('Ctrl Pts',(2.60168389996394,4.18062794511602,26.));
#59425=CARTESIAN_POINT('Ctrl Pts',(2.71822805906223,4.09534340135309,26.));
#59426=CARTESIAN_POINT('Ctrl Pts',(2.83065917997165,4.00470474933307,26.));
#59427=CARTESIAN_POINT('Ctrl Pts',(2.90083958424456,3.94812737831637,26.));
#59428=CARTESIAN_POINT('Ctrl Pts',(2.96941670994451,3.88946302886519,26.));
#59429=CARTESIAN_POINT('Ctrl Pts',(3.03633883105725,3.82880744415046,26.));
#59430=CARTESIAN_POINT('Ctrl Pts',(3.07291548330716,3.79565580173034,26.));
#59431=CARTESIAN_POINT('Ctrl Pts',(3.10899764098955,3.76190925146565,26.));
#59432=CARTESIAN_POINT('Ctrl Pts',(3.14457605294962,3.72758291425312,26.));
#59433=CARTESIAN_POINT('Ctrl Pts',(3.16870678245731,3.70430139288574,26.));
#59434=CARTESIAN_POINT('Ctrl Pts',(3.19260993644808,3.68074881011364,26.));
#59435=CARTESIAN_POINT('Ctrl Pts',(3.21625888633569,3.65695400262287,26.));
#59436=CARTESIAN_POINT('Ctrl Pts',(3.31788256697706,3.55470354630845,26.));
#59437=CARTESIAN_POINT('Ctrl Pts',(3.41488652713577,3.44791753206169,26.));
#59438=CARTESIAN_POINT('Ctrl Pts',(3.50709206651038,3.33701451625688,26.));
#59439=CARTESIAN_POINT('Ctrl Pts',(3.59746145912339,3.2283199817939,26.));
#59440=CARTESIAN_POINT('Ctrl Pts',(3.6832218206498,3.11566998580718,26.));
#59441=CARTESIAN_POINT('Ctrl Pts',(3.76416544626806,2.99943221817338,26.));
#59442=CARTESIAN_POINT('Ctrl Pts',(3.79957828247605,2.94857819483358,26.));
#59443=CARTESIAN_POINT('Ctrl Pts',(3.83406863332226,2.89703717531663,26.));
#59444=CARTESIAN_POINT('Ctrl Pts',(3.86761651871398,2.84483889381663,26.));
#59445=CARTESIAN_POINT('Ctrl Pts',(3.89532327236222,2.80172902535561,26.));
#59446=CARTESIAN_POINT('Ctrl Pts',(3.92238715315105,2.75817083249342,26.));
#59447=CARTESIAN_POINT('Ctrl Pts',(3.94879604378199,2.71418084548941,26.));
#59448=CARTESIAN_POINT('Ctrl Pts',(3.95941005243527,2.69650081079038,26.));
#59449=CARTESIAN_POINT('Ctrl Pts',(3.96991386666906,2.6787582983834,26.));
#59450=CARTESIAN_POINT('Ctrl Pts',(3.98030512442337,2.6609577203422,26.));
#59451=CARTESIAN_POINT('Ctrl Pts',(4.05292301831336,2.53656079766556,26.));
#59452=CARTESIAN_POINT('Ctrl Pts',(4.12007774857859,2.40928022608588,26.));
#59453=CARTESIAN_POINT('Ctrl Pts',(4.18159035621228,2.27951928558395,26.));
#59454=CARTESIAN_POINT('Ctrl Pts',(4.24297458767659,2.15002915480893,26.));
#59455=CARTESIAN_POINT('Ctrl Pts',(4.29874053362767,2.01806821927191,26.));
#59456=CARTESIAN_POINT('Ctrl Pts',(4.34866300062458,1.88401668144009,26.));
#59457=CARTESIAN_POINT('Ctrl Pts',(4.39830723531613,1.75071225148679,26.));
#59458=CARTESIAN_POINT('Ctrl Pts',(4.44217322437405,1.61533971306916,26.));
#59459=CARTESIAN_POINT('Ctrl Pts',(4.47998827572883,1.47826395773052,26.));
#59460=CARTESIAN_POINT('Ctrl Pts',(4.50834956424491,1.37545714122654,26.));
#59461=CARTESIAN_POINT('Ctrl Pts',(4.53330618455047,1.27169201598405,26.));
#59462=CARTESIAN_POINT('Ctrl Pts',(4.55472254010161,1.16712293514026,26.));
#59463=CARTESIAN_POINT('Ctrl Pts',(4.5633703360405,1.12489856739035,26.));
#59464=CARTESIAN_POINT('Ctrl Pts',(4.57144068485198,1.0825431363053,26.));
#59465=CARTESIAN_POINT('Ctrl Pts',(4.57892379357549,1.04006693008015,26.));
#59466=CARTESIAN_POINT('Ctrl Pts',(4.58238261217842,1.02043371376567,26.));
#59467=CARTESIAN_POINT('Ctrl Pts',(4.58571635833316,1.00077225530923,26.));
#59468=CARTESIAN_POINT('Ctrl Pts',(4.58892275403614,0.98109144089082,26.));
#59469=CARTESIAN_POINT('Ctrl Pts',(4.6112579051569,0.843998578707096,26.));
#59470=CARTESIAN_POINT('Ctrl Pts',(4.62736483254579,0.706302385469903,26.));
#59471=CARTESIAN_POINT('Ctrl Pts',(4.63704039371253,0.568349643633761,26.));
#59472=CARTESIAN_POINT('Ctrl Pts',(4.64529719664733,0.450625350021645,26.));
#59473=CARTESIAN_POINT('Ctrl Pts',(4.64886975587046,0.332713782967315,26.));
#59474=CARTESIAN_POINT('Ctrl Pts',(4.64760179618238,0.214828774577272,26.));
#59475=CARTESIAN_POINT('Ctrl Pts',(4.64610810169851,0.0759567044171535,
26.));
#59476=CARTESIAN_POINT('Ctrl Pts',(4.63789790766952,-0.0628793196366818,
26.));
#59477=CARTESIAN_POINT('Ctrl Pts',(4.62316922884463,-0.20123695388626,26.));
#59478=CARTESIAN_POINT('Ctrl Pts',(4.60840903270106,-0.339890654178337,
26.));
#59479=CARTESIAN_POINT('Ctrl Pts',(4.58710205140909,-0.478064733297057,
26.));
#59480=CARTESIAN_POINT('Ctrl Pts',(4.55939920087044,-0.615294818730504,
26.));
#59481=CARTESIAN_POINT('Ctrl Pts',(4.54980593455313,-0.66281645389487,26.));
#59482=CARTESIAN_POINT('Ctrl Pts',(4.53944529005038,-0.710224661945217,
26.));
#59483=CARTESIAN_POINT('Ctrl Pts',(4.52832231101321,-0.757499347947085,
26.));
#59484=CARTESIAN_POINT('Ctrl Pts',(4.52204558440698,-0.784176578789409,
26.));
#59485=CARTESIAN_POINT('Ctrl Pts',(4.51552434543633,-0.81081776400017,26.));
#59486=CARTESIAN_POINT('Ctrl Pts',(4.50876854798769,-0.837384466189193,
26.));
#59487=CARTESIAN_POINT('Ctrl Pts',(4.47488762719443,-0.97061882370914,26.));
#59488=CARTESIAN_POINT('Ctrl Pts',(4.43508456291388,-1.10210853291686,26.));
#59489=CARTESIAN_POINT('Ctrl Pts',(4.38958618794437,-1.2314396670372,26.));
#59490=CARTESIAN_POINT('Ctrl Pts',(4.34401166128567,-1.36098726568698,26.));
#59491=CARTESIAN_POINT('Ctrl Pts',(4.29272234355304,-1.48836984485114,26.));
#59492=CARTESIAN_POINT('Ctrl Pts',(4.23589771868779,-1.61315285151403,26.));
#59493=CARTESIAN_POINT('Ctrl Pts',(4.18015009153959,-1.73557084452973,26.));
#59494=CARTESIAN_POINT('Ctrl Pts',(4.11907449353476,-1.85548750502406,26.));
#59495=CARTESIAN_POINT('Ctrl Pts',(4.05280063784894,-1.97246430242313,26.));
#59496=CARTESIAN_POINT('Ctrl Pts',(4.0071971296468,-2.0529568629426,26.));
#59497=CARTESIAN_POINT('Ctrl Pts',(3.95913143391569,-2.13205676654158,26.));
#59498=CARTESIAN_POINT('Ctrl Pts',(3.90866288715487,-2.2096607611529,26.));
#59499=CARTESIAN_POINT('Ctrl Pts',(3.88457170018092,-2.24670506823327,26.));
#59500=CARTESIAN_POINT('Ctrl Pts',(3.85993289144,-2.28340838898037,26.));
#59501=CARTESIAN_POINT('Ctrl Pts',(3.83475240364166,-2.31975877789511,26.));
#59502=CARTESIAN_POINT('Ctrl Pts',(3.81911152043036,-2.34233785548306,26.));
#59503=CARTESIAN_POINT('Ctrl Pts',(3.80326163575805,-2.36478075250477,26.));
#59504=CARTESIAN_POINT('Ctrl Pts',(3.78720411571068,-2.38708450953735,26.));
#59505=CARTESIAN_POINT('Ctrl Pts',(3.77570997324099,-2.40304977442168,26.));
#59506=CARTESIAN_POINT('Ctrl Pts',(3.76411377204687,-2.41893767166227,26.));
#59507=CARTESIAN_POINT('Ctrl Pts',(3.75242084457745,-2.43474120045983,26.));
#59508=CARTESIAN_POINT('Ctrl Pts',(3.66959100122522,-2.54668954001269,26.));
#59509=CARTESIAN_POINT('Ctrl Pts',(3.58184107407233,-2.65450498805187,26.));
#59510=CARTESIAN_POINT('Ctrl Pts',(3.48944434360053,-2.75789800803035,26.));
#59511=CARTESIAN_POINT('Ctrl Pts',(3.40008035358429,-2.85789735603679,26.));
#59512=CARTESIAN_POINT('Ctrl Pts',(3.3063688476751,-2.95376016129811,26.));
#59513=CARTESIAN_POINT('Ctrl Pts',(3.20852006341883,-3.04518760514634,26.));
#59514=CARTESIAN_POINT('Ctrl Pts',(3.11161693078311,-3.13573145589637,26.));
#59515=CARTESIAN_POINT('Ctrl Pts',(3.01065557724222,-3.2219256920299,26.));
#59516=CARTESIAN_POINT('Ctrl Pts',(2.90581240538358,-3.30343749134566,26.));
#59517=CARTESIAN_POINT('Ctrl Pts',(2.80309976478498,-3.38329287915244,26.));
#59518=CARTESIAN_POINT('Ctrl Pts',(2.69666097167601,-3.45865450573126,26.));
#59519=CARTESIAN_POINT('Ctrl Pts',(2.58664264704464,-3.52916309203659,26.));
#59520=CARTESIAN_POINT('Ctrl Pts',(2.57062378681069,-3.53942926535911,26.));
#59521=CARTESIAN_POINT('Ctrl Pts',(2.55452901448013,-3.54959246856517,26.));
#59522=CARTESIAN_POINT('Ctrl Pts',(2.53835875722658,-3.55965150255066,26.));
#59523=CARTESIAN_POINT('Ctrl Pts',(2.16917135428672,4.4405021828327,86.));
#59524=CARTESIAN_POINT('Ctrl Pts',(2.90742207776984,4.07986902565238,85.973539872959));
#59525=CARTESIAN_POINT('Ctrl Pts',(3.54838370350565,3.53163043353487,85.947079745918));
#59526=CARTESIAN_POINT('Ctrl Pts',(4.02597047844268,2.86203885652618,85.9206196188771));
#59527=CARTESIAN_POINT('Ctrl Pts',(4.50355725337971,2.19244727951748,85.894159491836));
#59528=CARTESIAN_POINT('Ctrl Pts',(4.817769177518,1.40150271761755,85.8676993647951));
#59529=CARTESIAN_POINT('Ctrl Pts',(4.91302361527573,0.586752768661848,85.8412392377541));
#59530=CARTESIAN_POINT('Ctrl Pts',(5.10353249079119,-1.04274712924955,85.7883189836721));
#59531=CARTESIAN_POINT('Ctrl Pts',(4.41821142078444,-2.76746857538425,85.7353987295902));
#59532=CARTESIAN_POINT('Ctrl Pts',(3.16027096066549,-3.81000496808603,85.6824784755082));
#59533=CARTESIAN_POINT('Ctrl Pts',(1.90233050054647,-4.85254136078787,85.6295582214263));
#59534=CARTESIAN_POINT('Ctrl Pts',(0.071770650315324,-5.21289270005682,
85.5766379673442));
#59535=CARTESIAN_POINT('Ctrl Pts',(-1.4889429323282,-4.72167812247258,85.5237177132623));
#59536=CARTESIAN_POINT('Ctrl Pts',(-3.04965651497173,-4.23046354488835,
85.4707974591803));
#59537=CARTESIAN_POINT('Ctrl Pts',(-4.34052383002751,-2.88768305045078,
85.4178772050984));
#59538=CARTESIAN_POINT('Ctrl Pts',(-4.77319106421879,-1.30997578306141,
85.3649569510165));
#59539=CARTESIAN_POINT('Ctrl Pts',(-4.88938737554012,-0.886269640491669,
85.3507447855632));
#59540=CARTESIAN_POINT('Ctrl Pts',(-4.94368731125384,-0.445619761719663,
85.33653262011));
#59541=CARTESIAN_POINT('Ctrl Pts',(-4.93983901057914,-0.00407131671605609,
85.3223204546568));
#59542=CARTESIAN_POINT('Origin',(0.,0.,16.));
#59543=CARTESIAN_POINT('Origin',(0.,0.,86.));
#59544=CARTESIAN_POINT('Origin',(0.,0.,26.));
#59545=CARTESIAN_POINT('',(4.61880215351701,-8.,26.));
#59546=CARTESIAN_POINT('',(9.23760430703401,0.,26.));
#59547=CARTESIAN_POINT('',(4.61880215351701,-8.,26.));
#59548=CARTESIAN_POINT('',(4.61880215351701,8.,26.));
#59549=CARTESIAN_POINT('',(9.23760430703401,0.,26.));
#59550=CARTESIAN_POINT('',(-4.61880215351701,8.,26.));
#59551=CARTESIAN_POINT('',(4.61880215351701,8.,26.));
#59552=CARTESIAN_POINT('',(-9.23760430703401,1.11022302462516E-15,26.));
#59553=CARTESIAN_POINT('',(-4.618802153517,8.,26.));
#59554=CARTESIAN_POINT('',(-4.61880215351701,-8.,26.));
#59555=CARTESIAN_POINT('',(-9.23760430703401,1.1312802546399E-15,26.));
#59556=CARTESIAN_POINT('',(-4.61880215351701,-8.,26.));
#59557=CARTESIAN_POINT('Origin',(0.,0.,20.));
#59558=CARTESIAN_POINT('',(4.61880215351701,-8.,20.));
#59559=CARTESIAN_POINT('',(9.23760430703401,0.,20.));
#59560=CARTESIAN_POINT('',(4.61880215351701,-8.,20.));
#59561=CARTESIAN_POINT('',(-4.61880215351701,-8.,20.));
#59562=CARTESIAN_POINT('',(-4.61880215351701,-8.,20.));
#59563=CARTESIAN_POINT('',(-9.23760430703401,1.1312802546399E-15,20.));
#59564=CARTESIAN_POINT('',(-9.23760430703401,1.1312802546399E-15,20.));
#59565=CARTESIAN_POINT('',(-4.618802153517,8.,20.));
#59566=CARTESIAN_POINT('',(-4.618802153517,8.,20.));
#59567=CARTESIAN_POINT('',(4.61880215351701,8.,20.));
#59568=CARTESIAN_POINT('',(4.61880215351701,8.,20.));
#59569=CARTESIAN_POINT('',(9.23760430703401,0.,20.));
#59570=CARTESIAN_POINT('',(-5.,6.12323399573677E-16,20.));
#59571=CARTESIAN_POINT('Origin',(0.,0.,20.));
#59572=CARTESIAN_POINT('Origin',(-4.61880215351701,-8.,20.));
#59573=CARTESIAN_POINT('',(4.61880215351701,-8.,20.));
#59574=CARTESIAN_POINT('',(-4.61880215351701,-8.,20.));
#59575=CARTESIAN_POINT('Origin',(-9.23760430703401,1.1312802546399E-15,
20.));
#59576=CARTESIAN_POINT('',(-9.23760430703401,1.1312802546399E-15,20.));
#59577=CARTESIAN_POINT('Origin',(-4.618802153517,8.,20.));
#59578=CARTESIAN_POINT('',(-4.618802153517,8.,20.));
#59579=CARTESIAN_POINT('Origin',(4.61880215351701,8.,20.));
#59580=CARTESIAN_POINT('',(4.61880215351701,8.,20.));
#59581=CARTESIAN_POINT('Origin',(9.23760430703401,0.,20.));
#59582=CARTESIAN_POINT('',(9.23760430703401,0.,20.));
#59583=CARTESIAN_POINT('Origin',(4.61880215351701,-8.,20.));
#59584=CARTESIAN_POINT('Origin',(0.,0.,16.));
#59585=CARTESIAN_POINT('',(-5.,6.12323399573677E-16,17.3166247903554));
#59586=CARTESIAN_POINT('',(-5.,-6.12323399573677E-16,16.));
#59587=CARTESIAN_POINT('Origin',(0.,0.,17.3166247903554));
#59588=CARTESIAN_POINT('Origin',(0.,0.,86.));
#59589=CARTESIAN_POINT('Origin',(5.55111512312578E-16,0.,14.));
#59590=CARTESIAN_POINT('',(1.87717472568372E-16,-4.49927934798557E-32,8.));
#59591=CARTESIAN_POINT('Origin',(5.55111512312578E-16,0.,14.));
#63730=UNCERTAINTY_MEASURE_WITH_UNIT(LENGTH_MEASURE(0.01),#63756,
'DISTANCE_ACCURACY_VALUE',
'Maximum model space distance between geometric entities at asserted c
onnectivities');
#63735=UNCERTAINTY_MEASURE_WITH_UNIT(LENGTH_MEASURE(0.01),#63756,
'DISTANCE_ACCURACY_VALUE',
'Maximum model space distance between geometric entities at asserted c
onnectivities');
#63750=(
GEOMETRIC_REPRESENTATION_CONTEXT(3)
GLOBAL_UNCERTAINTY_ASSIGNED_CONTEXT((#63730))
GLOBAL_UNIT_ASSIGNED_CONTEXT((#63756,#63758,#63759))
REPRESENTATION_CONTEXT('','3D')
);
#63755=(
GEOMETRIC_REPRESENTATION_CONTEXT(3)
GLOBAL_UNCERTAINTY_ASSIGNED_CONTEXT((#63735))
GLOBAL_UNIT_ASSIGNED_CONTEXT((#63756,#63758,#63759))
REPRESENTATION_CONTEXT('','3D')
);
#63756=(
LENGTH_UNIT()
NAMED_UNIT(*)
SI_UNIT(.MILLI.,.METRE.)
);
#63758=(
NAMED_UNIT(*)
PLANE_ANGLE_UNIT()
SI_UNIT($,.RADIAN.)
);
#63759=(
NAMED_UNIT(*)
SI_UNIT($,.STERADIAN.)
SOLID_ANGLE_UNIT()
);
#63774=SHAPE_DEFINITION_REPRESENTATION(#63833,#63872);
#63833=PRODUCT_DEFINITION_SHAPE('',$,#63892);
#63872=SHAPE_REPRESENTATION('',(#15253),#63750);
#63877=PRODUCT_DEFINITION_CONTEXT('part definition',#63936,'design');
#63892=PRODUCT_DEFINITION('Adjusting spindle','Adjusting spindle',#63911,
#63877);
#63911=PRODUCT_DEFINITION_FORMATION('',$,#63952);
#63936=APPLICATION_CONTEXT(
'Core Data for Automotive Mechanical Design Process');
#63937=PRODUCT_CONTEXT('part definition',#63936,'mechanical');
#63952=PRODUCT('Adjusting spindle','Adjusting spindle',$,(#63937));
#63963=PRESENTATION_STYLE_ASSIGNMENT((#63970));
#63970=SURFACE_STYLE_USAGE(.BOTH.,#63977);
#63977=SURFACE_SIDE_STYLE('',(#63984));
#63984=SURFACE_STYLE_FILL_AREA(#63991);
#63991=FILL_AREA_STYLE('Light blue',(#63998));
#63998=FILL_AREA_STYLE_COLOUR('Light blue',#64005);
#64005=COLOUR_RGB('Light blue',0.662745098039216,0.831372549019608,0.949019607843137);
ENDSEC;
END-ISO-10303-21;
